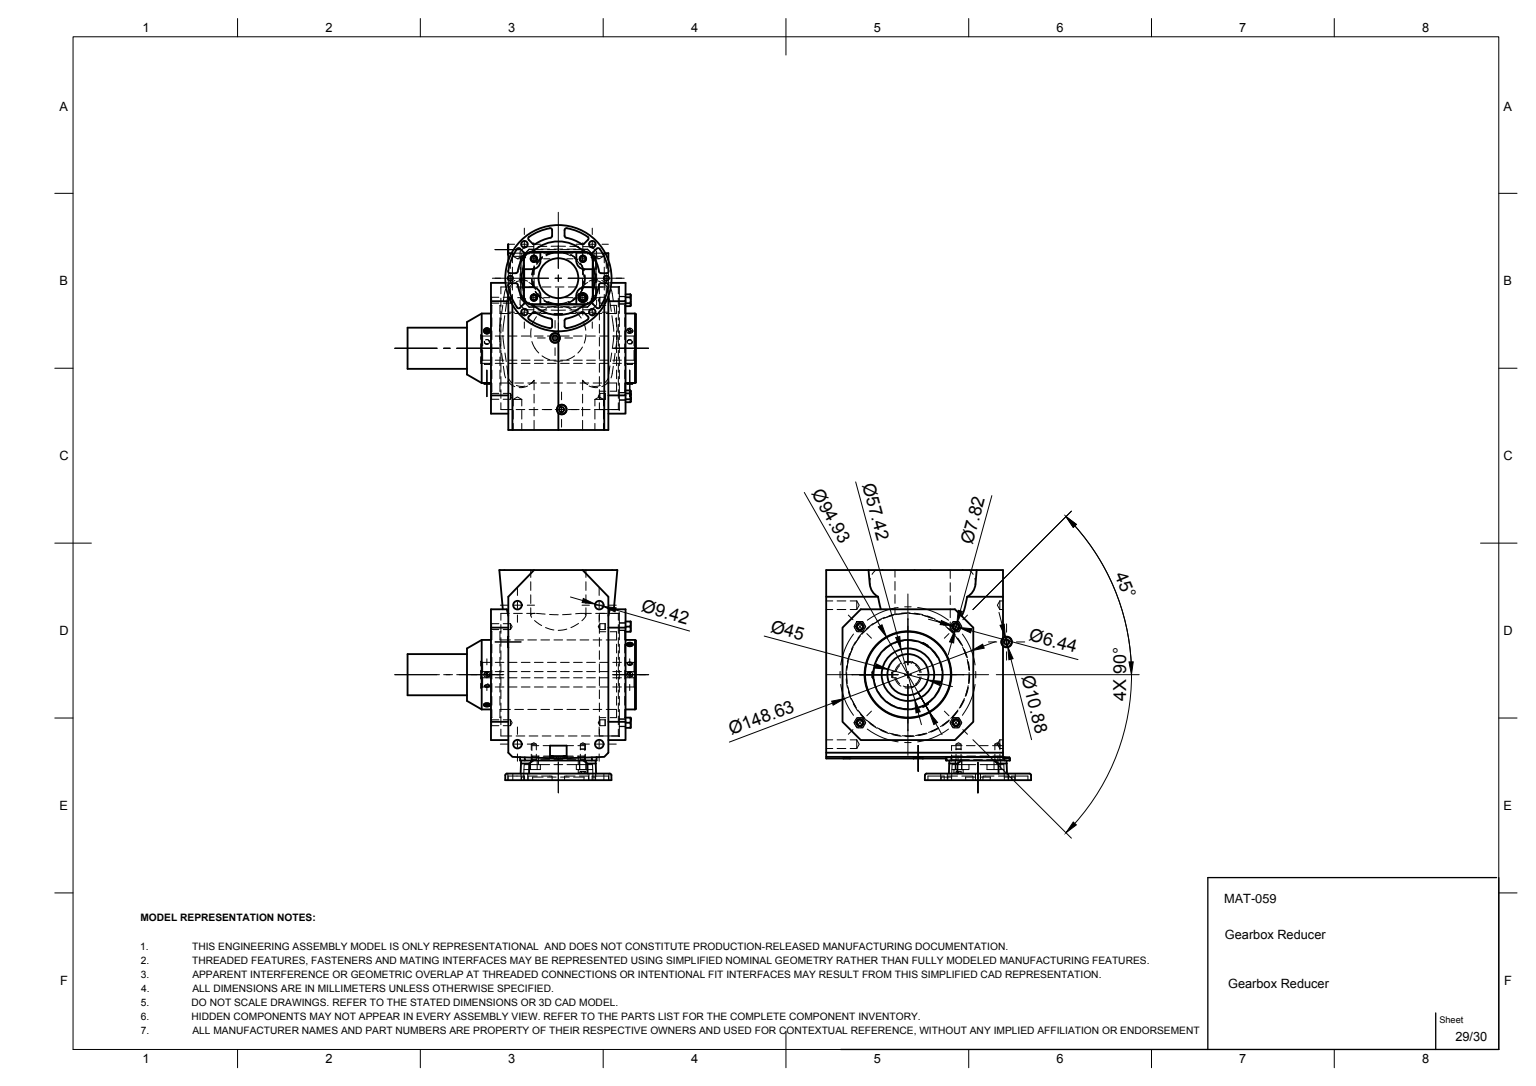
ISO-10303-21;
HEADER;
/* Generated by software containing ST-Developer
 * from STEP Tools, Inc. (www.steptools.com) 
 */

FILE_DESCRIPTION(
/* description */ ('', 'CAx-IF Rec.Pracs.---Representation and Presentation of Product Manufa
cturing Information (PMI)---4.0---2014-10-13'),
/* implementation_level */ '2;1');

FILE_NAME(
/* name */ 'Gearbox Reducer.step',
/* time_stamp */ '2026-10-28T23:00:48+01:00',
/* author */ (''),
/* organization */ (''),
/* preprocessor_version */ 'ST-DEVELOPER v20.2',
/* originating_system */ 'Autodesk Translation Framework v15.17.0.0',
/* authorisation */ '');

FILE_SCHEMA (('AP242_MANAGED_MODEL_BASED_3D_ENGINEERING_MIM_LF { 1 0 10303 442 2 1 4 }'));
ENDSEC;

DATA;
#10=MECHANICAL_DESIGN_GEOMETRIC_PRESENTATION_REPRESENTATION('',(#998),#61811);
#11=ORIENTED_CLOSED_SHELL('',*,#33828,.F.);
#12=ORIENTED_CLOSED_SHELL('',*,#33829,.F.);
#13=ORIENTED_CLOSED_SHELL('',*,#33830,.F.);
#14=ORIENTED_CLOSED_SHELL('',*,#33831,.F.);
#15=ORIENTED_CLOSED_SHELL('',*,#33832,.F.);
#16=ORIENTED_CLOSED_SHELL('',*,#33833,.F.);
#17=ORIENTED_CLOSED_SHELL('',*,#33834,.F.);
#18=ORIENTED_CLOSED_SHELL('',*,#33835,.F.);
#19=ORIENTED_CLOSED_SHELL('',*,#33836,.F.);
#20=ORIENTED_CLOSED_SHELL('',*,#33837,.F.);
#21=BREP_WITH_VOIDS('Body1',#33838,(#11,#12,#13,#14,#15,#16,#17,#18,#19,
#20));
#458=ELLIPSE('',#37359,23.7795204048042,16.4507119775366);
#459=ELLIPSE('',#37368,23.7795204048042,16.4507119775362);
#460=ELLIPSE('',#37370,5.0654611915013,5.05947474242203);
#461=ELLIPSE('',#37371,5.307986116055,5.30171304685244);
#462=ELLIPSE('',#37381,5.06546119150016,5.0594747424216);
#463=ELLIPSE('',#37382,5.30798611605508,5.3017130468524);
#464=ELLIPSE('',#37390,28.8874406483305,28.8698432);
#465=ELLIPSE('',#37391,28.8874406483305,28.8698432);
#466=ELLIPSE('',#37396,28.8695481487031,28.8519616);
#467=ELLIPSE('',#37397,28.8695481487031,28.8519616);
#468=ELLIPSE('',#37482,23.7795204048045,16.4507119775369);
#469=ELLIPSE('',#37484,23.7795204048049,16.4507119775379);
#470=ELLIPSE('',#37887,838.618438479801,28.7580992116283);
#471=ELLIPSE('',#37889,839.102181389802,28.77690685743);
#472=ELLIPSE('',#37898,838.752454381848,28.7633083459289);
#473=ELLIPSE('',#37900,838.930999847209,28.7702505633731);
#511=(
BOUNDED_CURVE()
B_SPLINE_CURVE(2,(#58779,#58780,#58781),.UNSPECIFIED.,.F.,.F.)
B_SPLINE_CURVE_WITH_KNOTS((3,3),(-1.96119676425552,-0.523147579176476),
 .UNSPECIFIED.)
CURVE()
GEOMETRIC_REPRESENTATION_ITEM()
RATIONAL_B_SPLINE_CURVE((1.06676786887492,1.04969648457804,1.02176211535249))
REPRESENTATION_ITEM('')
);
#512=(
BOUNDED_CURVE()
B_SPLINE_CURVE(2,(#58801,#58802,#58803),.UNSPECIFIED.,.F.,.F.)
B_SPLINE_CURVE_WITH_KNOTS((3,3),(-7.9190884120588,-5.23007186679282),
 .UNSPECIFIED.)
CURVE()
GEOMETRIC_REPRESENTATION_ITEM()
RATIONAL_B_SPLINE_CURVE((1.02176211535249,1.07399675503552,1.08824844879795))
REPRESENTATION_ITEM('')
);
#513=(
BOUNDED_CURVE()
B_SPLINE_CURVE(2,(#58988,#58989,#58990),.UNSPECIFIED.,.F.,.F.)
B_SPLINE_CURVE_WITH_KNOTS((3,3),(5.23007186679282,7.9190884120588),
 .UNSPECIFIED.)
CURVE()
GEOMETRIC_REPRESENTATION_ITEM()
RATIONAL_B_SPLINE_CURVE((1.08824844879795,1.07399675503552,1.02176211535249))
REPRESENTATION_ITEM('')
);
#514=(
BOUNDED_CURVE()
B_SPLINE_CURVE(2,(#59004,#59005,#59006),.UNSPECIFIED.,.F.,.F.)
B_SPLINE_CURVE_WITH_KNOTS((3,3),(0.523147579176475,1.96119676425551),
 .UNSPECIFIED.)
CURVE()
GEOMETRIC_REPRESENTATION_ITEM()
RATIONAL_B_SPLINE_CURVE((1.02176211535249,1.04969648457805,1.06676786887492))
REPRESENTATION_ITEM('')
);
#515=(
BOUNDED_CURVE()
B_SPLINE_CURVE(2,(#59072,#59073,#59074),.UNSPECIFIED.,.F.,.F.)
B_SPLINE_CURVE_WITH_KNOTS((3,3),(0.,0.357592968100342),.UNSPECIFIED.)
CURVE()
GEOMETRIC_REPRESENTATION_ITEM()
RATIONAL_B_SPLINE_CURVE((1.,1.00186100329507,1.))
REPRESENTATION_ITEM('')
);
#516=(
BOUNDED_CURVE()
B_SPLINE_CURVE(2,(#59077,#59078,#59079),.UNSPECIFIED.,.F.,.F.)
B_SPLINE_CURVE_WITH_KNOTS((3,3),(0.,0.357592968100342),.UNSPECIFIED.)
CURVE()
GEOMETRIC_REPRESENTATION_ITEM()
RATIONAL_B_SPLINE_CURVE((1.,1.00186100329509,1.))
REPRESENTATION_ITEM('')
);
#517=(
BOUNDED_CURVE()
B_SPLINE_CURVE(2,(#59162,#59163,#59164),.UNSPECIFIED.,.F.,.F.)
B_SPLINE_CURVE_WITH_KNOTS((3,3),(1.4922333840247,2.15631214646323),
 .UNSPECIFIED.)
CURVE()
GEOMETRIC_REPRESENTATION_ITEM()
RATIONAL_B_SPLINE_CURVE((1.8473383335981,1.95114786800464,1.97954092996664))
REPRESENTATION_ITEM('')
);
#518=(
BOUNDED_CURVE()
B_SPLINE_CURVE(2,(#59168,#59169,#59170),.UNSPECIFIED.,.F.,.F.)
B_SPLINE_CURVE_WITH_KNOTS((3,3),(2.65634161849746,3.32042038093599),
 .UNSPECIFIED.)
CURVE()
GEOMETRIC_REPRESENTATION_ITEM()
RATIONAL_B_SPLINE_CURVE((1.97954092996664,1.95114786800464,1.8473383335981))
REPRESENTATION_ITEM('')
);
#519=(
BOUNDED_CURVE()
B_SPLINE_CURVE(2,(#59179,#59180,#59181),.UNSPECIFIED.,.F.,.F.)
B_SPLINE_CURVE_WITH_KNOTS((3,3),(1.4922333840247,2.15631214646323),
 .UNSPECIFIED.)
CURVE()
GEOMETRIC_REPRESENTATION_ITEM()
RATIONAL_B_SPLINE_CURVE((1.8473383335981,1.95114786800464,1.97954092996664))
REPRESENTATION_ITEM('')
);
#520=(
BOUNDED_CURVE()
B_SPLINE_CURVE(2,(#59184,#59185,#59186),.UNSPECIFIED.,.F.,.F.)
B_SPLINE_CURVE_WITH_KNOTS((3,3),(2.65634161849746,3.32042038093599),
 .UNSPECIFIED.)
CURVE()
GEOMETRIC_REPRESENTATION_ITEM()
RATIONAL_B_SPLINE_CURVE((1.97954092996664,1.95114786800464,1.8473383335981))
REPRESENTATION_ITEM('')
);
#521=(
BOUNDED_CURVE()
B_SPLINE_CURVE(2,(#59193,#59194,#59195),.UNSPECIFIED.,.F.,.F.)
B_SPLINE_CURVE_WITH_KNOTS((3,3),(1.4922333840247,2.15631214646323),
 .UNSPECIFIED.)
CURVE()
GEOMETRIC_REPRESENTATION_ITEM()
RATIONAL_B_SPLINE_CURVE((1.8473383335981,1.95114786800464,1.97954092996664))
REPRESENTATION_ITEM('')
);
#522=(
BOUNDED_CURVE()
B_SPLINE_CURVE(2,(#59198,#59199,#59200),.UNSPECIFIED.,.F.,.F.)
B_SPLINE_CURVE_WITH_KNOTS((3,3),(2.65634161849746,3.32042038093599),
 .UNSPECIFIED.)
CURVE()
GEOMETRIC_REPRESENTATION_ITEM()
RATIONAL_B_SPLINE_CURVE((1.97954092996664,1.95114786800464,1.8473383335981))
REPRESENTATION_ITEM('')
);
#523=(
BOUNDED_CURVE()
B_SPLINE_CURVE(2,(#59207,#59208,#59209),.UNSPECIFIED.,.F.,.F.)
B_SPLINE_CURVE_WITH_KNOTS((3,3),(1.4922333840247,2.15631214646323),
 .UNSPECIFIED.)
CURVE()
GEOMETRIC_REPRESENTATION_ITEM()
RATIONAL_B_SPLINE_CURVE((1.8473383335981,1.95114786800464,1.97954092996664))
REPRESENTATION_ITEM('')
);
#524=(
BOUNDED_CURVE()
B_SPLINE_CURVE(2,(#59212,#59213,#59214),.UNSPECIFIED.,.F.,.F.)
B_SPLINE_CURVE_WITH_KNOTS((3,3),(2.65634161849746,3.32042038093599),
 .UNSPECIFIED.)
CURVE()
GEOMETRIC_REPRESENTATION_ITEM()
RATIONAL_B_SPLINE_CURVE((1.97954092996664,1.95114786800464,1.8473383335981))
REPRESENTATION_ITEM('')
);
#525=(
BOUNDED_CURVE()
B_SPLINE_CURVE(2,(#59220,#59221,#59222),.UNSPECIFIED.,.F.,.F.)
B_SPLINE_CURVE_WITH_KNOTS((3,3),(-2.15631214646323,-1.4922333840247),
 .UNSPECIFIED.)
CURVE()
GEOMETRIC_REPRESENTATION_ITEM()
RATIONAL_B_SPLINE_CURVE((1.97954092996664,1.95114786800464,1.8473383335981))
REPRESENTATION_ITEM('')
);
#526=(
BOUNDED_CURVE()
B_SPLINE_CURVE(2,(#59229,#59230,#59231),.UNSPECIFIED.,.F.,.F.)
B_SPLINE_CURVE_WITH_KNOTS((3,3),(-3.32042038093599,-2.65634161849746),
 .UNSPECIFIED.)
CURVE()
GEOMETRIC_REPRESENTATION_ITEM()
RATIONAL_B_SPLINE_CURVE((1.8473383335981,1.95114786800464,1.97954092996664))
REPRESENTATION_ITEM('')
);
#527=(
BOUNDED_CURVE()
B_SPLINE_CURVE(2,(#59233,#59234,#59235),.UNSPECIFIED.,.F.,.F.)
B_SPLINE_CURVE_WITH_KNOTS((3,3),(-2.15631214646323,-1.4922333840247),
 .UNSPECIFIED.)
CURVE()
GEOMETRIC_REPRESENTATION_ITEM()
RATIONAL_B_SPLINE_CURVE((1.97954092996664,1.95114786800464,1.8473383335981))
REPRESENTATION_ITEM('')
);
#528=(
BOUNDED_CURVE()
B_SPLINE_CURVE(2,(#59239,#59240,#59241),.UNSPECIFIED.,.F.,.F.)
B_SPLINE_CURVE_WITH_KNOTS((3,3),(-3.32042038093599,-2.65634161849746),
 .UNSPECIFIED.)
CURVE()
GEOMETRIC_REPRESENTATION_ITEM()
RATIONAL_B_SPLINE_CURVE((1.8473383335981,1.95114786800464,1.97954092996664))
REPRESENTATION_ITEM('')
);
#529=(
BOUNDED_CURVE()
B_SPLINE_CURVE(2,(#59259,#59260,#59261),.UNSPECIFIED.,.F.,.F.)
B_SPLINE_CURVE_WITH_KNOTS((3,3),(1.4922333840247,2.15631214646323),
 .UNSPECIFIED.)
CURVE()
GEOMETRIC_REPRESENTATION_ITEM()
RATIONAL_B_SPLINE_CURVE((1.8473383335981,1.95114786800464,1.97954092996664))
REPRESENTATION_ITEM('')
);
#530=(
BOUNDED_CURVE()
B_SPLINE_CURVE(2,(#59265,#59266,#59267),.UNSPECIFIED.,.F.,.F.)
B_SPLINE_CURVE_WITH_KNOTS((3,3),(2.65634161849746,3.32042038093599),
 .UNSPECIFIED.)
CURVE()
GEOMETRIC_REPRESENTATION_ITEM()
RATIONAL_B_SPLINE_CURVE((1.97954092996664,1.95114786800464,1.8473383335981))
REPRESENTATION_ITEM('')
);
#531=(
BOUNDED_CURVE()
B_SPLINE_CURVE(2,(#59276,#59277,#59278),.UNSPECIFIED.,.F.,.F.)
B_SPLINE_CURVE_WITH_KNOTS((3,3),(1.4922333840247,2.15631214646323),
 .UNSPECIFIED.)
CURVE()
GEOMETRIC_REPRESENTATION_ITEM()
RATIONAL_B_SPLINE_CURVE((1.8473383335981,1.95114786800464,1.97954092996664))
REPRESENTATION_ITEM('')
);
#532=(
BOUNDED_CURVE()
B_SPLINE_CURVE(2,(#59281,#59282,#59283),.UNSPECIFIED.,.F.,.F.)
B_SPLINE_CURVE_WITH_KNOTS((3,3),(2.65634161849746,3.32042038093599),
 .UNSPECIFIED.)
CURVE()
GEOMETRIC_REPRESENTATION_ITEM()
RATIONAL_B_SPLINE_CURVE((1.97954092996664,1.95114786800464,1.8473383335981))
REPRESENTATION_ITEM('')
);
#533=(
BOUNDED_CURVE()
B_SPLINE_CURVE(2,(#59290,#59291,#59292),.UNSPECIFIED.,.F.,.F.)
B_SPLINE_CURVE_WITH_KNOTS((3,3),(1.4922333840247,2.15631214646323),
 .UNSPECIFIED.)
CURVE()
GEOMETRIC_REPRESENTATION_ITEM()
RATIONAL_B_SPLINE_CURVE((1.8473383335981,1.95114786800464,1.97954092996664))
REPRESENTATION_ITEM('')
);
#534=(
BOUNDED_CURVE()
B_SPLINE_CURVE(2,(#59295,#59296,#59297),.UNSPECIFIED.,.F.,.F.)
B_SPLINE_CURVE_WITH_KNOTS((3,3),(2.65634161849746,3.32042038093599),
 .UNSPECIFIED.)
CURVE()
GEOMETRIC_REPRESENTATION_ITEM()
RATIONAL_B_SPLINE_CURVE((1.97954092996664,1.95114786800464,1.8473383335981))
REPRESENTATION_ITEM('')
);
#535=(
BOUNDED_CURVE()
B_SPLINE_CURVE(2,(#59304,#59305,#59306),.UNSPECIFIED.,.F.,.F.)
B_SPLINE_CURVE_WITH_KNOTS((3,3),(1.4922333840247,2.15631214646323),
 .UNSPECIFIED.)
CURVE()
GEOMETRIC_REPRESENTATION_ITEM()
RATIONAL_B_SPLINE_CURVE((1.8473383335981,1.95114786800464,1.97954092996664))
REPRESENTATION_ITEM('')
);
#536=(
BOUNDED_CURVE()
B_SPLINE_CURVE(2,(#59309,#59310,#59311),.UNSPECIFIED.,.F.,.F.)
B_SPLINE_CURVE_WITH_KNOTS((3,3),(2.65634161849746,3.32042038093599),
 .UNSPECIFIED.)
CURVE()
GEOMETRIC_REPRESENTATION_ITEM()
RATIONAL_B_SPLINE_CURVE((1.97954092996664,1.95114786800464,1.8473383335981))
REPRESENTATION_ITEM('')
);
#537=(
BOUNDED_CURVE()
B_SPLINE_CURVE(2,(#59317,#59318,#59319),.UNSPECIFIED.,.F.,.F.)
B_SPLINE_CURVE_WITH_KNOTS((3,3),(-2.15631214646323,-1.4922333840247),
 .UNSPECIFIED.)
CURVE()
GEOMETRIC_REPRESENTATION_ITEM()
RATIONAL_B_SPLINE_CURVE((1.97954092996664,1.95114786800464,1.8473383335981))
REPRESENTATION_ITEM('')
);
#538=(
BOUNDED_CURVE()
B_SPLINE_CURVE(2,(#59326,#59327,#59328),.UNSPECIFIED.,.F.,.F.)
B_SPLINE_CURVE_WITH_KNOTS((3,3),(-3.32042038093599,-2.65634161849746),
 .UNSPECIFIED.)
CURVE()
GEOMETRIC_REPRESENTATION_ITEM()
RATIONAL_B_SPLINE_CURVE((1.8473383335981,1.95114786800464,1.97954092996664))
REPRESENTATION_ITEM('')
);
#539=(
BOUNDED_CURVE()
B_SPLINE_CURVE(2,(#59330,#59331,#59332),.UNSPECIFIED.,.F.,.F.)
B_SPLINE_CURVE_WITH_KNOTS((3,3),(-2.15631214646323,-1.4922333840247),
 .UNSPECIFIED.)
CURVE()
GEOMETRIC_REPRESENTATION_ITEM()
RATIONAL_B_SPLINE_CURVE((1.97954092996664,1.95114786800464,1.8473383335981))
REPRESENTATION_ITEM('')
);
#540=(
BOUNDED_CURVE()
B_SPLINE_CURVE(2,(#59336,#59337,#59338),.UNSPECIFIED.,.F.,.F.)
B_SPLINE_CURVE_WITH_KNOTS((3,3),(-3.32042038093599,-2.65634161849746),
 .UNSPECIFIED.)
CURVE()
GEOMETRIC_REPRESENTATION_ITEM()
RATIONAL_B_SPLINE_CURVE((1.8473383335981,1.95114786800464,1.97954092996664))
REPRESENTATION_ITEM('')
);
#541=(
BOUNDED_CURVE()
B_SPLINE_CURVE(2,(#60436,#60437,#60438),.UNSPECIFIED.,.F.,.F.)
B_SPLINE_CURVE_WITH_KNOTS((3,3),(1.4922333840247,2.15631214646323),
 .UNSPECIFIED.)
CURVE()
GEOMETRIC_REPRESENTATION_ITEM()
RATIONAL_B_SPLINE_CURVE((1.8473383335981,1.95114786800464,1.97954092996664))
REPRESENTATION_ITEM('')
);
#542=(
BOUNDED_CURVE()
B_SPLINE_CURVE(2,(#60439,#60440,#60441),.UNSPECIFIED.,.F.,.F.)
B_SPLINE_CURVE_WITH_KNOTS((3,3),(2.65634161849746,3.32042038093599),
 .UNSPECIFIED.)
CURVE()
GEOMETRIC_REPRESENTATION_ITEM()
RATIONAL_B_SPLINE_CURVE((1.97954092996664,1.95114786800464,1.8473383335981))
REPRESENTATION_ITEM('')
);
#543=(
BOUNDED_CURVE()
B_SPLINE_CURVE(2,(#60444,#60445,#60446),.UNSPECIFIED.,.F.,.F.)
B_SPLINE_CURVE_WITH_KNOTS((3,3),(-3.32042038093599,-2.65634161849746),
 .UNSPECIFIED.)
CURVE()
GEOMETRIC_REPRESENTATION_ITEM()
RATIONAL_B_SPLINE_CURVE((1.8473383335981,1.95114786800464,1.97954092996664))
REPRESENTATION_ITEM('')
);
#544=(
BOUNDED_CURVE()
B_SPLINE_CURVE(2,(#60448,#60449,#60450),.UNSPECIFIED.,.F.,.F.)
B_SPLINE_CURVE_WITH_KNOTS((3,3),(-2.15631214646323,-1.4922333840247),
 .UNSPECIFIED.)
CURVE()
GEOMETRIC_REPRESENTATION_ITEM()
RATIONAL_B_SPLINE_CURVE((1.97954092996664,1.95114786800464,1.8473383335981))
REPRESENTATION_ITEM('')
);
#545=(
BOUNDED_CURVE()
B_SPLINE_CURVE(2,(#60455,#60456,#60457),.UNSPECIFIED.,.F.,.F.)
B_SPLINE_CURVE_WITH_KNOTS((3,3),(-3.32042038093599,-2.65634161849746),
 .UNSPECIFIED.)
CURVE()
GEOMETRIC_REPRESENTATION_ITEM()
RATIONAL_B_SPLINE_CURVE((1.8473383335981,1.95114786800464,1.97954092996664))
REPRESENTATION_ITEM('')
);
#546=(
BOUNDED_CURVE()
B_SPLINE_CURVE(2,(#60458,#60459,#60460),.UNSPECIFIED.,.F.,.F.)
B_SPLINE_CURVE_WITH_KNOTS((3,3),(-2.15631214646323,-1.4922333840247),
 .UNSPECIFIED.)
CURVE()
GEOMETRIC_REPRESENTATION_ITEM()
RATIONAL_B_SPLINE_CURVE((1.97954092996664,1.95114786800464,1.8473383335981))
REPRESENTATION_ITEM('')
);
#547=(
BOUNDED_CURVE()
B_SPLINE_CURVE(2,(#60464,#60465,#60466),.UNSPECIFIED.,.F.,.F.)
B_SPLINE_CURVE_WITH_KNOTS((3,3),(2.65634161849746,3.32042038093599),
 .UNSPECIFIED.)
CURVE()
GEOMETRIC_REPRESENTATION_ITEM()
RATIONAL_B_SPLINE_CURVE((1.97954092996664,1.95114786800464,1.8473383335981))
REPRESENTATION_ITEM('')
);
#548=(
BOUNDED_CURVE()
B_SPLINE_CURVE(2,(#60467,#60468,#60469),.UNSPECIFIED.,.F.,.F.)
B_SPLINE_CURVE_WITH_KNOTS((3,3),(1.4922333840247,2.15631214646323),
 .UNSPECIFIED.)
CURVE()
GEOMETRIC_REPRESENTATION_ITEM()
RATIONAL_B_SPLINE_CURVE((1.8473383335981,1.95114786800464,1.97954092996664))
REPRESENTATION_ITEM('')
);
#549=(
BOUNDED_CURVE()
B_SPLINE_CURVE(2,(#60471,#60472,#60473),.UNSPECIFIED.,.F.,.F.)
B_SPLINE_CURVE_WITH_KNOTS((3,3),(2.65634161849746,3.32042038093599),
 .UNSPECIFIED.)
CURVE()
GEOMETRIC_REPRESENTATION_ITEM()
RATIONAL_B_SPLINE_CURVE((1.97954092996664,1.95114786800464,1.8473383335981))
REPRESENTATION_ITEM('')
);
#550=(
BOUNDED_CURVE()
B_SPLINE_CURVE(2,(#60477,#60478,#60479),.UNSPECIFIED.,.F.,.F.)
B_SPLINE_CURVE_WITH_KNOTS((3,3),(2.65634161849746,3.32042038093599),
 .UNSPECIFIED.)
CURVE()
GEOMETRIC_REPRESENTATION_ITEM()
RATIONAL_B_SPLINE_CURVE((1.97954092996664,1.95114786800464,1.8473383335981))
REPRESENTATION_ITEM('')
);
#551=(
BOUNDED_CURVE()
B_SPLINE_CURVE(2,(#60480,#60481,#60482),.UNSPECIFIED.,.F.,.F.)
B_SPLINE_CURVE_WITH_KNOTS((3,3),(1.4922333840247,2.15631214646323),
 .UNSPECIFIED.)
CURVE()
GEOMETRIC_REPRESENTATION_ITEM()
RATIONAL_B_SPLINE_CURVE((1.8473383335981,1.95114786800464,1.97954092996664))
REPRESENTATION_ITEM('')
);
#552=(
BOUNDED_CURVE()
B_SPLINE_CURVE(2,(#60484,#60485,#60486),.UNSPECIFIED.,.F.,.F.)
B_SPLINE_CURVE_WITH_KNOTS((3,3),(1.4922333840247,2.15631214646323),
 .UNSPECIFIED.)
CURVE()
GEOMETRIC_REPRESENTATION_ITEM()
RATIONAL_B_SPLINE_CURVE((1.8473383335981,1.95114786800464,1.97954092996664))
REPRESENTATION_ITEM('')
);
#553=(
BOUNDED_CURVE()
B_SPLINE_CURVE(2,(#60521,#60522,#60523),.UNSPECIFIED.,.F.,.F.)
B_SPLINE_CURVE_WITH_KNOTS((3,3),(1.4922333840247,2.15631214646323),
 .UNSPECIFIED.)
CURVE()
GEOMETRIC_REPRESENTATION_ITEM()
RATIONAL_B_SPLINE_CURVE((1.8473383335981,1.95114786800464,1.97954092996664))
REPRESENTATION_ITEM('')
);
#554=(
BOUNDED_CURVE()
B_SPLINE_CURVE(2,(#60524,#60525,#60526),.UNSPECIFIED.,.F.,.F.)
B_SPLINE_CURVE_WITH_KNOTS((3,3),(2.65634161849746,3.32042038093599),
 .UNSPECIFIED.)
CURVE()
GEOMETRIC_REPRESENTATION_ITEM()
RATIONAL_B_SPLINE_CURVE((1.97954092996664,1.95114786800464,1.8473383335981))
REPRESENTATION_ITEM('')
);
#555=(
BOUNDED_CURVE()
B_SPLINE_CURVE(2,(#60529,#60530,#60531),.UNSPECIFIED.,.F.,.F.)
B_SPLINE_CURVE_WITH_KNOTS((3,3),(-3.32042038093599,-2.65634161849746),
 .UNSPECIFIED.)
CURVE()
GEOMETRIC_REPRESENTATION_ITEM()
RATIONAL_B_SPLINE_CURVE((1.8473383335981,1.95114786800464,1.97954092996664))
REPRESENTATION_ITEM('')
);
#556=(
BOUNDED_CURVE()
B_SPLINE_CURVE(2,(#60533,#60534,#60535),.UNSPECIFIED.,.F.,.F.)
B_SPLINE_CURVE_WITH_KNOTS((3,3),(-2.15631214646323,-1.4922333840247),
 .UNSPECIFIED.)
CURVE()
GEOMETRIC_REPRESENTATION_ITEM()
RATIONAL_B_SPLINE_CURVE((1.97954092996664,1.95114786800464,1.8473383335981))
REPRESENTATION_ITEM('')
);
#557=(
BOUNDED_CURVE()
B_SPLINE_CURVE(2,(#60540,#60541,#60542),.UNSPECIFIED.,.F.,.F.)
B_SPLINE_CURVE_WITH_KNOTS((3,3),(-3.32042038093599,-2.65634161849746),
 .UNSPECIFIED.)
CURVE()
GEOMETRIC_REPRESENTATION_ITEM()
RATIONAL_B_SPLINE_CURVE((1.8473383335981,1.95114786800464,1.97954092996664))
REPRESENTATION_ITEM('')
);
#558=(
BOUNDED_CURVE()
B_SPLINE_CURVE(2,(#60543,#60544,#60545),.UNSPECIFIED.,.F.,.F.)
B_SPLINE_CURVE_WITH_KNOTS((3,3),(-2.15631214646323,-1.4922333840247),
 .UNSPECIFIED.)
CURVE()
GEOMETRIC_REPRESENTATION_ITEM()
RATIONAL_B_SPLINE_CURVE((1.97954092996664,1.95114786800464,1.8473383335981))
REPRESENTATION_ITEM('')
);
#559=(
BOUNDED_CURVE()
B_SPLINE_CURVE(2,(#60549,#60550,#60551),.UNSPECIFIED.,.F.,.F.)
B_SPLINE_CURVE_WITH_KNOTS((3,3),(2.65634161849746,3.32042038093599),
 .UNSPECIFIED.)
CURVE()
GEOMETRIC_REPRESENTATION_ITEM()
RATIONAL_B_SPLINE_CURVE((1.97954092996664,1.95114786800464,1.8473383335981))
REPRESENTATION_ITEM('')
);
#560=(
BOUNDED_CURVE()
B_SPLINE_CURVE(2,(#60552,#60553,#60554),.UNSPECIFIED.,.F.,.F.)
B_SPLINE_CURVE_WITH_KNOTS((3,3),(1.4922333840247,2.15631214646323),
 .UNSPECIFIED.)
CURVE()
GEOMETRIC_REPRESENTATION_ITEM()
RATIONAL_B_SPLINE_CURVE((1.8473383335981,1.95114786800464,1.97954092996664))
REPRESENTATION_ITEM('')
);
#561=(
BOUNDED_CURVE()
B_SPLINE_CURVE(2,(#60556,#60557,#60558),.UNSPECIFIED.,.F.,.F.)
B_SPLINE_CURVE_WITH_KNOTS((3,3),(2.65634161849746,3.32042038093599),
 .UNSPECIFIED.)
CURVE()
GEOMETRIC_REPRESENTATION_ITEM()
RATIONAL_B_SPLINE_CURVE((1.97954092996664,1.95114786800464,1.8473383335981))
REPRESENTATION_ITEM('')
);
#562=(
BOUNDED_CURVE()
B_SPLINE_CURVE(2,(#60562,#60563,#60564),.UNSPECIFIED.,.F.,.F.)
B_SPLINE_CURVE_WITH_KNOTS((3,3),(2.65634161849746,3.32042038093599),
 .UNSPECIFIED.)
CURVE()
GEOMETRIC_REPRESENTATION_ITEM()
RATIONAL_B_SPLINE_CURVE((1.97954092996664,1.95114786800464,1.8473383335981))
REPRESENTATION_ITEM('')
);
#563=(
BOUNDED_CURVE()
B_SPLINE_CURVE(2,(#60565,#60566,#60567),.UNSPECIFIED.,.F.,.F.)
B_SPLINE_CURVE_WITH_KNOTS((3,3),(1.4922333840247,2.15631214646323),
 .UNSPECIFIED.)
CURVE()
GEOMETRIC_REPRESENTATION_ITEM()
RATIONAL_B_SPLINE_CURVE((1.8473383335981,1.95114786800464,1.97954092996664))
REPRESENTATION_ITEM('')
);
#564=(
BOUNDED_CURVE()
B_SPLINE_CURVE(2,(#60569,#60570,#60571),.UNSPECIFIED.,.F.,.F.)
B_SPLINE_CURVE_WITH_KNOTS((3,3),(1.4922333840247,2.15631214646323),
 .UNSPECIFIED.)
CURVE()
GEOMETRIC_REPRESENTATION_ITEM()
RATIONAL_B_SPLINE_CURVE((1.8473383335981,1.95114786800464,1.97954092996664))
REPRESENTATION_ITEM('')
);
#616=CONICAL_SURFACE('',#37248,3.21359174399996,0.785398163397452);
#617=CONICAL_SURFACE('',#37253,0.322047616000012,1.0471975511966);
#618=CONICAL_SURFACE('',#37265,3.21359174400012,0.785398163397384);
#619=CONICAL_SURFACE('',#37270,0.322047616,1.04719755119659);
#620=CONICAL_SURFACE('',#37282,2.74142809600001,0.785398163397436);
#621=CONICAL_SURFACE('',#37290,0.274750783999988,1.04719755119659);
#622=CONICAL_SURFACE('',#37307,3.21359174400008,0.785398163397464);
#623=CONICAL_SURFACE('',#37315,0.322047616,1.04719755119659);
#624=CONICAL_SURFACE('',#37324,3.21359174399998,0.785398163397522);
#625=CONICAL_SURFACE('',#37332,0.322047616000012,1.04719755119659);
#626=CONICAL_SURFACE('',#37334,62.4381557149574,0.0364929375524579);
#627=CONICAL_SURFACE('',#37338,62.4381557149626,0.0364929375527776);
#628=CONICAL_SURFACE('',#37404,28.7625535999985,0.785398163397467);
#629=CONICAL_SURFACE('',#37440,6.37205498762855,1.04719755119635);
#630=CONICAL_SURFACE('',#37442,6.37205498762726,1.04719755119649);
#631=CONICAL_SURFACE('',#37444,6.37205498762869,1.04719755119634);
#632=CONICAL_SURFACE('',#37446,6.37205498762701,1.04719755119652);
#633=CONICAL_SURFACE('',#37448,6.37205498762724,1.04719755119655);
#634=CONICAL_SURFACE('',#37452,6.37205498762882,1.04719755119634);
#635=CONICAL_SURFACE('',#37459,6.37205498762342,1.04719755119681);
#636=CONICAL_SURFACE('',#37461,6.37205498762507,1.04719755119686);
#637=CONICAL_SURFACE('',#37463,6.37205498763146,1.04719755119606);
#638=CONICAL_SURFACE('',#37465,6.37205498762404,1.04719755119683);
#639=CONICAL_SURFACE('',#37467,6.37205498762824,1.04719755119636);
#640=CONICAL_SURFACE('',#37471,6.37205498763465,1.04719755119586);
#641=CONICAL_SURFACE('',#37485,17.3000533734216,0.0872664625997182);
#642=CONICAL_SURFACE('',#37486,5.46753820577589,0.769793460898297);
#643=CONICAL_SURFACE('',#37488,5.24100524633615,0.769793460899118);
#644=CONICAL_SURFACE('',#37497,5.24100524634338,0.769793460898339);
#645=CONICAL_SURFACE('',#37507,5.46753820577565,0.769793460898311);
#646=CONICAL_SURFACE('',#37515,5.83240278777977,0.769793460898674);
#647=CONICAL_SURFACE('',#37516,0.274750783999998,1.04719755119659);
#648=CONICAL_SURFACE('',#37522,2.80803705600002,0.785398163397436);
#649=CONICAL_SURFACE('',#37524,0.274750783999993,1.04719755119659);
#650=CONICAL_SURFACE('',#37530,2.808037056,0.785398163397464);
#651=CONICAL_SURFACE('',#37532,0.274750783999995,1.04719755119659);
#652=CONICAL_SURFACE('',#37538,2.80803705600003,0.785398163397438);
#653=CONICAL_SURFACE('',#37540,3.28958854399998,0.78539816339744);
#654=CONICAL_SURFACE('',#37547,0.322047616000123,1.04719755119657);
#655=CONICAL_SURFACE('',#37548,3.2895885439999,0.785398163397438);
#656=CONICAL_SURFACE('',#37555,0.322047615999997,1.04719755119659);
#657=CONICAL_SURFACE('',#37556,3.289588544,0.78539816339742);
#658=CONICAL_SURFACE('',#37563,0.322047616000094,1.04719755119659);
#659=CONICAL_SURFACE('',#37564,3.2895885439999,0.78539816339744);
#660=CONICAL_SURFACE('',#37571,0.32204761600005,1.04719755119655);
#661=CONICAL_SURFACE('',#37572,0.470822528000023,1.04719755119659);
#662=CONICAL_SURFACE('',#37573,0.470822528000024,1.04719755119659);
#663=CONICAL_SURFACE('',#37574,0.470822528000001,1.04719755119667);
#664=CONICAL_SURFACE('',#37575,0.470822528000002,1.04719755119667);
#665=CONICAL_SURFACE('',#37576,0.47082252800002,1.04719755119667);
#666=CONICAL_SURFACE('',#37577,0.470822528000018,1.04719755119667);
#667=CONICAL_SURFACE('',#37578,0.470822528000013,1.04719755119659);
#668=CONICAL_SURFACE('',#37579,0.470822528000016,1.04719755119659);
#669=CONICAL_SURFACE('',#37594,46.9997605328678,0.523598775598269);
#670=CONICAL_SURFACE('',#37609,17.3000533734219,0.0872664625997327);
#671=CONICAL_SURFACE('',#37610,67.117943679437,0.523598775598465);
#672=CONICAL_SURFACE('',#37615,28.921462932868,0.52359877559825);
#673=CONICAL_SURFACE('',#37618,17.3539050991947,0.0872664625997172);
#674=CONICAL_SURFACE('',#37619,17.3539050991947,0.0872664625997133);
#675=CONICAL_SURFACE('',#37623,46.9997605328686,0.523598775598271);
#676=CONICAL_SURFACE('',#37637,37.927515520559,0.523598775598339);
#677=CONICAL_SURFACE('',#37643,13.5507337588825,0.523598775598299);
#678=CONICAL_SURFACE('',#37670,3.2861910399999,0.785398163397455);
#679=CONICAL_SURFACE('',#37674,2.74142809599801,0.78539816339774);
#680=CONICAL_SURFACE('',#37681,3.28619103999997,0.78539816339744);
#681=CONICAL_SURFACE('',#37700,3.28619104000002,0.785398163397459);
#682=CONICAL_SURFACE('',#37704,2.74142809600037,0.785398163397935);
#683=CONICAL_SURFACE('',#37711,3.28619104000001,0.785398163397442);
#684=CONICAL_SURFACE('',#37715,2.74142809599998,0.78539816339744);
#685=CONICAL_SURFACE('',#37722,2.74142809599988,0.785398163397487);
#686=CONICAL_SURFACE('',#37728,37.0614901167744,0.523598775598295);
#687=CONICAL_SURFACE('',#37730,13.5507337588825,0.523598775598308);
#688=CONICAL_SURFACE('',#37752,6.37205498763392,1.04719755119592);
#689=CONICAL_SURFACE('',#37755,6.37205498762829,1.04719755119636);
#690=CONICAL_SURFACE('',#37756,6.37205498762407,1.04719755119683);
#691=CONICAL_SURFACE('',#37757,6.3720549876336,1.04719755119585);
#692=CONICAL_SURFACE('',#37758,6.3720549876249,1.04719755119687);
#693=CONICAL_SURFACE('',#37759,6.37205498762508,1.04719755119666);
#694=CONICAL_SURFACE('',#37771,6.37205498762851,1.04719755119636);
#695=CONICAL_SURFACE('',#37774,6.372054987629,1.04719755119631);
#696=CONICAL_SURFACE('',#37775,6.37205498762379,1.04719755119685);
#697=CONICAL_SURFACE('',#37776,6.37205498762845,1.04719755119638);
#698=CONICAL_SURFACE('',#37777,6.37205498762874,1.04719755119636);
#699=CONICAL_SURFACE('',#37778,6.37205498762885,1.04719755119632);
#700=CONICAL_SURFACE('',#37913,58.1057817920919,0.0174532925199245);
#701=CONICAL_SURFACE('',#37922,8.57550304943042,0.0349065850398547);
#702=CONICAL_SURFACE('',#37925,8.57550304942994,0.0349065850398894);
#703=CONICAL_SURFACE('',#37928,8.57550304942982,0.0349065850398904);
#704=CONICAL_SURFACE('',#37934,8.57550304942991,0.034906585039891);
#705=CONICAL_SURFACE('',#38071,4.98002560000028,0.785398163397452);
#706=CONICAL_SURFACE('',#38078,5.01355360000019,0.785398163397488);
#831=B_SPLINE_CURVE_WITH_KNOTS('',3,(#59743,#59744,#59745,#59746,#59747,
#59748,#59749,#59750),.UNSPECIFIED.,.F.,.F.,(4,2,2,4),(-6.50854151614474,
-6.00862181551197,-5.43826767053468,-4.86791352555738),.UNSPECIFIED.);
#832=B_SPLINE_CURVE_WITH_KNOTS('',3,(#59752,#59753,#59754,#59755,#59756,
#59757,#59758,#59759,#59760,#59761,#59762,#59763,#59764,#59765,#59766,#59767,
#59768,#59769,#59770,#59771,#59772,#59773,#59774,#59775,#59776,#59777),
 .UNSPECIFIED.,.F.,.F.,(4,2,2,2,2,2,2,2,2,2,2,2,4),(6.50854151613977,6.57897596048927,
7.14933010546656,7.72311029238147,8.29689047929639,8.8706706662113,9.44445085312622,
10.0182310400411,10.592011226956,11.165791413871,11.7395716007859,12.3099257457632,
12.3803601901077),.UNSPECIFIED.);
#833=B_SPLINE_CURVE_WITH_KNOTS('',3,(#59778,#59779,#59780,#59781,#59782,
#59783,#59784,#59785,#59786,#59787,#59788,#59789,#59790,#59791,#59792,#59793,
#59794,#59795,#59796,#59797,#59798,#59799,#59800,#59801,#59802,#59803,#59804,
#59805,#59806,#59807,#59808,#59809,#59810,#59811,#59812,#59813,#59814,#59815,
#59816,#59817,#59818),.UNSPECIFIED.,.F.,.F.,(4,2,2,2,2,2,2,2,3,2,2,2,2,
2,2,2,2,2,2,4),(-4.86791352555738,-4.23909906011465,-3.61028459467191,-2.98147012922918,
-2.35265566378644,-1.76449174783983,-1.17632783189322,-0.588163915946611,
0.,0.588163915946613,1.17632783189323,1.76449174783983,2.35265566378645,
2.98147012922918,3.61028459467192,4.23909906011465,4.86791352555738,5.43826767053468,
6.00862181551197,6.50854151613977),.UNSPECIFIED.);
#834=B_SPLINE_CURVE_WITH_KNOTS('',3,(#59904,#59905,#59906,#59907),
 .UNSPECIFIED.,.F.,.F.,(4,4),(0.0184096978210032,0.021955582065653),
 .UNSPECIFIED.);
#835=B_SPLINE_CURVE_WITH_KNOTS('',3,(#59908,#59909,#59910,#59911),
 .UNSPECIFIED.,.F.,.F.,(4,4),(0.0186156132125293,0.0221618161533776),
 .UNSPECIFIED.);
#836=B_SPLINE_CURVE_WITH_KNOTS('',3,(#59922,#59923,#59924,#59925,#59926,
#59927,#59928,#59929,#59930,#59931,#59932,#59933,#59934,#59935,#59936,#59937,
#59938,#59939,#59940,#59941,#59942,#59943,#59944,#59945,#59946,#59947,#59948,
#59949,#59950,#59951,#59952,#59953,#59954,#59955),.UNSPECIFIED.,.T.,.F.,
(4,2,2,2,2,2,2,2,2,2,2,2,2,2,2,2,4),(0.,0.103814244533191,0.207628489066383,
0.311436347509041,0.415244205951698,0.519052064394355,0.622859922837012,
0.726674167370203,0.830488411903395,0.934302656436586,1.03811690096978,
1.14192475941243,1.24573261785509,1.34954047629775,1.45334833474041,1.5571625792736,
1.66097682380679),.UNSPECIFIED.);
#837=B_SPLINE_CURVE_WITH_KNOTS('',3,(#59957,#59958,#59959,#59960,#59961,
#59962,#59963,#59964,#59965,#59966,#59967,#59968,#59969,#59970,#59971,#59972,
#59973,#59974,#59975,#59976,#59977,#59978,#59979,#59980,#59981,#59982,#59983,
#59984,#59985,#59986,#59987,#59988,#59989,#59990),.UNSPECIFIED.,.T.,.F.,
(4,2,2,2,2,2,2,2,2,2,2,2,2,2,2,2,4),(0.,0.103814244533193,0.207628489066386,
0.311436347509045,0.415244205951704,0.519052064394364,0.622859922837024,
0.726674167370216,0.830488411903409,0.934302656436602,1.0381169009698,1.14192475941245,
1.24573261785511,1.34954047629777,1.45334833474043,1.55716257927362,1.66097682380682),
 .UNSPECIFIED.);
#838=B_SPLINE_CURVE_WITH_KNOTS('',3,(#60087,#60088,#60089,#60090,#60091,
#60092,#60093,#60094,#60095,#60096,#60097,#60098,#60099,#60100,#60101,#60102,
#60103,#60104,#60105,#60106,#60107,#60108,#60109,#60110,#60111,#60112,#60113,
#60114,#60115,#60116,#60117,#60118,#60119,#60120),.UNSPECIFIED.,.T.,.F.,
(4,2,2,2,2,2,2,2,2,2,2,2,2,2,2,2,4),(0.,0.126366208363918,0.252732416727836,
0.37909836467664,0.505464312625444,0.631830260574249,0.758196208523054,
0.884562416886971,1.01092862525089,1.13729483361481,1.26366104197873,1.39002698992753,
1.51639293787633,1.64275888582514,1.76912483377394,1.89549104213786,2.02185725050178),
 .UNSPECIFIED.);
#839=B_SPLINE_CURVE_WITH_KNOTS('',3,(#60225,#60226,#60227,#60228,#60229,
#60230,#60231,#60232,#60233,#60234,#60235,#60236,#60237,#60238,#60239,#60240,
#60241,#60242,#60243,#60244,#60245,#60246,#60247,#60248,#60249,#60250,#60251,
#60252,#60253,#60254,#60255,#60256,#60257,#60258),.UNSPECIFIED.,.T.,.F.,
(4,2,2,2,2,2,2,2,2,2,2,2,2,2,2,2,4),(0.,0.126366208363919,0.252732416727838,
0.379098364676642,0.505464312625446,0.631830260574251,0.758196208523055,
0.884562416886973,1.01092862525089,1.13729483361481,1.26366104197873,1.39002698992753,
1.51639293787634,1.64275888582514,1.76912483377395,1.89549104213787,2.02185725050179),
 .UNSPECIFIED.);
#840=B_SPLINE_CURVE_WITH_KNOTS('',3,(#60280,#60281,#60282,#60283,#60284,
#60285,#60286,#60287,#60288,#60289,#60290,#60291,#60292,#60293,#60294,#60295,
#60296,#60297,#60298,#60299,#60300,#60301,#60302,#60303,#60304,#60305,#60306,
#60307,#60308,#60309,#60310,#60311,#60312,#60313),.UNSPECIFIED.,.T.,.F.,
(4,2,2,2,2,2,2,2,2,2,2,2,2,2,2,2,4),(0.,0.126366208363919,0.252732416727837,
0.379098364676641,0.505464312625445,0.63183026057425,0.758196208523054,
0.884562416886973,1.01092862525089,1.13729483361481,1.26366104197873,1.39002698992753,
1.51639293787634,1.64275888582514,1.76912483377395,1.89549104213786,2.02185725050178),
 .UNSPECIFIED.);
#841=B_SPLINE_CURVE_WITH_KNOTS('',3,(#60331,#60332,#60333,#60334,#60335,
#60336,#60337,#60338,#60339,#60340,#60341,#60342,#60343,#60344,#60345,#60346,
#60347,#60348,#60349,#60350,#60351,#60352,#60353,#60354,#60355,#60356,#60357,
#60358,#60359,#60360,#60361,#60362,#60363,#60364),.UNSPECIFIED.,.T.,.F.,
(4,2,2,2,2,2,2,2,2,2,2,2,2,2,2,2,4),(0.,0.126366208363918,0.252732416727836,
0.37909836467664,0.505464312625445,0.631830260574249,0.758196208523054,
0.884562416886972,1.01092862525089,1.13729483361481,1.26366104197873,1.39002698992753,
1.51639293787633,1.64275888582514,1.76912483377394,1.89549104213786,2.02185725050178),
 .UNSPECIFIED.);
#842=B_SPLINE_CURVE_WITH_KNOTS('',3,(#60377,#60378,#60379,#60380),
 .UNSPECIFIED.,.F.,.F.,(4,4),(0.0184096978210031,0.0219555820656529),
 .UNSPECIFIED.);
#843=B_SPLINE_CURVE_WITH_KNOTS('',3,(#60382,#60383,#60384,#60385),
 .UNSPECIFIED.,.F.,.F.,(4,4),(0.0186156132125292,0.0221618161533775),
 .UNSPECIFIED.);
#910=TOROIDAL_SURFACE('',#38057,56.233130266379,1.78815999999988);
#934=SHAPE_REPRESENTATION_RELATIONSHIP('SRR','None',#61996,#959);
#959=ADVANCED_BREP_SHAPE_REPRESENTATION('',(#21),#61809);
#998=STYLED_ITEM('',(#62170),#21);
#1751=CYLINDRICAL_SURFACE('',#37256,3.22047616000001);
#1752=CYLINDRICAL_SURFACE('',#37257,3.9116);
#1753=CYLINDRICAL_SURFACE('',#37264,4.19099999999999);
#1754=CYLINDRICAL_SURFACE('',#37273,3.22047616000001);
#1755=CYLINDRICAL_SURFACE('',#37274,3.91160000000001);
#1756=CYLINDRICAL_SURFACE('',#37281,4.19099999999999);
#1757=CYLINDRICAL_SURFACE('',#37287,2.74750784000002);
#1758=CYLINDRICAL_SURFACE('',#37291,3.3527999999999);
#1759=CYLINDRICAL_SURFACE('',#37296,3.6322);
#1760=CYLINDRICAL_SURFACE('',#37299,3.9116);
#1761=CYLINDRICAL_SURFACE('',#37304,4.191);
#1762=CYLINDRICAL_SURFACE('',#37312,3.22047616000001);
#1763=CYLINDRICAL_SURFACE('',#37316,3.91160000000001);
#1764=CYLINDRICAL_SURFACE('',#37321,4.19099999999999);
#1765=CYLINDRICAL_SURFACE('',#37329,3.22047616000001);
#1766=CYLINDRICAL_SURFACE('',#37354,4.70822528);
#1767=CYLINDRICAL_SURFACE('',#37364,4.70822528000001);
#1768=CYLINDRICAL_SURFACE('',#37372,4.70822528000003);
#1769=CYLINDRICAL_SURFACE('',#37377,4.70822527999992);
#1770=CYLINDRICAL_SURFACE('',#37385,28.8698432);
#1771=CYLINDRICAL_SURFACE('',#37392,28.8519616);
#1772=CYLINDRICAL_SURFACE('',#37408,4.70822528000001);
#1773=CYLINDRICAL_SURFACE('',#37412,4.70822528);
#1774=CYLINDRICAL_SURFACE('',#37416,4.70822528000001);
#1775=CYLINDRICAL_SURFACE('',#37420,4.70822528000002);
#1776=CYLINDRICAL_SURFACE('',#37432,22.5);
#1777=CYLINDRICAL_SURFACE('',#37519,2.74750784);
#1778=CYLINDRICAL_SURFACE('',#37527,2.74750784000001);
#1779=CYLINDRICAL_SURFACE('',#37535,2.74750784);
#1780=CYLINDRICAL_SURFACE('',#37544,3.2204761600001);
#1781=CYLINDRICAL_SURFACE('',#37552,3.22047616000001);
#1782=CYLINDRICAL_SURFACE('',#37560,3.22047616000007);
#1783=CYLINDRICAL_SURFACE('',#37568,3.22047616000001);
#1784=CYLINDRICAL_SURFACE('',#37592,46.9481408);
#1785=CYLINDRICAL_SURFACE('',#37614,30.1930816);
#1786=CYLINDRICAL_SURFACE('',#37617,67.056);
#1787=CYLINDRICAL_SURFACE('',#37620,46.9481408);
#1788=CYLINDRICAL_SURFACE('',#37630,67.0291776);
#1789=CYLINDRICAL_SURFACE('',#37633,2.74750783999999);
#1790=CYLINDRICAL_SURFACE('',#37647,13.4268464);
#1791=CYLINDRICAL_SURFACE('',#37649,2.74750784);
#1792=CYLINDRICAL_SURFACE('',#37673,3.3528);
#1793=CYLINDRICAL_SURFACE('',#37703,3.35280000000001);
#1794=CYLINDRICAL_SURFACE('',#37714,3.3528);
#1795=CYLINDRICAL_SURFACE('',#37718,2.74750783999998);
#1796=CYLINDRICAL_SURFACE('',#37719,2.74750784000003);
#1797=CYLINDRICAL_SURFACE('',#37723,3.3528);
#1798=CYLINDRICAL_SURFACE('',#37724,37.9894592000001);
#1799=CYLINDRICAL_SURFACE('',#37732,37.9894592000001);
#1800=CYLINDRICAL_SURFACE('',#37738,46.9481408);
#1801=CYLINDRICAL_SURFACE('',#37739,37.9894592000001);
#1802=CYLINDRICAL_SURFACE('',#37744,46.9481408);
#1803=CYLINDRICAL_SURFACE('',#37789,2.74750784);
#1804=CYLINDRICAL_SURFACE('',#37792,2.74750784000001);
#1805=CYLINDRICAL_SURFACE('',#37795,21.82583392);
#1806=CYLINDRICAL_SURFACE('',#37797,3.63219999999997);
#1807=CYLINDRICAL_SURFACE('',#37800,3.63219999999997);
#1808=CYLINDRICAL_SURFACE('',#37803,3.63219999999999);
#1809=CYLINDRICAL_SURFACE('',#37806,3.63219999999999);
#1810=CYLINDRICAL_SURFACE('',#37817,2.14579200000041);
#1811=CYLINDRICAL_SURFACE('',#37820,55.4329599999993);
#1812=CYLINDRICAL_SURFACE('',#37823,2.14579200000012);
#1813=CYLINDRICAL_SURFACE('',#37827,2.14579200000009);
#1814=CYLINDRICAL_SURFACE('',#37830,45.0616320000007);
#1815=CYLINDRICAL_SURFACE('',#37833,2.145792);
#1816=CYLINDRICAL_SURFACE('',#37838,2.14579200000016);
#1817=CYLINDRICAL_SURFACE('',#37841,55.4329600000005);
#1818=CYLINDRICAL_SURFACE('',#37844,2.14579199999963);
#1819=CYLINDRICAL_SURFACE('',#37848,2.14579199999972);
#1820=CYLINDRICAL_SURFACE('',#37851,45.0616320000002);
#1821=CYLINDRICAL_SURFACE('',#37854,2.14579199999999);
#1822=CYLINDRICAL_SURFACE('',#37859,2.14579199999966);
#1823=CYLINDRICAL_SURFACE('',#37862,55.432960000003);
#1824=CYLINDRICAL_SURFACE('',#37865,2.14579200000016);
#1825=CYLINDRICAL_SURFACE('',#37869,2.14579199999998);
#1826=CYLINDRICAL_SURFACE('',#37872,45.0616319999968);
#1827=CYLINDRICAL_SURFACE('',#37875,2.14579199999998);
#1828=CYLINDRICAL_SURFACE('',#37879,3.63219999999999);
#1829=CYLINDRICAL_SURFACE('',#37881,3.63220000000001);
#1830=CYLINDRICAL_SURFACE('',#37883,3.63220000000001);
#1831=CYLINDRICAL_SURFACE('',#37885,40.2514816000001);
#1832=CYLINDRICAL_SURFACE('',#37891,40.251481599999);
#1833=CYLINDRICAL_SURFACE('',#37897,40.2514815999998);
#1834=CYLINDRICAL_SURFACE('',#37942,8.94079999999995);
#1835=CYLINDRICAL_SURFACE('',#37946,8.9408000000001);
#1836=CYLINDRICAL_SURFACE('',#37949,8.94079999999996);
#1837=CYLINDRICAL_SURFACE('',#37952,8.94080000000006);
#1838=CYLINDRICAL_SURFACE('',#37955,40.2514815999993);
#1839=CYLINDRICAL_SURFACE('',#37959,2.14579200000032);
#1840=CYLINDRICAL_SURFACE('',#37963,2.14579199999841);
#1841=CYLINDRICAL_SURFACE('',#37966,45.0616320000031);
#1842=CYLINDRICAL_SURFACE('',#37969,2.14579199999958);
#1843=CYLINDRICAL_SURFACE('',#37973,2.1457920000008);
#1844=CYLINDRICAL_SURFACE('',#37976,55.4329600000096);
#1845=CYLINDRICAL_SURFACE('',#37981,2.14579199999998);
#1846=CYLINDRICAL_SURFACE('',#37984,45.0616319999932);
#1847=CYLINDRICAL_SURFACE('',#37987,2.14579199999989);
#1848=CYLINDRICAL_SURFACE('',#37991,2.14579199999978);
#1849=CYLINDRICAL_SURFACE('',#37994,55.4329600000042);
#1850=CYLINDRICAL_SURFACE('',#37997,2.14579200000232);
#1851=CYLINDRICAL_SURFACE('',#38001,55.4329599999945);
#1852=CYLINDRICAL_SURFACE('',#38004,2.14579199999928);
#1853=CYLINDRICAL_SURFACE('',#38008,2.14579200000044);
#1854=CYLINDRICAL_SURFACE('',#38011,45.0616320000025);
#1855=CYLINDRICAL_SURFACE('',#38014,2.14579200000129);
#1856=CYLINDRICAL_SURFACE('',#38018,2.14579199999758);
#1857=CYLINDRICAL_SURFACE('',#38022,55.4329600000029);
#1858=CYLINDRICAL_SURFACE('',#38025,2.14579199999957);
#1859=CYLINDRICAL_SURFACE('',#38029,2.1457920000006);
#1860=CYLINDRICAL_SURFACE('',#38032,45.0616319999986);
#1861=CYLINDRICAL_SURFACE('',#38035,2.14579199999942);
#1862=CYLINDRICAL_SURFACE('',#38039,2.14579200000082);
#1863=CYLINDRICAL_SURFACE('',#38043,45.0616319999982);
#1864=CYLINDRICAL_SURFACE('',#38045,2.1457920000002);
#1865=CYLINDRICAL_SURFACE('',#38048,2.14579199999973);
#1866=CYLINDRICAL_SURFACE('',#38050,55.4329600000018);
#1867=CYLINDRICAL_SURFACE('',#38052,2.14579199999995);
#1868=CYLINDRICAL_SURFACE('',#38054,2.145792);
#1869=CYLINDRICAL_SURFACE('',#38075,5.02472959999993);
#2137=FACE_BOUND('',#7787,.T.);
#2138=FACE_BOUND('',#7789,.T.);
#2139=FACE_BOUND('',#7797,.T.);
#2140=FACE_BOUND('',#7799,.T.);
#2141=FACE_BOUND('',#7807,.T.);
#2142=FACE_BOUND('',#7810,.T.);
#2143=FACE_BOUND('',#7813,.T.);
#2144=FACE_BOUND('',#7816,.T.);
#2145=FACE_BOUND('',#7823,.T.);
#2146=FACE_BOUND('',#7826,.T.);
#2147=FACE_BOUND('',#7841,.T.);
#2148=FACE_BOUND('',#7845,.T.);
#2149=FACE_BOUND('',#7846,.T.);
#2150=FACE_BOUND('',#7847,.T.);
#2151=FACE_BOUND('',#7848,.T.);
#2152=FACE_BOUND('',#7868,.T.);
#2153=FACE_BOUND('',#7877,.T.);
#2154=FACE_BOUND('',#7928,.T.);
#2155=FACE_BOUND('',#7938,.T.);
#2156=FACE_BOUND('',#7943,.T.);
#2157=FACE_BOUND('',#7983,.T.);
#2158=FACE_BOUND('',#7985,.T.);
#2159=FACE_BOUND('',#7989,.T.);
#2160=FACE_BOUND('',#7990,.T.);
#2161=FACE_BOUND('',#7991,.T.);
#2162=FACE_BOUND('',#7992,.T.);
#2163=FACE_BOUND('',#8001,.T.);
#2164=FACE_BOUND('',#8002,.T.);
#2165=FACE_BOUND('',#8003,.T.);
#2166=FACE_BOUND('',#8004,.T.);
#2167=FACE_BOUND('',#8005,.T.);
#2168=FACE_BOUND('',#8018,.T.);
#2169=FACE_BOUND('',#8019,.T.);
#2170=FACE_BOUND('',#8020,.T.);
#2171=FACE_BOUND('',#8021,.T.);
#2172=FACE_BOUND('',#8022,.T.);
#2173=FACE_BOUND('',#8024,.T.);
#2174=FACE_BOUND('',#8027,.T.);
#2175=FACE_BOUND('',#8031,.T.);
#2176=FACE_BOUND('',#8034,.T.);
#2177=FACE_BOUND('',#8036,.T.);
#2178=FACE_BOUND('',#8037,.T.);
#2179=FACE_BOUND('',#8040,.T.);
#2180=FACE_BOUND('',#8041,.T.);
#2181=FACE_BOUND('',#8057,.T.);
#2182=FACE_BOUND('',#8063,.T.);
#2183=FACE_BOUND('',#8080,.T.);
#2184=FACE_BOUND('',#8086,.T.);
#2185=FACE_BOUND('',#8097,.T.);
#2186=FACE_BOUND('',#8098,.T.);
#2187=FACE_BOUND('',#8104,.T.);
#2188=FACE_BOUND('',#8105,.T.);
#2189=FACE_BOUND('',#8107,.T.);
#2190=FACE_BOUND('',#8109,.T.);
#2191=FACE_BOUND('',#8113,.T.);
#2192=FACE_BOUND('',#8115,.T.);
#2193=FACE_BOUND('',#8144,.T.);
#2194=FACE_BOUND('',#8146,.T.);
#2195=FACE_BOUND('',#8148,.T.);
#2196=FACE_BOUND('',#8194,.T.);
#2197=FACE_BOUND('',#8196,.T.);
#2198=FACE_BOUND('',#8198,.T.);
#2199=FACE_BOUND('',#8213,.T.);
#2200=FACE_BOUND('',#8227,.T.);
#2201=FACE_BOUND('',#8276,.T.);
#2202=FACE_BOUND('',#8277,.T.);
#2203=FACE_BOUND('',#8278,.T.);
#2204=FACE_BOUND('',#8279,.T.);
#2205=FACE_BOUND('',#8280,.T.);
#2206=FACE_BOUND('',#8281,.T.);
#2207=FACE_BOUND('',#8282,.T.);
#2208=FACE_BOUND('',#8289,.T.);
#2209=FACE_BOUND('',#8290,.T.);
#2210=FACE_BOUND('',#8291,.T.);
#2211=FACE_BOUND('',#8292,.T.);
#2212=FACE_BOUND('',#8293,.T.);
#2213=FACE_BOUND('',#8294,.T.);
#2214=FACE_BOUND('',#8295,.T.);
#2215=FACE_BOUND('',#8296,.T.);
#2216=FACE_BOUND('',#8297,.T.);
#2217=FACE_BOUND('',#8298,.T.);
#2218=FACE_BOUND('',#8299,.T.);
#2219=FACE_BOUND('',#8300,.T.);
#2220=FACE_BOUND('',#8301,.T.);
#2221=FACE_BOUND('',#8302,.T.);
#2222=FACE_BOUND('',#8303,.T.);
#2223=FACE_BOUND('',#8308,.T.);
#2224=FACE_BOUND('',#8320,.T.);
#3847=CIRCLE('',#37249,3.22047616);
#3848=CIRCLE('',#37250,3.22047616);
#3849=CIRCLE('',#37251,3.15163199999999);
#3850=CIRCLE('',#37254,3.22047616);
#3851=CIRCLE('',#37255,3.22047616);
#3852=CIRCLE('',#37258,3.9116);
#3853=CIRCLE('',#37259,3.9116);
#3854=CIRCLE('',#37261,4.19099999999999);
#3855=CIRCLE('',#37263,4.19100000000001);
#3856=CIRCLE('',#37266,3.22047616);
#3857=CIRCLE('',#37267,3.22047616);
#3858=CIRCLE('',#37268,3.151632);
#3859=CIRCLE('',#37271,3.22047616000001);
#3860=CIRCLE('',#37272,3.22047616000001);
#3861=CIRCLE('',#37275,3.9116);
#3862=CIRCLE('',#37276,3.9116);
#3863=CIRCLE('',#37278,4.19099999999999);
#3864=CIRCLE('',#37280,4.191);
#3865=CIRCLE('',#37283,2.74750784);
#3866=CIRCLE('',#37284,2.68671039999999);
#3867=CIRCLE('',#37285,2.74750784);
#3868=CIRCLE('',#37288,2.74750784);
#3869=CIRCLE('',#37289,2.74750784);
#3870=CIRCLE('',#37292,3.3528);
#3871=CIRCLE('',#37293,3.35280000000001);
#3872=CIRCLE('',#37295,3.6322);
#3873=CIRCLE('',#37297,3.6322);
#3874=CIRCLE('',#37300,3.9116);
#3875=CIRCLE('',#37301,3.9116);
#3876=CIRCLE('',#37303,4.191);
#3877=CIRCLE('',#37305,4.19099999999999);
#3878=CIRCLE('',#37308,3.22047616);
#3879=CIRCLE('',#37309,3.22047616);
#3880=CIRCLE('',#37310,3.15163200000001);
#3881=CIRCLE('',#37313,3.22047616);
#3882=CIRCLE('',#37314,3.22047616);
#3883=CIRCLE('',#37317,3.9116);
#3884=CIRCLE('',#37318,3.9116);
#3885=CIRCLE('',#37320,4.191);
#3886=CIRCLE('',#37322,4.191);
#3887=CIRCLE('',#37325,3.22047616000001);
#3888=CIRCLE('',#37326,3.22047616000001);
#3889=CIRCLE('',#37327,3.151632);
#3890=CIRCLE('',#37330,3.22047616);
#3891=CIRCLE('',#37331,3.22047616);
#3892=CIRCLE('',#37335,62.3964875794553);
#3893=CIRCLE('',#37336,60.8301548187703);
#3894=CIRCLE('',#37339,62.3964875794704);
#3895=CIRCLE('',#37340,60.8301548187776);
#3896=CIRCLE('',#37344,13.9758160535843);
#3897=CIRCLE('',#37346,13.9758160535819);
#3898=CIRCLE('',#37349,17.7292483264849);
#3899=CIRCLE('',#37350,17.729248326485);
#3900=CIRCLE('',#37351,17.7292483264851);
#3901=CIRCLE('',#37352,17.7292483264851);
#3902=CIRCLE('',#37353,30.1930816);
#3903=CIRCLE('',#37355,4.70822528);
#3904=CIRCLE('',#37356,4.70822528);
#3905=CIRCLE('',#37357,4.70822528);
#3906=CIRCLE('',#37361,4.70822528);
#3907=CIRCLE('',#37362,4.70822528);
#3908=CIRCLE('',#37363,4.70822528000005);
#3909=CIRCLE('',#37365,4.70822528);
#3910=CIRCLE('',#37366,4.70822528);
#3911=CIRCLE('',#37373,4.70822528000005);
#3912=CIRCLE('',#37374,4.70822528000005);
#3913=CIRCLE('',#37378,4.70822527999999);
#3914=CIRCLE('',#37379,4.70822527999999);
#3915=CIRCLE('',#37384,5.87573292967013);
#3916=CIRCLE('',#37386,28.8698432);
#3917=CIRCLE('',#37387,28.8698432);
#3918=CIRCLE('',#37388,28.8698432);
#3919=CIRCLE('',#37389,28.8698432);
#3920=CIRCLE('',#37393,28.8519616);
#3921=CIRCLE('',#37394,28.8519616);
#3922=CIRCLE('',#37395,28.8519616);
#3923=CIRCLE('',#37405,27.9578816);
#3924=CIRCLE('',#37407,21.82583392);
#3925=CIRCLE('',#37409,4.70822527999999);
#3926=CIRCLE('',#37410,4.70822527999999);
#3927=CIRCLE('',#37411,4.70822528);
#3928=CIRCLE('',#37413,4.70822528);
#3929=CIRCLE('',#37414,4.70822528);
#3930=CIRCLE('',#37415,4.70822528);
#3931=CIRCLE('',#37417,4.70822528);
#3932=CIRCLE('',#37418,4.70822528);
#3933=CIRCLE('',#37419,4.70822528);
#3934=CIRCLE('',#37421,4.70822528);
#3935=CIRCLE('',#37422,4.70822528);
#3936=CIRCLE('',#37423,4.70822528);
#3937=CIRCLE('',#37428,5.87573292967001);
#3938=CIRCLE('',#37429,5.87573292967001);
#3939=CIRCLE('',#37431,14.6657199888249);
#3940=CIRCLE('',#37433,22.5);
#3941=CIRCLE('',#37434,22.5);
#3942=CIRCLE('',#37441,5.64835039999983);
#3943=CIRCLE('',#37443,5.6483504000001);
#3944=CIRCLE('',#37445,5.64835039999984);
#3945=CIRCLE('',#37447,5.64835040000001);
#3946=CIRCLE('',#37449,5.64835039999994);
#3947=CIRCLE('',#37453,5.64835039999982);
#3948=CIRCLE('',#37460,5.64835040000232);
#3949=CIRCLE('',#37462,5.64835039999654);
#3950=CIRCLE('',#37464,5.64835040000021);
#3951=CIRCLE('',#37466,5.64835039999982);
#3952=CIRCLE('',#37468,5.64835040000023);
#3953=CIRCLE('',#37472,5.64835040000259);
#3954=CIRCLE('',#37487,5.17762544927992);
#3955=CIRCLE('',#37489,5.17762544927979);
#3956=CIRCLE('',#37498,5.17762544928);
#3957=CIRCLE('',#37508,5.17762544927989);
#3958=CIRCLE('',#37514,5.44243151077326);
#3959=CIRCLE('',#37517,2.74750784);
#3960=CIRCLE('',#37518,2.74750784);
#3961=CIRCLE('',#37520,2.74750784);
#3962=CIRCLE('',#37521,2.74750784);
#3963=CIRCLE('',#37523,3.35280000000001);
#3964=CIRCLE('',#37525,2.74750784);
#3965=CIRCLE('',#37526,2.74750784);
#3966=CIRCLE('',#37528,2.74750784000001);
#3967=CIRCLE('',#37529,2.74750784000001);
#3968=CIRCLE('',#37531,3.3528);
#3969=CIRCLE('',#37533,2.74750784);
#3970=CIRCLE('',#37534,2.74750784);
#3971=CIRCLE('',#37536,2.74750784000001);
#3972=CIRCLE('',#37537,2.74750784000001);
#3973=CIRCLE('',#37539,3.3528);
#3974=CIRCLE('',#37541,3.22047616000005);
#3975=CIRCLE('',#37542,3.22047616000005);
#3976=CIRCLE('',#37543,3.9116);
#3977=CIRCLE('',#37545,3.22047616000005);
#3978=CIRCLE('',#37546,3.22047616000005);
#3979=CIRCLE('',#37549,3.22047616);
#3980=CIRCLE('',#37550,3.22047616);
#3981=CIRCLE('',#37551,3.9116);
#3982=CIRCLE('',#37553,3.22047616);
#3983=CIRCLE('',#37554,3.22047616);
#3984=CIRCLE('',#37557,3.22047616000005);
#3985=CIRCLE('',#37558,3.22047616000005);
#3986=CIRCLE('',#37559,3.9116);
#3987=CIRCLE('',#37561,3.22047616000005);
#3988=CIRCLE('',#37562,3.22047616000005);
#3989=CIRCLE('',#37565,3.22047616000001);
#3990=CIRCLE('',#37566,3.22047616000001);
#3991=CIRCLE('',#37567,3.9116);
#3992=CIRCLE('',#37569,3.22047616000001);
#3993=CIRCLE('',#37570,3.22047616000001);
#3994=CIRCLE('',#37590,67.056);
#3995=CIRCLE('',#37591,46.9481408);
#3996=CIRCLE('',#37593,46.9481408);
#3997=CIRCLE('',#37595,46.9481408);
#3998=CIRCLE('',#37596,47.4643381286771);
#3999=CIRCLE('',#37597,46.9481408);
#4000=CIRCLE('',#37611,67.056);
#4001=CIRCLE('',#37612,67.056);
#4002=CIRCLE('',#37613,67.6754367944125);
#4003=CIRCLE('',#37616,29.386040528677);
#4004=CIRCLE('',#37621,46.9481408);
#4005=CIRCLE('',#37622,46.9481408);
#4006=CIRCLE('',#37624,46.9481408);
#4007=CIRCLE('',#37625,46.9481408);
#4008=CIRCLE('',#37626,47.4643381286771);
#4009=CIRCLE('',#37629,67.0291776);
#4010=CIRCLE('',#37631,67.0291776000001);
#4011=CIRCLE('',#37634,2.74750784);
#4012=CIRCLE('',#37635,2.74750784);
#4013=CIRCLE('',#37636,2.74750784);
#4014=CIRCLE('',#37638,37.9894592000001);
#4015=CIRCLE('',#37639,37.9894592000001);
#4016=CIRCLE('',#37640,37.3700224055875);
#4017=CIRCLE('',#37642,14.6657199888249);
#4018=CIRCLE('',#37644,13.4268464);
#4019=CIRCLE('',#37646,28.7097683677432);
#4020=CIRCLE('',#37648,13.4268464);
#4021=CIRCLE('',#37650,2.74750784);
#4022=CIRCLE('',#37651,2.74750784);
#4023=CIRCLE('',#37652,2.74750784);
#4024=CIRCLE('',#37669,2.68671040000002);
#4025=CIRCLE('',#37671,3.35279999999999);
#4026=CIRCLE('',#37672,3.35279999999999);
#4027=CIRCLE('',#37675,2.74750783999999);
#4028=CIRCLE('',#37676,2.74750783999999);
#4029=CIRCLE('',#37677,2.6867104);
#4030=CIRCLE('',#37680,2.68671040000002);
#4031=CIRCLE('',#37682,3.3528);
#4032=CIRCLE('',#37683,3.3528);
#4033=CIRCLE('',#37699,2.6867104);
#4034=CIRCLE('',#37701,3.35279999999998);
#4035=CIRCLE('',#37702,3.35279999999998);
#4036=CIRCLE('',#37705,2.74750783999999);
#4037=CIRCLE('',#37706,2.74750783999999);
#4038=CIRCLE('',#37707,2.6867104);
#4039=CIRCLE('',#37710,2.6867104);
#4040=CIRCLE('',#37712,3.3528);
#4041=CIRCLE('',#37713,3.3528);
#4042=CIRCLE('',#37716,2.6867104);
#4043=CIRCLE('',#37721,2.6867104);
#4044=CIRCLE('',#37725,37.9894592000001);
#4045=CIRCLE('',#37726,37.9894592000001);
#4046=CIRCLE('',#37727,37.9894592);
#4047=CIRCLE('',#37733,37.9894592);
#4048=CIRCLE('',#37735,37.9894592);
#4049=CIRCLE('',#37737,46.9481408);
#4050=CIRCLE('',#37740,37.9894592);
#4051=CIRCLE('',#37743,46.9481408);
#4052=CIRCLE('',#37746,5.64835039999681);
#4053=CIRCLE('',#37747,5.64835040000208);
#4054=CIRCLE('',#37748,5.64835039999998);
#4055=CIRCLE('',#37749,5.64835040000009);
#4056=CIRCLE('',#37750,5.64835040000009);
#4057=CIRCLE('',#37751,5.64835040000243);
#4058=CIRCLE('',#37765,5.64835039999982);
#4059=CIRCLE('',#37766,5.64835040000004);
#4060=CIRCLE('',#37767,5.64835040000006);
#4061=CIRCLE('',#37768,5.64835039999973);
#4062=CIRCLE('',#37769,5.64835039999998);
#4063=CIRCLE('',#37770,5.64835039999987);
#4064=CIRCLE('',#37784,3.63220000000001);
#4065=CIRCLE('',#37786,3.6322);
#4066=CIRCLE('',#37788,3.63220000000001);
#4067=CIRCLE('',#37790,2.74750784);
#4068=CIRCLE('',#37791,2.74750784);
#4069=CIRCLE('',#37793,2.74750784);
#4070=CIRCLE('',#37794,2.74750784);
#4071=CIRCLE('',#37796,21.82583392);
#4072=CIRCLE('',#37798,3.6322);
#4073=CIRCLE('',#37799,3.6322);
#4074=CIRCLE('',#37801,3.6322);
#4075=CIRCLE('',#37802,3.6322);
#4076=CIRCLE('',#37804,3.6322);
#4077=CIRCLE('',#37805,3.6322);
#4078=CIRCLE('',#37807,3.6322);
#4079=CIRCLE('',#37808,3.6322);
#4080=CIRCLE('',#37810,45.0616320000016);
#4081=CIRCLE('',#37811,2.14579199999995);
#4082=CIRCLE('',#37812,2.14579200000003);
#4083=CIRCLE('',#37813,55.4329599999972);
#4084=CIRCLE('',#37814,2.14579200000022);
#4085=CIRCLE('',#37815,2.14579200000003);
#4086=CIRCLE('',#37818,2.14579200000017);
#4087=CIRCLE('',#37819,2.14579200000006);
#4088=CIRCLE('',#37821,55.4329599999999);
#4089=CIRCLE('',#37822,55.4329599999999);
#4090=CIRCLE('',#37824,2.14579200000009);
#4091=CIRCLE('',#37825,2.14579199999991);
#4092=CIRCLE('',#37828,2.14579200000003);
#4093=CIRCLE('',#37829,2.14579200000003);
#4094=CIRCLE('',#37831,45.0616320000003);
#4095=CIRCLE('',#37832,45.0616320000003);
#4096=CIRCLE('',#37834,2.14579199999998);
#4097=CIRCLE('',#37835,2.14579199999998);
#4098=CIRCLE('',#37839,2.14579200000001);
#4099=CIRCLE('',#37840,2.14579200000002);
#4100=CIRCLE('',#37842,55.4329600000002);
#4101=CIRCLE('',#37843,55.4329600000002);
#4102=CIRCLE('',#37845,2.14579200000004);
#4103=CIRCLE('',#37846,2.14579200000004);
#4104=CIRCLE('',#37849,2.1457919999999);
#4105=CIRCLE('',#37850,2.14579200000004);
#4106=CIRCLE('',#37852,45.0616320000005);
#4107=CIRCLE('',#37853,45.0616320000005);
#4108=CIRCLE('',#37855,2.14579199999994);
#4109=CIRCLE('',#37856,2.14579199999996);
#4110=CIRCLE('',#37860,2.14579200000037);
#4111=CIRCLE('',#37861,2.14579200000037);
#4112=CIRCLE('',#37863,55.432960000001);
#4113=CIRCLE('',#37864,55.432960000001);
#4114=CIRCLE('',#37866,2.14579200000004);
#4115=CIRCLE('',#37867,2.14579200000016);
#4116=CIRCLE('',#37870,2.14579199999993);
#4117=CIRCLE('',#37871,2.14579200000008);
#4118=CIRCLE('',#37873,45.0616319999978);
#4119=CIRCLE('',#37874,45.0616319999978);
#4120=CIRCLE('',#37876,2.14579200000014);
#4121=CIRCLE('',#37877,2.14579200000014);
#4122=CIRCLE('',#37880,3.6322);
#4123=CIRCLE('',#37882,3.6322);
#4124=CIRCLE('',#37884,3.6322);
#4125=CIRCLE('',#37886,40.2514816);
#4126=CIRCLE('',#37888,40.2514816000002);
#4127=CIRCLE('',#37892,40.2514816000021);
#4128=CIRCLE('',#37893,1249.18823030311);
#4129=CIRCLE('',#37894,40.2514815999989);
#4130=CIRCLE('',#37895,1249.18823049325);
#4131=CIRCLE('',#37899,40.2514815999998);
#4132=CIRCLE('',#37901,40.2514815999992);
#4133=CIRCLE('',#37904,8.94079999999999);
#4134=CIRCLE('',#37905,8.5349144993668);
#4135=CIRCLE('',#37907,8.53491449936691);
#4136=CIRCLE('',#37908,8.94079999999999);
#4137=CIRCLE('',#37910,8.5349144993666);
#4138=CIRCLE('',#37911,8.9408);
#4139=CIRCLE('',#37912,4.91296959999996);
#4140=CIRCLE('',#37914,58.1152000000001);
#4141=CIRCLE('',#37915,58.0210179209497);
#4142=CIRCLE('',#37916,58.0210179209497);
#4143=CIRCLE('',#37923,8.94080000000002);
#4144=CIRCLE('',#37926,8.94079999999995);
#4145=CIRCLE('',#37929,8.53491449936659);
#4146=CIRCLE('',#37930,8.94079999999992);
#4147=CIRCLE('',#37932,1249.18889184763);
#4148=CIRCLE('',#37933,1249.18889156446);
#4149=CIRCLE('',#37935,8.94080000000007);
#4150=CIRCLE('',#37937,8.94079999999999);
#4151=CIRCLE('',#37938,8.94079999999999);
#4152=CIRCLE('',#37939,8.94080000000001);
#4153=CIRCLE('',#37940,8.94079999999999);
#4154=CIRCLE('',#37943,8.94079999999999);
#4155=CIRCLE('',#37956,40.2514816000013);
#4156=CIRCLE('',#37957,40.2514815999992);
#4157=CIRCLE('',#37960,2.14579200000002);
#4158=CIRCLE('',#37961,2.14579200000014);
#4159=CIRCLE('',#37964,2.14579199999958);
#4160=CIRCLE('',#37965,2.14579199999958);
#4161=CIRCLE('',#37967,45.0616320000041);
#4162=CIRCLE('',#37968,45.061632000004);
#4163=CIRCLE('',#37970,2.14579200000037);
#4164=CIRCLE('',#37971,2.14579200000037);
#4165=CIRCLE('',#37974,2.14579200000006);
#4166=CIRCLE('',#37975,2.14579200000006);
#4167=CIRCLE('',#37977,55.4329600000085);
#4168=CIRCLE('',#37978,55.4329600000085);
#4169=CIRCLE('',#37982,2.14579200000079);
#4170=CIRCLE('',#37983,2.14579200000084);
#4171=CIRCLE('',#37985,45.0616319999978);
#4172=CIRCLE('',#37986,45.0616319999971);
#4173=CIRCLE('',#37988,2.14579199999999);
#4174=CIRCLE('',#37989,2.14579199999999);
#4175=CIRCLE('',#37992,2.14579200000036);
#4176=CIRCLE('',#37993,2.14579200000036);
#4177=CIRCLE('',#37995,55.4329600000016);
#4178=CIRCLE('',#37996,55.4329600000016);
#4179=CIRCLE('',#37998,2.14579199999924);
#4180=CIRCLE('',#37999,2.14579199999924);
#4181=CIRCLE('',#38002,55.4329599999945);
#4182=CIRCLE('',#38003,55.4329599999945);
#4183=CIRCLE('',#38005,2.1457919999994);
#4184=CIRCLE('',#38006,2.1457919999994);
#4185=CIRCLE('',#38009,2.14579200000024);
#4186=CIRCLE('',#38010,2.14579200000024);
#4187=CIRCLE('',#38012,45.0616320000037);
#4188=CIRCLE('',#38013,45.0616320000037);
#4189=CIRCLE('',#38015,2.1457919999996);
#4190=CIRCLE('',#38016,2.1457919999996);
#4191=CIRCLE('',#38019,2.14579200000019);
#4192=CIRCLE('',#38020,2.14579200000016);
#4193=CIRCLE('',#38023,55.4329599999988);
#4194=CIRCLE('',#38024,55.432959999998);
#4195=CIRCLE('',#38026,2.1457920000003);
#4196=CIRCLE('',#38027,2.1457920000003);
#4197=CIRCLE('',#38030,2.14579200000034);
#4198=CIRCLE('',#38031,2.14579200000023);
#4199=CIRCLE('',#38033,45.0616319999981);
#4200=CIRCLE('',#38034,45.0616319999962);
#4201=CIRCLE('',#38036,2.14579199999954);
#4202=CIRCLE('',#38037,2.14579199999954);
#4203=CIRCLE('',#38040,2.14579199999923);
#4204=CIRCLE('',#38041,2.14579199999923);
#4205=CIRCLE('',#38044,45.0616320000016);
#4206=CIRCLE('',#38046,2.14579200000003);
#4207=CIRCLE('',#38049,2.14579200000008);
#4208=CIRCLE('',#38051,55.4329599999972);
#4209=CIRCLE('',#38053,2.14579200000014);
#4210=CIRCLE('',#38055,2.14579199999995);
#4211=CIRCLE('',#38058,1.78815999999988);
#4212=CIRCLE('',#38059,56.2331302663788);
#4213=CIRCLE('',#38072,5.0247296);
#4214=CIRCLE('',#38073,5.0247296);
#4215=CIRCLE('',#38074,4.5776896);
#4216=CIRCLE('',#38076,5.0247296);
#4217=CIRCLE('',#38077,5.0247296);
#5644=FACE_OUTER_BOUND('',#7781,.T.);
#5645=FACE_OUTER_BOUND('',#7782,.T.);
#5646=FACE_OUTER_BOUND('',#7783,.T.);
#5647=FACE_OUTER_BOUND('',#7784,.T.);
#5648=FACE_OUTER_BOUND('',#7785,.T.);
#5649=FACE_OUTER_BOUND('',#7786,.T.);
#5650=FACE_OUTER_BOUND('',#7788,.T.);
#5651=FACE_OUTER_BOUND('',#7790,.T.);
#5652=FACE_OUTER_BOUND('',#7791,.T.);
#5653=FACE_OUTER_BOUND('',#7792,.T.);
#5654=FACE_OUTER_BOUND('',#7793,.T.);
#5655=FACE_OUTER_BOUND('',#7794,.T.);
#5656=FACE_OUTER_BOUND('',#7795,.T.);
#5657=FACE_OUTER_BOUND('',#7796,.T.);
#5658=FACE_OUTER_BOUND('',#7798,.T.);
#5659=FACE_OUTER_BOUND('',#7800,.T.);
#5660=FACE_OUTER_BOUND('',#7801,.T.);
#5661=FACE_OUTER_BOUND('',#7802,.T.);
#5662=FACE_OUTER_BOUND('',#7803,.T.);
#5663=FACE_OUTER_BOUND('',#7804,.T.);
#5664=FACE_OUTER_BOUND('',#7805,.T.);
#5665=FACE_OUTER_BOUND('',#7806,.T.);
#5666=FACE_OUTER_BOUND('',#7808,.T.);
#5667=FACE_OUTER_BOUND('',#7809,.T.);
#5668=FACE_OUTER_BOUND('',#7811,.T.);
#5669=FACE_OUTER_BOUND('',#7812,.T.);
#5670=FACE_OUTER_BOUND('',#7814,.T.);
#5671=FACE_OUTER_BOUND('',#7815,.T.);
#5672=FACE_OUTER_BOUND('',#7817,.T.);
#5673=FACE_OUTER_BOUND('',#7818,.T.);
#5674=FACE_OUTER_BOUND('',#7819,.T.);
#5675=FACE_OUTER_BOUND('',#7820,.T.);
#5676=FACE_OUTER_BOUND('',#7821,.T.);
#5677=FACE_OUTER_BOUND('',#7822,.T.);
#5678=FACE_OUTER_BOUND('',#7824,.T.);
#5679=FACE_OUTER_BOUND('',#7825,.T.);
#5680=FACE_OUTER_BOUND('',#7827,.T.);
#5681=FACE_OUTER_BOUND('',#7828,.T.);
#5682=FACE_OUTER_BOUND('',#7829,.T.);
#5683=FACE_OUTER_BOUND('',#7830,.T.);
#5684=FACE_OUTER_BOUND('',#7831,.T.);
#5685=FACE_OUTER_BOUND('',#7832,.T.);
#5686=FACE_OUTER_BOUND('',#7833,.T.);
#5687=FACE_OUTER_BOUND('',#7834,.T.);
#5688=FACE_OUTER_BOUND('',#7835,.T.);
#5689=FACE_OUTER_BOUND('',#7836,.T.);
#5690=FACE_OUTER_BOUND('',#7837,.T.);
#5691=FACE_OUTER_BOUND('',#7838,.T.);
#5692=FACE_OUTER_BOUND('',#7839,.T.);
#5693=FACE_OUTER_BOUND('',#7840,.T.);
#5694=FACE_OUTER_BOUND('',#7842,.T.);
#5695=FACE_OUTER_BOUND('',#7843,.T.);
#5696=FACE_OUTER_BOUND('',#7844,.T.);
#5697=FACE_OUTER_BOUND('',#7849,.T.);
#5698=FACE_OUTER_BOUND('',#7850,.T.);
#5699=FACE_OUTER_BOUND('',#7851,.T.);
#5700=FACE_OUTER_BOUND('',#7852,.T.);
#5701=FACE_OUTER_BOUND('',#7853,.T.);
#5702=FACE_OUTER_BOUND('',#7854,.T.);
#5703=FACE_OUTER_BOUND('',#7855,.T.);
#5704=FACE_OUTER_BOUND('',#7856,.T.);
#5705=FACE_OUTER_BOUND('',#7857,.T.);
#5706=FACE_OUTER_BOUND('',#7858,.T.);
#5707=FACE_OUTER_BOUND('',#7859,.T.);
#5708=FACE_OUTER_BOUND('',#7860,.T.);
#5709=FACE_OUTER_BOUND('',#7861,.T.);
#5710=FACE_OUTER_BOUND('',#7862,.T.);
#5711=FACE_OUTER_BOUND('',#7863,.T.);
#5712=FACE_OUTER_BOUND('',#7864,.T.);
#5713=FACE_OUTER_BOUND('',#7865,.T.);
#5714=FACE_OUTER_BOUND('',#7866,.T.);
#5715=FACE_OUTER_BOUND('',#7867,.T.);
#5716=FACE_OUTER_BOUND('',#7869,.T.);
#5717=FACE_OUTER_BOUND('',#7870,.T.);
#5718=FACE_OUTER_BOUND('',#7871,.T.);
#5719=FACE_OUTER_BOUND('',#7872,.T.);
#5720=FACE_OUTER_BOUND('',#7873,.T.);
#5721=FACE_OUTER_BOUND('',#7874,.T.);
#5722=FACE_OUTER_BOUND('',#7875,.T.);
#5723=FACE_OUTER_BOUND('',#7876,.T.);
#5724=FACE_OUTER_BOUND('',#7878,.T.);
#5725=FACE_OUTER_BOUND('',#7879,.T.);
#5726=FACE_OUTER_BOUND('',#7880,.T.);
#5727=FACE_OUTER_BOUND('',#7881,.T.);
#5728=FACE_OUTER_BOUND('',#7882,.T.);
#5729=FACE_OUTER_BOUND('',#7883,.T.);
#5730=FACE_OUTER_BOUND('',#7884,.T.);
#5731=FACE_OUTER_BOUND('',#7885,.T.);
#5732=FACE_OUTER_BOUND('',#7886,.T.);
#5733=FACE_OUTER_BOUND('',#7887,.T.);
#5734=FACE_OUTER_BOUND('',#7888,.T.);
#5735=FACE_OUTER_BOUND('',#7889,.T.);
#5736=FACE_OUTER_BOUND('',#7890,.T.);
#5737=FACE_OUTER_BOUND('',#7891,.T.);
#5738=FACE_OUTER_BOUND('',#7892,.T.);
#5739=FACE_OUTER_BOUND('',#7893,.T.);
#5740=FACE_OUTER_BOUND('',#7894,.T.);
#5741=FACE_OUTER_BOUND('',#7895,.T.);
#5742=FACE_OUTER_BOUND('',#7896,.T.);
#5743=FACE_OUTER_BOUND('',#7897,.T.);
#5744=FACE_OUTER_BOUND('',#7898,.T.);
#5745=FACE_OUTER_BOUND('',#7899,.T.);
#5746=FACE_OUTER_BOUND('',#7900,.T.);
#5747=FACE_OUTER_BOUND('',#7901,.T.);
#5748=FACE_OUTER_BOUND('',#7902,.T.);
#5749=FACE_OUTER_BOUND('',#7903,.T.);
#5750=FACE_OUTER_BOUND('',#7904,.T.);
#5751=FACE_OUTER_BOUND('',#7905,.T.);
#5752=FACE_OUTER_BOUND('',#7906,.T.);
#5753=FACE_OUTER_BOUND('',#7907,.T.);
#5754=FACE_OUTER_BOUND('',#7908,.T.);
#5755=FACE_OUTER_BOUND('',#7909,.T.);
#5756=FACE_OUTER_BOUND('',#7910,.T.);
#5757=FACE_OUTER_BOUND('',#7911,.T.);
#5758=FACE_OUTER_BOUND('',#7912,.T.);
#5759=FACE_OUTER_BOUND('',#7913,.T.);
#5760=FACE_OUTER_BOUND('',#7914,.T.);
#5761=FACE_OUTER_BOUND('',#7915,.T.);
#5762=FACE_OUTER_BOUND('',#7916,.T.);
#5763=FACE_OUTER_BOUND('',#7917,.T.);
#5764=FACE_OUTER_BOUND('',#7918,.T.);
#5765=FACE_OUTER_BOUND('',#7919,.T.);
#5766=FACE_OUTER_BOUND('',#7920,.T.);
#5767=FACE_OUTER_BOUND('',#7921,.T.);
#5768=FACE_OUTER_BOUND('',#7922,.T.);
#5769=FACE_OUTER_BOUND('',#7923,.T.);
#5770=FACE_OUTER_BOUND('',#7924,.T.);
#5771=FACE_OUTER_BOUND('',#7925,.T.);
#5772=FACE_OUTER_BOUND('',#7926,.T.);
#5773=FACE_OUTER_BOUND('',#7927,.T.);
#5774=FACE_OUTER_BOUND('',#7929,.T.);
#5775=FACE_OUTER_BOUND('',#7930,.T.);
#5776=FACE_OUTER_BOUND('',#7931,.T.);
#5777=FACE_OUTER_BOUND('',#7932,.T.);
#5778=FACE_OUTER_BOUND('',#7933,.T.);
#5779=FACE_OUTER_BOUND('',#7934,.T.);
#5780=FACE_OUTER_BOUND('',#7935,.T.);
#5781=FACE_OUTER_BOUND('',#7936,.T.);
#5782=FACE_OUTER_BOUND('',#7937,.T.);
#5783=FACE_OUTER_BOUND('',#7939,.T.);
#5784=FACE_OUTER_BOUND('',#7940,.T.);
#5785=FACE_OUTER_BOUND('',#7941,.T.);
#5786=FACE_OUTER_BOUND('',#7942,.T.);
#5787=FACE_OUTER_BOUND('',#7944,.T.);
#5788=FACE_OUTER_BOUND('',#7945,.T.);
#5789=FACE_OUTER_BOUND('',#7946,.T.);
#5790=FACE_OUTER_BOUND('',#7947,.T.);
#5791=FACE_OUTER_BOUND('',#7948,.T.);
#5792=FACE_OUTER_BOUND('',#7949,.T.);
#5793=FACE_OUTER_BOUND('',#7950,.T.);
#5794=FACE_OUTER_BOUND('',#7951,.T.);
#5795=FACE_OUTER_BOUND('',#7952,.T.);
#5796=FACE_OUTER_BOUND('',#7953,.T.);
#5797=FACE_OUTER_BOUND('',#7954,.T.);
#5798=FACE_OUTER_BOUND('',#7955,.T.);
#5799=FACE_OUTER_BOUND('',#7956,.T.);
#5800=FACE_OUTER_BOUND('',#7957,.T.);
#5801=FACE_OUTER_BOUND('',#7958,.T.);
#5802=FACE_OUTER_BOUND('',#7959,.T.);
#5803=FACE_OUTER_BOUND('',#7960,.T.);
#5804=FACE_OUTER_BOUND('',#7961,.T.);
#5805=FACE_OUTER_BOUND('',#7962,.T.);
#5806=FACE_OUTER_BOUND('',#7963,.T.);
#5807=FACE_OUTER_BOUND('',#7964,.T.);
#5808=FACE_OUTER_BOUND('',#7965,.T.);
#5809=FACE_OUTER_BOUND('',#7966,.T.);
#5810=FACE_OUTER_BOUND('',#7967,.T.);
#5811=FACE_OUTER_BOUND('',#7968,.T.);
#5812=FACE_OUTER_BOUND('',#7969,.T.);
#5813=FACE_OUTER_BOUND('',#7970,.T.);
#5814=FACE_OUTER_BOUND('',#7971,.T.);
#5815=FACE_OUTER_BOUND('',#7972,.T.);
#5816=FACE_OUTER_BOUND('',#7973,.T.);
#5817=FACE_OUTER_BOUND('',#7974,.T.);
#5818=FACE_OUTER_BOUND('',#7975,.T.);
#5819=FACE_OUTER_BOUND('',#7976,.T.);
#5820=FACE_OUTER_BOUND('',#7977,.T.);
#5821=FACE_OUTER_BOUND('',#7978,.T.);
#5822=FACE_OUTER_BOUND('',#7979,.T.);
#5823=FACE_OUTER_BOUND('',#7980,.T.);
#5824=FACE_OUTER_BOUND('',#7981,.T.);
#5825=FACE_OUTER_BOUND('',#7982,.T.);
#5826=FACE_OUTER_BOUND('',#7984,.T.);
#5827=FACE_OUTER_BOUND('',#7986,.T.);
#5828=FACE_OUTER_BOUND('',#7987,.T.);
#5829=FACE_OUTER_BOUND('',#7988,.T.);
#5830=FACE_OUTER_BOUND('',#7993,.T.);
#5831=FACE_OUTER_BOUND('',#7994,.T.);
#5832=FACE_OUTER_BOUND('',#7995,.T.);
#5833=FACE_OUTER_BOUND('',#7996,.T.);
#5834=FACE_OUTER_BOUND('',#7997,.T.);
#5835=FACE_OUTER_BOUND('',#7998,.T.);
#5836=FACE_OUTER_BOUND('',#7999,.T.);
#5837=FACE_OUTER_BOUND('',#8000,.T.);
#5838=FACE_OUTER_BOUND('',#8006,.T.);
#5839=FACE_OUTER_BOUND('',#8007,.T.);
#5840=FACE_OUTER_BOUND('',#8008,.T.);
#5841=FACE_OUTER_BOUND('',#8009,.T.);
#5842=FACE_OUTER_BOUND('',#8010,.T.);
#5843=FACE_OUTER_BOUND('',#8011,.T.);
#5844=FACE_OUTER_BOUND('',#8012,.T.);
#5845=FACE_OUTER_BOUND('',#8013,.T.);
#5846=FACE_OUTER_BOUND('',#8014,.T.);
#5847=FACE_OUTER_BOUND('',#8015,.T.);
#5848=FACE_OUTER_BOUND('',#8016,.T.);
#5849=FACE_OUTER_BOUND('',#8017,.T.);
#5850=FACE_OUTER_BOUND('',#8023,.T.);
#5851=FACE_OUTER_BOUND('',#8025,.T.);
#5852=FACE_OUTER_BOUND('',#8026,.T.);
#5853=FACE_OUTER_BOUND('',#8028,.T.);
#5854=FACE_OUTER_BOUND('',#8029,.T.);
#5855=FACE_OUTER_BOUND('',#8030,.T.);
#5856=FACE_OUTER_BOUND('',#8032,.T.);
#5857=FACE_OUTER_BOUND('',#8033,.T.);
#5858=FACE_OUTER_BOUND('',#8035,.T.);
#5859=FACE_OUTER_BOUND('',#8038,.T.);
#5860=FACE_OUTER_BOUND('',#8039,.T.);
#5861=FACE_OUTER_BOUND('',#8042,.T.);
#5862=FACE_OUTER_BOUND('',#8043,.T.);
#5863=FACE_OUTER_BOUND('',#8044,.T.);
#5864=FACE_OUTER_BOUND('',#8045,.T.);
#5865=FACE_OUTER_BOUND('',#8046,.T.);
#5866=FACE_OUTER_BOUND('',#8047,.T.);
#5867=FACE_OUTER_BOUND('',#8048,.T.);
#5868=FACE_OUTER_BOUND('',#8049,.T.);
#5869=FACE_OUTER_BOUND('',#8050,.T.);
#5870=FACE_OUTER_BOUND('',#8051,.T.);
#5871=FACE_OUTER_BOUND('',#8052,.T.);
#5872=FACE_OUTER_BOUND('',#8053,.T.);
#5873=FACE_OUTER_BOUND('',#8054,.T.);
#5874=FACE_OUTER_BOUND('',#8055,.T.);
#5875=FACE_OUTER_BOUND('',#8056,.T.);
#5876=FACE_OUTER_BOUND('',#8058,.T.);
#5877=FACE_OUTER_BOUND('',#8059,.T.);
#5878=FACE_OUTER_BOUND('',#8060,.T.);
#5879=FACE_OUTER_BOUND('',#8061,.T.);
#5880=FACE_OUTER_BOUND('',#8062,.T.);
#5881=FACE_OUTER_BOUND('',#8064,.T.);
#5882=FACE_OUTER_BOUND('',#8065,.T.);
#5883=FACE_OUTER_BOUND('',#8066,.T.);
#5884=FACE_OUTER_BOUND('',#8067,.T.);
#5885=FACE_OUTER_BOUND('',#8068,.T.);
#5886=FACE_OUTER_BOUND('',#8069,.T.);
#5887=FACE_OUTER_BOUND('',#8070,.T.);
#5888=FACE_OUTER_BOUND('',#8071,.T.);
#5889=FACE_OUTER_BOUND('',#8072,.T.);
#5890=FACE_OUTER_BOUND('',#8073,.T.);
#5891=FACE_OUTER_BOUND('',#8074,.T.);
#5892=FACE_OUTER_BOUND('',#8075,.T.);
#5893=FACE_OUTER_BOUND('',#8076,.T.);
#5894=FACE_OUTER_BOUND('',#8077,.T.);
#5895=FACE_OUTER_BOUND('',#8078,.T.);
#5896=FACE_OUTER_BOUND('',#8079,.T.);
#5897=FACE_OUTER_BOUND('',#8081,.T.);
#5898=FACE_OUTER_BOUND('',#8082,.T.);
#5899=FACE_OUTER_BOUND('',#8083,.T.);
#5900=FACE_OUTER_BOUND('',#8084,.T.);
#5901=FACE_OUTER_BOUND('',#8085,.T.);
#5902=FACE_OUTER_BOUND('',#8087,.T.);
#5903=FACE_OUTER_BOUND('',#8088,.T.);
#5904=FACE_OUTER_BOUND('',#8089,.T.);
#5905=FACE_OUTER_BOUND('',#8090,.T.);
#5906=FACE_OUTER_BOUND('',#8091,.T.);
#5907=FACE_OUTER_BOUND('',#8092,.T.);
#5908=FACE_OUTER_BOUND('',#8093,.T.);
#5909=FACE_OUTER_BOUND('',#8094,.T.);
#5910=FACE_OUTER_BOUND('',#8095,.T.);
#5911=FACE_OUTER_BOUND('',#8096,.T.);
#5912=FACE_OUTER_BOUND('',#8099,.T.);
#5913=FACE_OUTER_BOUND('',#8100,.T.);
#5914=FACE_OUTER_BOUND('',#8101,.T.);
#5915=FACE_OUTER_BOUND('',#8102,.T.);
#5916=FACE_OUTER_BOUND('',#8103,.T.);
#5917=FACE_OUTER_BOUND('',#8106,.T.);
#5918=FACE_OUTER_BOUND('',#8108,.T.);
#5919=FACE_OUTER_BOUND('',#8110,.T.);
#5920=FACE_OUTER_BOUND('',#8111,.T.);
#5921=FACE_OUTER_BOUND('',#8112,.T.);
#5922=FACE_OUTER_BOUND('',#8114,.T.);
#5923=FACE_OUTER_BOUND('',#8116,.T.);
#5924=FACE_OUTER_BOUND('',#8117,.T.);
#5925=FACE_OUTER_BOUND('',#8118,.T.);
#5926=FACE_OUTER_BOUND('',#8119,.T.);
#5927=FACE_OUTER_BOUND('',#8120,.T.);
#5928=FACE_OUTER_BOUND('',#8121,.T.);
#5929=FACE_OUTER_BOUND('',#8122,.T.);
#5930=FACE_OUTER_BOUND('',#8123,.T.);
#5931=FACE_OUTER_BOUND('',#8124,.T.);
#5932=FACE_OUTER_BOUND('',#8125,.T.);
#5933=FACE_OUTER_BOUND('',#8126,.T.);
#5934=FACE_OUTER_BOUND('',#8127,.T.);
#5935=FACE_OUTER_BOUND('',#8128,.T.);
#5936=FACE_OUTER_BOUND('',#8129,.T.);
#5937=FACE_OUTER_BOUND('',#8130,.T.);
#5938=FACE_OUTER_BOUND('',#8131,.T.);
#5939=FACE_OUTER_BOUND('',#8132,.T.);
#5940=FACE_OUTER_BOUND('',#8133,.T.);
#5941=FACE_OUTER_BOUND('',#8134,.T.);
#5942=FACE_OUTER_BOUND('',#8135,.T.);
#5943=FACE_OUTER_BOUND('',#8136,.T.);
#5944=FACE_OUTER_BOUND('',#8137,.T.);
#5945=FACE_OUTER_BOUND('',#8138,.T.);
#5946=FACE_OUTER_BOUND('',#8139,.T.);
#5947=FACE_OUTER_BOUND('',#8140,.T.);
#5948=FACE_OUTER_BOUND('',#8141,.T.);
#5949=FACE_OUTER_BOUND('',#8142,.T.);
#5950=FACE_OUTER_BOUND('',#8143,.T.);
#5951=FACE_OUTER_BOUND('',#8145,.T.);
#5952=FACE_OUTER_BOUND('',#8147,.T.);
#5953=FACE_OUTER_BOUND('',#8149,.T.);
#5954=FACE_OUTER_BOUND('',#8150,.T.);
#5955=FACE_OUTER_BOUND('',#8151,.T.);
#5956=FACE_OUTER_BOUND('',#8152,.T.);
#5957=FACE_OUTER_BOUND('',#8153,.T.);
#5958=FACE_OUTER_BOUND('',#8154,.T.);
#5959=FACE_OUTER_BOUND('',#8155,.T.);
#5960=FACE_OUTER_BOUND('',#8156,.T.);
#5961=FACE_OUTER_BOUND('',#8157,.T.);
#5962=FACE_OUTER_BOUND('',#8158,.T.);
#5963=FACE_OUTER_BOUND('',#8159,.T.);
#5964=FACE_OUTER_BOUND('',#8160,.T.);
#5965=FACE_OUTER_BOUND('',#8161,.T.);
#5966=FACE_OUTER_BOUND('',#8162,.T.);
#5967=FACE_OUTER_BOUND('',#8163,.T.);
#5968=FACE_OUTER_BOUND('',#8164,.T.);
#5969=FACE_OUTER_BOUND('',#8165,.T.);
#5970=FACE_OUTER_BOUND('',#8166,.T.);
#5971=FACE_OUTER_BOUND('',#8167,.T.);
#5972=FACE_OUTER_BOUND('',#8168,.T.);
#5973=FACE_OUTER_BOUND('',#8169,.T.);
#5974=FACE_OUTER_BOUND('',#8170,.T.);
#5975=FACE_OUTER_BOUND('',#8171,.T.);
#5976=FACE_OUTER_BOUND('',#8172,.T.);
#5977=FACE_OUTER_BOUND('',#8173,.T.);
#5978=FACE_OUTER_BOUND('',#8174,.T.);
#5979=FACE_OUTER_BOUND('',#8175,.T.);
#5980=FACE_OUTER_BOUND('',#8176,.T.);
#5981=FACE_OUTER_BOUND('',#8177,.T.);
#5982=FACE_OUTER_BOUND('',#8178,.T.);
#5983=FACE_OUTER_BOUND('',#8179,.T.);
#5984=FACE_OUTER_BOUND('',#8180,.T.);
#5985=FACE_OUTER_BOUND('',#8181,.T.);
#5986=FACE_OUTER_BOUND('',#8182,.T.);
#5987=FACE_OUTER_BOUND('',#8183,.T.);
#5988=FACE_OUTER_BOUND('',#8184,.T.);
#5989=FACE_OUTER_BOUND('',#8185,.T.);
#5990=FACE_OUTER_BOUND('',#8186,.T.);
#5991=FACE_OUTER_BOUND('',#8187,.T.);
#5992=FACE_OUTER_BOUND('',#8188,.T.);
#5993=FACE_OUTER_BOUND('',#8189,.T.);
#5994=FACE_OUTER_BOUND('',#8190,.T.);
#5995=FACE_OUTER_BOUND('',#8191,.T.);
#5996=FACE_OUTER_BOUND('',#8192,.T.);
#5997=FACE_OUTER_BOUND('',#8193,.T.);
#5998=FACE_OUTER_BOUND('',#8195,.T.);
#5999=FACE_OUTER_BOUND('',#8197,.T.);
#6000=FACE_OUTER_BOUND('',#8199,.T.);
#6001=FACE_OUTER_BOUND('',#8200,.T.);
#6002=FACE_OUTER_BOUND('',#8201,.T.);
#6003=FACE_OUTER_BOUND('',#8202,.T.);
#6004=FACE_OUTER_BOUND('',#8203,.T.);
#6005=FACE_OUTER_BOUND('',#8204,.T.);
#6006=FACE_OUTER_BOUND('',#8205,.T.);
#6007=FACE_OUTER_BOUND('',#8206,.T.);
#6008=FACE_OUTER_BOUND('',#8207,.T.);
#6009=FACE_OUTER_BOUND('',#8208,.T.);
#6010=FACE_OUTER_BOUND('',#8209,.T.);
#6011=FACE_OUTER_BOUND('',#8210,.T.);
#6012=FACE_OUTER_BOUND('',#8211,.T.);
#6013=FACE_OUTER_BOUND('',#8212,.T.);
#6014=FACE_OUTER_BOUND('',#8214,.T.);
#6015=FACE_OUTER_BOUND('',#8215,.T.);
#6016=FACE_OUTER_BOUND('',#8216,.T.);
#6017=FACE_OUTER_BOUND('',#8217,.T.);
#6018=FACE_OUTER_BOUND('',#8218,.T.);
#6019=FACE_OUTER_BOUND('',#8219,.T.);
#6020=FACE_OUTER_BOUND('',#8220,.T.);
#6021=FACE_OUTER_BOUND('',#8221,.T.);
#6022=FACE_OUTER_BOUND('',#8222,.T.);
#6023=FACE_OUTER_BOUND('',#8223,.T.);
#6024=FACE_OUTER_BOUND('',#8224,.T.);
#6025=FACE_OUTER_BOUND('',#8225,.T.);
#6026=FACE_OUTER_BOUND('',#8226,.T.);
#6027=FACE_OUTER_BOUND('',#8228,.T.);
#6028=FACE_OUTER_BOUND('',#8229,.T.);
#6029=FACE_OUTER_BOUND('',#8230,.T.);
#6030=FACE_OUTER_BOUND('',#8231,.T.);
#6031=FACE_OUTER_BOUND('',#8232,.T.);
#6032=FACE_OUTER_BOUND('',#8233,.T.);
#6033=FACE_OUTER_BOUND('',#8234,.T.);
#6034=FACE_OUTER_BOUND('',#8235,.T.);
#6035=FACE_OUTER_BOUND('',#8236,.T.);
#6036=FACE_OUTER_BOUND('',#8237,.T.);
#6037=FACE_OUTER_BOUND('',#8238,.T.);
#6038=FACE_OUTER_BOUND('',#8239,.T.);
#6039=FACE_OUTER_BOUND('',#8240,.T.);
#6040=FACE_OUTER_BOUND('',#8241,.T.);
#6041=FACE_OUTER_BOUND('',#8242,.T.);
#6042=FACE_OUTER_BOUND('',#8243,.T.);
#6043=FACE_OUTER_BOUND('',#8244,.T.);
#6044=FACE_OUTER_BOUND('',#8245,.T.);
#6045=FACE_OUTER_BOUND('',#8246,.T.);
#6046=FACE_OUTER_BOUND('',#8247,.T.);
#6047=FACE_OUTER_BOUND('',#8248,.T.);
#6048=FACE_OUTER_BOUND('',#8249,.T.);
#6049=FACE_OUTER_BOUND('',#8250,.T.);
#6050=FACE_OUTER_BOUND('',#8251,.T.);
#6051=FACE_OUTER_BOUND('',#8252,.T.);
#6052=FACE_OUTER_BOUND('',#8253,.T.);
#6053=FACE_OUTER_BOUND('',#8254,.T.);
#6054=FACE_OUTER_BOUND('',#8255,.T.);
#6055=FACE_OUTER_BOUND('',#8256,.T.);
#6056=FACE_OUTER_BOUND('',#8257,.T.);
#6057=FACE_OUTER_BOUND('',#8258,.T.);
#6058=FACE_OUTER_BOUND('',#8259,.T.);
#6059=FACE_OUTER_BOUND('',#8260,.T.);
#6060=FACE_OUTER_BOUND('',#8261,.T.);
#6061=FACE_OUTER_BOUND('',#8262,.T.);
#6062=FACE_OUTER_BOUND('',#8263,.T.);
#6063=FACE_OUTER_BOUND('',#8264,.T.);
#6064=FACE_OUTER_BOUND('',#8265,.T.);
#6065=FACE_OUTER_BOUND('',#8266,.T.);
#6066=FACE_OUTER_BOUND('',#8267,.T.);
#6067=FACE_OUTER_BOUND('',#8268,.T.);
#6068=FACE_OUTER_BOUND('',#8269,.T.);
#6069=FACE_OUTER_BOUND('',#8270,.T.);
#6070=FACE_OUTER_BOUND('',#8271,.T.);
#6071=FACE_OUTER_BOUND('',#8272,.T.);
#6072=FACE_OUTER_BOUND('',#8273,.T.);
#6073=FACE_OUTER_BOUND('',#8274,.T.);
#6074=FACE_OUTER_BOUND('',#8275,.T.);
#6075=FACE_OUTER_BOUND('',#8283,.T.);
#6076=FACE_OUTER_BOUND('',#8284,.T.);
#6077=FACE_OUTER_BOUND('',#8285,.T.);
#6078=FACE_OUTER_BOUND('',#8286,.T.);
#6079=FACE_OUTER_BOUND('',#8287,.T.);
#6080=FACE_OUTER_BOUND('',#8288,.T.);
#6081=FACE_OUTER_BOUND('',#8304,.T.);
#6082=FACE_OUTER_BOUND('',#8305,.T.);
#6083=FACE_OUTER_BOUND('',#8306,.T.);
#6084=FACE_OUTER_BOUND('',#8307,.T.);
#6085=FACE_OUTER_BOUND('',#8309,.T.);
#6086=FACE_OUTER_BOUND('',#8310,.T.);
#6087=FACE_OUTER_BOUND('',#8311,.T.);
#6088=FACE_OUTER_BOUND('',#8312,.T.);
#6089=FACE_OUTER_BOUND('',#8313,.T.);
#6090=FACE_OUTER_BOUND('',#8314,.T.);
#6091=FACE_OUTER_BOUND('',#8315,.T.);
#6092=FACE_OUTER_BOUND('',#8316,.T.);
#6093=FACE_OUTER_BOUND('',#8317,.T.);
#6094=FACE_OUTER_BOUND('',#8318,.T.);
#6095=FACE_OUTER_BOUND('',#8319,.T.);
#7781=EDGE_LOOP('',(#28770,#28771,#28772,#28773,#28774));
#7782=EDGE_LOOP('',(#28775));
#7783=EDGE_LOOP('',(#28776,#28777,#28778,#28779));
#7784=EDGE_LOOP('',(#28780,#28781,#28782,#28783,#28784,#28785));
#7785=EDGE_LOOP('',(#28786,#28787,#28788,#28789));
#7786=EDGE_LOOP('',(#28790));
#7787=EDGE_LOOP('',(#28791));
#7788=EDGE_LOOP('',(#28792));
#7789=EDGE_LOOP('',(#28793));
#7790=EDGE_LOOP('',(#28794,#28795,#28796,#28797));
#7791=EDGE_LOOP('',(#28798,#28799,#28800,#28801,#28802));
#7792=EDGE_LOOP('',(#28803));
#7793=EDGE_LOOP('',(#28804,#28805,#28806,#28807));
#7794=EDGE_LOOP('',(#28808,#28809,#28810,#28811,#28812,#28813));
#7795=EDGE_LOOP('',(#28814,#28815,#28816,#28817));
#7796=EDGE_LOOP('',(#28818));
#7797=EDGE_LOOP('',(#28819));
#7798=EDGE_LOOP('',(#28820));
#7799=EDGE_LOOP('',(#28821));
#7800=EDGE_LOOP('',(#28822,#28823,#28824,#28825));
#7801=EDGE_LOOP('',(#28826,#28827,#28828,#28829,#28830));
#7802=EDGE_LOOP('',(#28831));
#7803=EDGE_LOOP('',(#28832,#28833,#28834,#28835,#28836,#28837));
#7804=EDGE_LOOP('',(#28838,#28839,#28840,#28841));
#7805=EDGE_LOOP('',(#28842,#28843,#28844,#28845));
#7806=EDGE_LOOP('',(#28846));
#7807=EDGE_LOOP('',(#28847));
#7808=EDGE_LOOP('',(#28848,#28849,#28850,#28851));
#7809=EDGE_LOOP('',(#28852));
#7810=EDGE_LOOP('',(#28853));
#7811=EDGE_LOOP('',(#28854,#28855,#28856,#28857));
#7812=EDGE_LOOP('',(#28858));
#7813=EDGE_LOOP('',(#28859));
#7814=EDGE_LOOP('',(#28860,#28861,#28862,#28863));
#7815=EDGE_LOOP('',(#28864));
#7816=EDGE_LOOP('',(#28865));
#7817=EDGE_LOOP('',(#28866,#28867,#28868,#28869,#28870));
#7818=EDGE_LOOP('',(#28871));
#7819=EDGE_LOOP('',(#28872,#28873,#28874,#28875,#28876,#28877));
#7820=EDGE_LOOP('',(#28878,#28879,#28880,#28881));
#7821=EDGE_LOOP('',(#28882,#28883,#28884,#28885));
#7822=EDGE_LOOP('',(#28886));
#7823=EDGE_LOOP('',(#28887));
#7824=EDGE_LOOP('',(#28888,#28889,#28890,#28891));
#7825=EDGE_LOOP('',(#28892));
#7826=EDGE_LOOP('',(#28893));
#7827=EDGE_LOOP('',(#28894,#28895,#28896,#28897,#28898));
#7828=EDGE_LOOP('',(#28899));
#7829=EDGE_LOOP('',(#28900,#28901,#28902,#28903,#28904,#28905));
#7830=EDGE_LOOP('',(#28906,#28907,#28908,#28909));
#7831=EDGE_LOOP('',(#28910,#28911,#28912,#28913,#28914,#28915,#28916,#28917,
#28918,#28919,#28920,#28921,#28922,#28923,#28924,#28925));
#7832=EDGE_LOOP('',(#28926,#28927,#28928,#28929));
#7833=EDGE_LOOP('',(#28930,#28931,#28932,#28933));
#7834=EDGE_LOOP('',(#28934,#28935,#28936,#28937));
#7835=EDGE_LOOP('',(#28938,#28939,#28940,#28941,#28942,#28943));
#7836=EDGE_LOOP('',(#28944,#28945,#28946,#28947,#28948,#28949));
#7837=EDGE_LOOP('',(#28950,#28951,#28952,#28953,#28954,#28955,#28956,#28957));
#7838=EDGE_LOOP('',(#28958,#28959,#28960,#28961,#28962,#28963,#28964,#28965));
#7839=EDGE_LOOP('',(#28966,#28967,#28968,#28969));
#7840=EDGE_LOOP('',(#28970,#28971,#28972,#28973,#28974,#28975,#28976,#28977,
#28978,#28979,#28980,#28981,#28982,#28983,#28984,#28985));
#7841=EDGE_LOOP('',(#28986));
#7842=EDGE_LOOP('',(#28987,#28988,#28989,#28990,#28991));
#7843=EDGE_LOOP('',(#28992,#28993,#28994,#28995));
#7844=EDGE_LOOP('',(#28996,#28997,#28998,#28999,#29000,#29001,#29002,#29003,
#29004));
#7845=EDGE_LOOP('',(#29005));
#7846=EDGE_LOOP('',(#29006));
#7847=EDGE_LOOP('',(#29007));
#7848=EDGE_LOOP('',(#29008));
#7849=EDGE_LOOP('',(#29009,#29010,#29011,#29012,#29013));
#7850=EDGE_LOOP('',(#29014,#29015,#29016,#29017));
#7851=EDGE_LOOP('',(#29018,#29019,#29020,#29021,#29022,#29023,#29024,#29025,
#29026,#29027,#29028));
#7852=EDGE_LOOP('',(#29029,#29030,#29031,#29032,#29033));
#7853=EDGE_LOOP('',(#29034,#29035,#29036,#29037));
#7854=EDGE_LOOP('',(#29038,#29039,#29040,#29041));
#7855=EDGE_LOOP('',(#29042,#29043,#29044,#29045,#29046));
#7856=EDGE_LOOP('',(#29047,#29048,#29049,#29050,#29051,#29052,#29053,#29054,
#29055,#29056,#29057));
#7857=EDGE_LOOP('',(#29058,#29059,#29060,#29061,#29062,#29063,#29064,#29065,
#29066,#29067,#29068,#29069,#29070,#29071,#29072,#29073,#29074,#29075));
#7858=EDGE_LOOP('',(#29076,#29077,#29078,#29079,#29080,#29081,#29082,#29083,
#29084,#29085));
#7859=EDGE_LOOP('',(#29086,#29087,#29088,#29089,#29090,#29091,#29092,#29093,
#29094));
#7860=EDGE_LOOP('',(#29095,#29096,#29097));
#7861=EDGE_LOOP('',(#29098,#29099,#29100));
#7862=EDGE_LOOP('',(#29101,#29102,#29103,#29104));
#7863=EDGE_LOOP('',(#29105,#29106,#29107,#29108));
#7864=EDGE_LOOP('',(#29109,#29110,#29111,#29112));
#7865=EDGE_LOOP('',(#29113,#29114,#29115));
#7866=EDGE_LOOP('',(#29116,#29117,#29118,#29119,#29120));
#7867=EDGE_LOOP('',(#29121,#29122));
#7868=EDGE_LOOP('',(#29123));
#7869=EDGE_LOOP('',(#29124,#29125,#29126,#29127,#29128));
#7870=EDGE_LOOP('',(#29129,#29130,#29131,#29132,#29133));
#7871=EDGE_LOOP('',(#29134,#29135,#29136,#29137,#29138));
#7872=EDGE_LOOP('',(#29139,#29140,#29141,#29142,#29143));
#7873=EDGE_LOOP('',(#29144,#29145,#29146,#29147,#29148,#29149,#29150));
#7874=EDGE_LOOP('',(#29151,#29152,#29153,#29154,#29155,#29156));
#7875=EDGE_LOOP('',(#29157,#29158,#29159,#29160,#29161,#29162));
#7876=EDGE_LOOP('',(#29163,#29164,#29165));
#7877=EDGE_LOOP('',(#29166,#29167,#29168,#29169,#29170,#29171));
#7878=EDGE_LOOP('',(#29172,#29173,#29174,#29175));
#7879=EDGE_LOOP('',(#29176,#29177,#29178,#29179));
#7880=EDGE_LOOP('',(#29180));
#7881=EDGE_LOOP('',(#29181,#29182,#29183,#29184,#29185,#29186));
#7882=EDGE_LOOP('',(#29187,#29188,#29189,#29190,#29191,#29192));
#7883=EDGE_LOOP('',(#29193,#29194,#29195,#29196,#29197,#29198));
#7884=EDGE_LOOP('',(#29199,#29200,#29201,#29202,#29203,#29204));
#7885=EDGE_LOOP('',(#29205,#29206,#29207));
#7886=EDGE_LOOP('',(#29208,#29209,#29210));
#7887=EDGE_LOOP('',(#29211,#29212,#29213));
#7888=EDGE_LOOP('',(#29214,#29215,#29216));
#7889=EDGE_LOOP('',(#29217,#29218,#29219));
#7890=EDGE_LOOP('',(#29220,#29221,#29222,#29223,#29224,#29225));
#7891=EDGE_LOOP('',(#29226,#29227,#29228,#29229,#29230,#29231));
#7892=EDGE_LOOP('',(#29232,#29233,#29234));
#7893=EDGE_LOOP('',(#29235,#29236,#29237,#29238,#29239,#29240,#29241,#29242,
#29243,#29244,#29245,#29246));
#7894=EDGE_LOOP('',(#29247,#29248,#29249,#29250,#29251,#29252));
#7895=EDGE_LOOP('',(#29253,#29254,#29255,#29256,#29257,#29258));
#7896=EDGE_LOOP('',(#29259,#29260,#29261,#29262,#29263,#29264));
#7897=EDGE_LOOP('',(#29265,#29266,#29267,#29268,#29269,#29270));
#7898=EDGE_LOOP('',(#29271,#29272,#29273));
#7899=EDGE_LOOP('',(#29274,#29275,#29276));
#7900=EDGE_LOOP('',(#29277,#29278,#29279));
#7901=EDGE_LOOP('',(#29280,#29281,#29282));
#7902=EDGE_LOOP('',(#29283,#29284,#29285));
#7903=EDGE_LOOP('',(#29286,#29287,#29288,#29289,#29290,#29291));
#7904=EDGE_LOOP('',(#29292,#29293,#29294,#29295,#29296,#29297));
#7905=EDGE_LOOP('',(#29298,#29299,#29300));
#7906=EDGE_LOOP('',(#29301,#29302,#29303,#29304,#29305,#29306,#29307,#29308,
#29309,#29310,#29311,#29312));
#7907=EDGE_LOOP('',(#29313,#29314,#29315,#29316,#29317));
#7908=EDGE_LOOP('',(#29318,#29319,#29320,#29321));
#7909=EDGE_LOOP('',(#29322,#29323,#29324,#29325));
#7910=EDGE_LOOP('',(#29326,#29327,#29328,#29329));
#7911=EDGE_LOOP('',(#29330,#29331,#29332,#29333));
#7912=EDGE_LOOP('',(#29334,#29335,#29336,#29337));
#7913=EDGE_LOOP('',(#29338,#29339,#29340,#29341));
#7914=EDGE_LOOP('',(#29342,#29343,#29344,#29345));
#7915=EDGE_LOOP('',(#29346,#29347,#29348,#29349));
#7916=EDGE_LOOP('',(#29350,#29351,#29352,#29353));
#7917=EDGE_LOOP('',(#29354,#29355));
#7918=EDGE_LOOP('',(#29356,#29357));
#7919=EDGE_LOOP('',(#29358,#29359,#29360,#29361,#29362,#29363));
#7920=EDGE_LOOP('',(#29364,#29365,#29366,#29367));
#7921=EDGE_LOOP('',(#29368,#29369,#29370,#29371));
#7922=EDGE_LOOP('',(#29372,#29373,#29374,#29375));
#7923=EDGE_LOOP('',(#29376,#29377,#29378,#29379));
#7924=EDGE_LOOP('',(#29380,#29381,#29382,#29383));
#7925=EDGE_LOOP('',(#29384,#29385,#29386,#29387));
#7926=EDGE_LOOP('',(#29388,#29389));
#7927=EDGE_LOOP('',(#29390,#29391));
#7928=EDGE_LOOP('',(#29392,#29393,#29394,#29395,#29396,#29397));
#7929=EDGE_LOOP('',(#29398,#29399,#29400,#29401,#29402,#29403));
#7930=EDGE_LOOP('',(#29404,#29405,#29406,#29407));
#7931=EDGE_LOOP('',(#29408,#29409,#29410,#29411));
#7932=EDGE_LOOP('',(#29412,#29413,#29414,#29415));
#7933=EDGE_LOOP('',(#29416,#29417,#29418,#29419));
#7934=EDGE_LOOP('',(#29420,#29421,#29422,#29423));
#7935=EDGE_LOOP('',(#29424,#29425,#29426,#29427));
#7936=EDGE_LOOP('',(#29428,#29429));
#7937=EDGE_LOOP('',(#29430,#29431));
#7938=EDGE_LOOP('',(#29432,#29433,#29434,#29435,#29436,#29437));
#7939=EDGE_LOOP('',(#29438,#29439,#29440,#29441));
#7940=EDGE_LOOP('',(#29442,#29443,#29444,#29445));
#7941=EDGE_LOOP('',(#29446,#29447,#29448,#29449));
#7942=EDGE_LOOP('',(#29450));
#7943=EDGE_LOOP('',(#29451,#29452,#29453,#29454,#29455,#29456));
#7944=EDGE_LOOP('',(#29457,#29458,#29459,#29460,#29461,#29462));
#7945=EDGE_LOOP('',(#29463,#29464,#29465,#29466));
#7946=EDGE_LOOP('',(#29467,#29468,#29469,#29470,#29471,#29472));
#7947=EDGE_LOOP('',(#29473,#29474,#29475,#29476,#29477));
#7948=EDGE_LOOP('',(#29478,#29479,#29480,#29481));
#7949=EDGE_LOOP('',(#29482,#29483,#29484,#29485,#29486,#29487));
#7950=EDGE_LOOP('',(#29488,#29489,#29490,#29491,#29492));
#7951=EDGE_LOOP('',(#29493,#29494,#29495,#29496));
#7952=EDGE_LOOP('',(#29497,#29498,#29499,#29500,#29501,#29502));
#7953=EDGE_LOOP('',(#29503,#29504,#29505,#29506,#29507));
#7954=EDGE_LOOP('',(#29508,#29509,#29510,#29511,#29512));
#7955=EDGE_LOOP('',(#29513,#29514,#29515,#29516,#29517,#29518));
#7956=EDGE_LOOP('',(#29519,#29520,#29521,#29522));
#7957=EDGE_LOOP('',(#29523,#29524,#29525,#29526,#29527));
#7958=EDGE_LOOP('',(#29528,#29529,#29530,#29531,#29532,#29533));
#7959=EDGE_LOOP('',(#29534,#29535,#29536,#29537));
#7960=EDGE_LOOP('',(#29538,#29539,#29540,#29541,#29542));
#7961=EDGE_LOOP('',(#29543,#29544,#29545,#29546,#29547,#29548));
#7962=EDGE_LOOP('',(#29549,#29550,#29551,#29552));
#7963=EDGE_LOOP('',(#29553,#29554,#29555,#29556,#29557));
#7964=EDGE_LOOP('',(#29558,#29559,#29560,#29561,#29562,#29563));
#7965=EDGE_LOOP('',(#29564,#29565,#29566,#29567));
#7966=EDGE_LOOP('',(#29568,#29569,#29570,#29571));
#7967=EDGE_LOOP('',(#29572,#29573,#29574,#29575));
#7968=EDGE_LOOP('',(#29576,#29577,#29578,#29579));
#7969=EDGE_LOOP('',(#29580,#29581,#29582,#29583));
#7970=EDGE_LOOP('',(#29584,#29585,#29586,#29587));
#7971=EDGE_LOOP('',(#29588,#29589,#29590,#29591));
#7972=EDGE_LOOP('',(#29592,#29593,#29594,#29595));
#7973=EDGE_LOOP('',(#29596,#29597,#29598,#29599));
#7974=EDGE_LOOP('',(#29600,#29601,#29602,#29603));
#7975=EDGE_LOOP('',(#29604,#29605,#29606,#29607));
#7976=EDGE_LOOP('',(#29608,#29609,#29610,#29611));
#7977=EDGE_LOOP('',(#29612,#29613,#29614,#29615));
#7978=EDGE_LOOP('',(#29616,#29617,#29618,#29619));
#7979=EDGE_LOOP('',(#29620,#29621,#29622,#29623,#29624));
#7980=EDGE_LOOP('',(#29625,#29626,#29627,#29628));
#7981=EDGE_LOOP('',(#29629,#29630,#29631,#29632));
#7982=EDGE_LOOP('',(#29633,#29634,#29635,#29636,#29637,#29638,#29639,#29640,
#29641,#29642));
#7983=EDGE_LOOP('',(#29643,#29644,#29645,#29646,#29647,#29648,#29649,#29650));
#7984=EDGE_LOOP('',(#29651));
#7985=EDGE_LOOP('',(#29652));
#7986=EDGE_LOOP('',(#29653,#29654,#29655,#29656));
#7987=EDGE_LOOP('',(#29657,#29658,#29659,#29660,#29661));
#7988=EDGE_LOOP('',(#29662,#29663,#29664,#29665,#29666,#29667,#29668,#29669,
#29670,#29671,#29672,#29673,#29674,#29675,#29676,#29677));
#7989=EDGE_LOOP('',(#29678));
#7990=EDGE_LOOP('',(#29679));
#7991=EDGE_LOOP('',(#29680));
#7992=EDGE_LOOP('',(#29681));
#7993=EDGE_LOOP('',(#29682,#29683,#29684,#29685,#29686));
#7994=EDGE_LOOP('',(#29687,#29688,#29689,#29690));
#7995=EDGE_LOOP('',(#29691,#29692,#29693,#29694));
#7996=EDGE_LOOP('',(#29695,#29696,#29697,#29698));
#7997=EDGE_LOOP('',(#29699,#29700,#29701,#29702));
#7998=EDGE_LOOP('',(#29703,#29704,#29705,#29706));
#7999=EDGE_LOOP('',(#29707,#29708,#29709,#29710));
#8000=EDGE_LOOP('',(#29711,#29712,#29713,#29714,#29715,#29716,#29717,#29718));
#8001=EDGE_LOOP('',(#29719));
#8002=EDGE_LOOP('',(#29720));
#8003=EDGE_LOOP('',(#29721));
#8004=EDGE_LOOP('',(#29722));
#8005=EDGE_LOOP('',(#29723));
#8006=EDGE_LOOP('',(#29724,#29725,#29726,#29727,#29728));
#8007=EDGE_LOOP('',(#29729,#29730,#29731,#29732));
#8008=EDGE_LOOP('',(#29733,#29734,#29735,#29736));
#8009=EDGE_LOOP('',(#29737,#29738,#29739,#29740,#29741));
#8010=EDGE_LOOP('',(#29742,#29743,#29744,#29745,#29746,#29747));
#8011=EDGE_LOOP('',(#29748,#29749,#29750,#29751,#29752));
#8012=EDGE_LOOP('',(#29753,#29754,#29755,#29756,#29757,#29758,#29759,#29760,
#29761,#29762));
#8013=EDGE_LOOP('',(#29763,#29764,#29765,#29766,#29767));
#8014=EDGE_LOOP('',(#29768,#29769,#29770,#29771,#29772));
#8015=EDGE_LOOP('',(#29773,#29774,#29775,#29776));
#8016=EDGE_LOOP('',(#29777,#29778,#29779,#29780,#29781));
#8017=EDGE_LOOP('',(#29782,#29783,#29784,#29785,#29786,#29787,#29788,#29789));
#8018=EDGE_LOOP('',(#29790,#29791,#29792,#29793,#29794,#29795));
#8019=EDGE_LOOP('',(#29796,#29797,#29798,#29799,#29800,#29801));
#8020=EDGE_LOOP('',(#29802,#29803,#29804,#29805,#29806,#29807));
#8021=EDGE_LOOP('',(#29808,#29809,#29810,#29811,#29812,#29813));
#8022=EDGE_LOOP('',(#29814));
#8023=EDGE_LOOP('',(#29815));
#8024=EDGE_LOOP('',(#29816));
#8025=EDGE_LOOP('',(#29817,#29818,#29819,#29820));
#8026=EDGE_LOOP('',(#29821));
#8027=EDGE_LOOP('',(#29822));
#8028=EDGE_LOOP('',(#29823,#29824,#29825,#29826,#29827));
#8029=EDGE_LOOP('',(#29828,#29829,#29830,#29831,#29832));
#8030=EDGE_LOOP('',(#29833));
#8031=EDGE_LOOP('',(#29834,#29835,#29836,#29837));
#8032=EDGE_LOOP('',(#29838,#29839,#29840,#29841));
#8033=EDGE_LOOP('',(#29842));
#8034=EDGE_LOOP('',(#29843));
#8035=EDGE_LOOP('',(#29844,#29845,#29846,#29847));
#8036=EDGE_LOOP('',(#29848));
#8037=EDGE_LOOP('',(#29849));
#8038=EDGE_LOOP('',(#29850,#29851,#29852,#29853,#29854));
#8039=EDGE_LOOP('',(#29855,#29856,#29857,#29858));
#8040=EDGE_LOOP('',(#29859));
#8041=EDGE_LOOP('',(#29860));
#8042=EDGE_LOOP('',(#29861,#29862,#29863,#29864,#29865,#29866));
#8043=EDGE_LOOP('',(#29867,#29868,#29869,#29870));
#8044=EDGE_LOOP('',(#29871,#29872,#29873,#29874));
#8045=EDGE_LOOP('',(#29875,#29876,#29877,#29878));
#8046=EDGE_LOOP('',(#29879,#29880,#29881,#29882));
#8047=EDGE_LOOP('',(#29883,#29884,#29885,#29886));
#8048=EDGE_LOOP('',(#29887,#29888,#29889,#29890));
#8049=EDGE_LOOP('',(#29891,#29892,#29893,#29894,#29895,#29896));
#8050=EDGE_LOOP('',(#29897,#29898,#29899,#29900));
#8051=EDGE_LOOP('',(#29901,#29902,#29903,#29904));
#8052=EDGE_LOOP('',(#29905,#29906,#29907,#29908));
#8053=EDGE_LOOP('',(#29909,#29910,#29911,#29912));
#8054=EDGE_LOOP('',(#29913,#29914,#29915,#29916));
#8055=EDGE_LOOP('',(#29917,#29918,#29919,#29920));
#8056=EDGE_LOOP('',(#29921));
#8057=EDGE_LOOP('',(#29922,#29923,#29924,#29925,#29926,#29927));
#8058=EDGE_LOOP('',(#29928,#29929,#29930,#29931,#29932));
#8059=EDGE_LOOP('',(#29933,#29934,#29935,#29936,#29937));
#8060=EDGE_LOOP('',(#29938,#29939,#29940,#29941,#29942));
#8061=EDGE_LOOP('',(#29943));
#8062=EDGE_LOOP('',(#29944));
#8063=EDGE_LOOP('',(#29945,#29946,#29947,#29948,#29949,#29950));
#8064=EDGE_LOOP('',(#29951,#29952,#29953,#29954,#29955));
#8065=EDGE_LOOP('',(#29956,#29957,#29958,#29959,#29960,#29961));
#8066=EDGE_LOOP('',(#29962,#29963,#29964,#29965));
#8067=EDGE_LOOP('',(#29966,#29967,#29968,#29969));
#8068=EDGE_LOOP('',(#29970,#29971,#29972,#29973));
#8069=EDGE_LOOP('',(#29974,#29975,#29976,#29977));
#8070=EDGE_LOOP('',(#29978,#29979,#29980,#29981));
#8071=EDGE_LOOP('',(#29982,#29983,#29984,#29985));
#8072=EDGE_LOOP('',(#29986,#29987,#29988,#29989,#29990,#29991));
#8073=EDGE_LOOP('',(#29992,#29993,#29994,#29995));
#8074=EDGE_LOOP('',(#29996,#29997,#29998,#29999));
#8075=EDGE_LOOP('',(#30000,#30001,#30002,#30003));
#8076=EDGE_LOOP('',(#30004,#30005,#30006,#30007));
#8077=EDGE_LOOP('',(#30008,#30009,#30010,#30011));
#8078=EDGE_LOOP('',(#30012,#30013,#30014,#30015));
#8079=EDGE_LOOP('',(#30016));
#8080=EDGE_LOOP('',(#30017,#30018,#30019,#30020,#30021,#30022));
#8081=EDGE_LOOP('',(#30023,#30024,#30025,#30026,#30027));
#8082=EDGE_LOOP('',(#30028,#30029,#30030,#30031,#30032));
#8083=EDGE_LOOP('',(#30033,#30034,#30035,#30036,#30037));
#8084=EDGE_LOOP('',(#30038));
#8085=EDGE_LOOP('',(#30039));
#8086=EDGE_LOOP('',(#30040,#30041,#30042,#30043,#30044,#30045));
#8087=EDGE_LOOP('',(#30046,#30047,#30048,#30049,#30050));
#8088=EDGE_LOOP('',(#30051,#30052,#30053,#30054,#30055));
#8089=EDGE_LOOP('',(#30056,#30057,#30058,#30059,#30060));
#8090=EDGE_LOOP('',(#30061));
#8091=EDGE_LOOP('',(#30062,#30063,#30064,#30065,#30066));
#8092=EDGE_LOOP('',(#30067,#30068,#30069,#30070,#30071));
#8093=EDGE_LOOP('',(#30072));
#8094=EDGE_LOOP('',(#30073,#30074,#30075,#30076,#30077));
#8095=EDGE_LOOP('',(#30078,#30079,#30080,#30081,#30082));
#8096=EDGE_LOOP('',(#30083,#30084,#30085,#30086,#30087));
#8097=EDGE_LOOP('',(#30088));
#8098=EDGE_LOOP('',(#30089));
#8099=EDGE_LOOP('',(#30090,#30091,#30092,#30093,#30094));
#8100=EDGE_LOOP('',(#30095,#30096,#30097,#30098,#30099,#30100));
#8101=EDGE_LOOP('',(#30101,#30102,#30103,#30104));
#8102=EDGE_LOOP('',(#30105,#30106,#30107,#30108,#30109,#30110));
#8103=EDGE_LOOP('',(#30111,#30112,#30113,#30114,#30115));
#8104=EDGE_LOOP('',(#30116));
#8105=EDGE_LOOP('',(#30117));
#8106=EDGE_LOOP('',(#30118));
#8107=EDGE_LOOP('',(#30119));
#8108=EDGE_LOOP('',(#30120));
#8109=EDGE_LOOP('',(#30121));
#8110=EDGE_LOOP('',(#30122,#30123,#30124,#30125,#30126));
#8111=EDGE_LOOP('',(#30127,#30128,#30129,#30130));
#8112=EDGE_LOOP('',(#30131));
#8113=EDGE_LOOP('',(#30132));
#8114=EDGE_LOOP('',(#30133));
#8115=EDGE_LOOP('',(#30134));
#8116=EDGE_LOOP('',(#30135,#30136,#30137,#30138,#30139));
#8117=EDGE_LOOP('',(#30140,#30141,#30142,#30143,#30144,#30145,#30146,#30147,
#30148,#30149,#30150,#30151));
#8118=EDGE_LOOP('',(#30152,#30153,#30154));
#8119=EDGE_LOOP('',(#30155,#30156,#30157,#30158,#30159,#30160));
#8120=EDGE_LOOP('',(#30161,#30162,#30163,#30164,#30165,#30166));
#8121=EDGE_LOOP('',(#30167,#30168,#30169));
#8122=EDGE_LOOP('',(#30170,#30171,#30172));
#8123=EDGE_LOOP('',(#30173,#30174,#30175));
#8124=EDGE_LOOP('',(#30176,#30177,#30178));
#8125=EDGE_LOOP('',(#30179,#30180,#30181));
#8126=EDGE_LOOP('',(#30182,#30183,#30184,#30185,#30186,#30187));
#8127=EDGE_LOOP('',(#30188,#30189,#30190,#30191,#30192,#30193));
#8128=EDGE_LOOP('',(#30194,#30195,#30196,#30197,#30198,#30199));
#8129=EDGE_LOOP('',(#30200,#30201,#30202,#30203,#30204,#30205));
#8130=EDGE_LOOP('',(#30206,#30207,#30208,#30209,#30210,#30211,#30212,#30213,
#30214,#30215,#30216,#30217));
#8131=EDGE_LOOP('',(#30218,#30219,#30220));
#8132=EDGE_LOOP('',(#30221,#30222,#30223,#30224,#30225,#30226));
#8133=EDGE_LOOP('',(#30227,#30228,#30229,#30230,#30231,#30232));
#8134=EDGE_LOOP('',(#30233,#30234,#30235));
#8135=EDGE_LOOP('',(#30236,#30237,#30238));
#8136=EDGE_LOOP('',(#30239,#30240,#30241));
#8137=EDGE_LOOP('',(#30242,#30243,#30244));
#8138=EDGE_LOOP('',(#30245,#30246,#30247));
#8139=EDGE_LOOP('',(#30248,#30249,#30250,#30251,#30252,#30253));
#8140=EDGE_LOOP('',(#30254,#30255,#30256,#30257,#30258,#30259));
#8141=EDGE_LOOP('',(#30260,#30261,#30262,#30263,#30264,#30265));
#8142=EDGE_LOOP('',(#30266,#30267,#30268,#30269,#30270,#30271));
#8143=EDGE_LOOP('',(#30272));
#8144=EDGE_LOOP('',(#30273));
#8145=EDGE_LOOP('',(#30274));
#8146=EDGE_LOOP('',(#30275));
#8147=EDGE_LOOP('',(#30276));
#8148=EDGE_LOOP('',(#30277));
#8149=EDGE_LOOP('',(#30278,#30279,#30280,#30281));
#8150=EDGE_LOOP('',(#30282,#30283,#30284,#30285));
#8151=EDGE_LOOP('',(#30286,#30287,#30288,#30289));
#8152=EDGE_LOOP('',(#30290,#30291,#30292,#30293));
#8153=EDGE_LOOP('',(#30294,#30295,#30296,#30297));
#8154=EDGE_LOOP('',(#30298,#30299,#30300,#30301));
#8155=EDGE_LOOP('',(#30302,#30303,#30304,#30305));
#8156=EDGE_LOOP('',(#30306,#30307,#30308,#30309,#30310,#30311,#30312,#30313));
#8157=EDGE_LOOP('',(#30314,#30315,#30316,#30317));
#8158=EDGE_LOOP('',(#30318,#30319,#30320,#30321));
#8159=EDGE_LOOP('',(#30322,#30323,#30324,#30325));
#8160=EDGE_LOOP('',(#30326,#30327,#30328,#30329));
#8161=EDGE_LOOP('',(#30330,#30331,#30332,#30333));
#8162=EDGE_LOOP('',(#30334,#30335,#30336,#30337));
#8163=EDGE_LOOP('',(#30338,#30339,#30340,#30341));
#8164=EDGE_LOOP('',(#30342,#30343,#30344,#30345));
#8165=EDGE_LOOP('',(#30346,#30347,#30348,#30349,#30350,#30351,#30352,#30353));
#8166=EDGE_LOOP('',(#30354,#30355,#30356,#30357));
#8167=EDGE_LOOP('',(#30358,#30359,#30360,#30361));
#8168=EDGE_LOOP('',(#30362,#30363,#30364,#30365));
#8169=EDGE_LOOP('',(#30366,#30367,#30368,#30369));
#8170=EDGE_LOOP('',(#30370,#30371,#30372,#30373));
#8171=EDGE_LOOP('',(#30374,#30375,#30376,#30377));
#8172=EDGE_LOOP('',(#30378,#30379,#30380,#30381));
#8173=EDGE_LOOP('',(#30382,#30383,#30384,#30385));
#8174=EDGE_LOOP('',(#30386,#30387,#30388,#30389,#30390,#30391,#30392,#30393));
#8175=EDGE_LOOP('',(#30394,#30395,#30396,#30397));
#8176=EDGE_LOOP('',(#30398,#30399,#30400,#30401));
#8177=EDGE_LOOP('',(#30402,#30403,#30404,#30405));
#8178=EDGE_LOOP('',(#30406,#30407,#30408,#30409));
#8179=EDGE_LOOP('',(#30410,#30411,#30412,#30413));
#8180=EDGE_LOOP('',(#30414,#30415,#30416,#30417));
#8181=EDGE_LOOP('',(#30418,#30419,#30420,#30421));
#8182=EDGE_LOOP('',(#30422,#30423,#30424,#30425));
#8183=EDGE_LOOP('',(#30426,#30427,#30428,#30429,#30430,#30431,#30432,#30433));
#8184=EDGE_LOOP('',(#30434,#30435,#30436,#30437));
#8185=EDGE_LOOP('',(#30438,#30439,#30440,#30441));
#8186=EDGE_LOOP('',(#30442,#30443,#30444,#30445));
#8187=EDGE_LOOP('',(#30446,#30447,#30448,#30449));
#8188=EDGE_LOOP('',(#30450,#30451));
#8189=EDGE_LOOP('',(#30452,#30453,#30454,#30455));
#8190=EDGE_LOOP('',(#30456,#30457));
#8191=EDGE_LOOP('',(#30458,#30459,#30460,#30461));
#8192=EDGE_LOOP('',(#30462,#30463));
#8193=EDGE_LOOP('',(#30464,#30465,#30466,#30467,#30468,#30469));
#8194=EDGE_LOOP('',(#30470));
#8195=EDGE_LOOP('',(#30471,#30472,#30473,#30474,#30475,#30476));
#8196=EDGE_LOOP('',(#30477));
#8197=EDGE_LOOP('',(#30478,#30479,#30480,#30481,#30482,#30483));
#8198=EDGE_LOOP('',(#30484));
#8199=EDGE_LOOP('',(#30485,#30486,#30487,#30488,#30489));
#8200=EDGE_LOOP('',(#30490,#30491,#30492,#30493));
#8201=EDGE_LOOP('',(#30494,#30495,#30496,#30497));
#8202=EDGE_LOOP('',(#30498,#30499,#30500,#30501));
#8203=EDGE_LOOP('',(#30502,#30503,#30504,#30505));
#8204=EDGE_LOOP('',(#30506,#30507,#30508,#30509,#30510,#30511,#30512,#30513,
#30514,#30515,#30516,#30517));
#8205=EDGE_LOOP('',(#30518,#30519,#30520,#30521));
#8206=EDGE_LOOP('',(#30522,#30523,#30524,#30525,#30526,#30527,#30528,#30529,
#30530,#30531,#30532,#30533));
#8207=EDGE_LOOP('',(#30534,#30535,#30536,#30537));
#8208=EDGE_LOOP('',(#30538,#30539,#30540,#30541,#30542,#30543,#30544,#30545,
#30546,#30547,#30548,#30549));
#8209=EDGE_LOOP('',(#30550,#30551,#30552,#30553));
#8210=EDGE_LOOP('',(#30554,#30555,#30556,#30557,#30558,#30559,#30560,#30561,
#30562,#30563,#30564,#30565));
#8211=EDGE_LOOP('',(#30566,#30567,#30568,#30569));
#8212=EDGE_LOOP('',(#30570,#30571,#30572,#30573,#30574,#30575,#30576,#30577,
#30578,#30579,#30580,#30581,#30582,#30583,#30584,#30585));
#8213=EDGE_LOOP('',(#30586));
#8214=EDGE_LOOP('',(#30587,#30588,#30589,#30590));
#8215=EDGE_LOOP('',(#30591,#30592,#30593,#30594));
#8216=EDGE_LOOP('',(#30595,#30596,#30597,#30598));
#8217=EDGE_LOOP('',(#30599,#30600,#30601,#30602));
#8218=EDGE_LOOP('',(#30603,#30604,#30605,#30606));
#8219=EDGE_LOOP('',(#30607,#30608,#30609,#30610));
#8220=EDGE_LOOP('',(#30611,#30612,#30613,#30614));
#8221=EDGE_LOOP('',(#30615,#30616,#30617,#30618));
#8222=EDGE_LOOP('',(#30619,#30620,#30621,#30622));
#8223=EDGE_LOOP('',(#30623,#30624,#30625,#30626));
#8224=EDGE_LOOP('',(#30627,#30628,#30629,#30630));
#8225=EDGE_LOOP('',(#30631,#30632,#30633,#30634));
#8226=EDGE_LOOP('',(#30635,#30636,#30637,#30638,#30639,#30640));
#8227=EDGE_LOOP('',(#30641));
#8228=EDGE_LOOP('',(#30642,#30643,#30644,#30645));
#8229=EDGE_LOOP('',(#30646,#30647));
#8230=EDGE_LOOP('',(#30648,#30649,#30650,#30651));
#8231=EDGE_LOOP('',(#30652,#30653,#30654,#30655));
#8232=EDGE_LOOP('',(#30656,#30657,#30658,#30659));
#8233=EDGE_LOOP('',(#30660,#30661,#30662,#30663));
#8234=EDGE_LOOP('',(#30664,#30665,#30666,#30667));
#8235=EDGE_LOOP('',(#30668,#30669,#30670,#30671));
#8236=EDGE_LOOP('',(#30672,#30673,#30674,#30675));
#8237=EDGE_LOOP('',(#30676,#30677,#30678,#30679));
#8238=EDGE_LOOP('',(#30680,#30681,#30682,#30683,#30684,#30685,#30686,#30687));
#8239=EDGE_LOOP('',(#30688,#30689,#30690,#30691));
#8240=EDGE_LOOP('',(#30692,#30693,#30694,#30695));
#8241=EDGE_LOOP('',(#30696,#30697,#30698,#30699));
#8242=EDGE_LOOP('',(#30700,#30701,#30702,#30703));
#8243=EDGE_LOOP('',(#30704,#30705,#30706,#30707));
#8244=EDGE_LOOP('',(#30708,#30709,#30710,#30711));
#8245=EDGE_LOOP('',(#30712,#30713,#30714,#30715));
#8246=EDGE_LOOP('',(#30716,#30717,#30718,#30719));
#8247=EDGE_LOOP('',(#30720,#30721,#30722,#30723,#30724,#30725,#30726,#30727));
#8248=EDGE_LOOP('',(#30728,#30729,#30730,#30731));
#8249=EDGE_LOOP('',(#30732,#30733,#30734,#30735));
#8250=EDGE_LOOP('',(#30736,#30737,#30738,#30739));
#8251=EDGE_LOOP('',(#30740,#30741,#30742,#30743));
#8252=EDGE_LOOP('',(#30744,#30745,#30746,#30747));
#8253=EDGE_LOOP('',(#30748,#30749,#30750,#30751));
#8254=EDGE_LOOP('',(#30752,#30753,#30754,#30755));
#8255=EDGE_LOOP('',(#30756,#30757,#30758,#30759));
#8256=EDGE_LOOP('',(#30760,#30761,#30762,#30763,#30764,#30765,#30766,#30767));
#8257=EDGE_LOOP('',(#30768,#30769,#30770,#30771));
#8258=EDGE_LOOP('',(#30772,#30773,#30774,#30775));
#8259=EDGE_LOOP('',(#30776,#30777,#30778,#30779));
#8260=EDGE_LOOP('',(#30780,#30781,#30782,#30783));
#8261=EDGE_LOOP('',(#30784,#30785,#30786,#30787));
#8262=EDGE_LOOP('',(#30788,#30789,#30790,#30791));
#8263=EDGE_LOOP('',(#30792,#30793,#30794,#30795));
#8264=EDGE_LOOP('',(#30796,#30797,#30798,#30799));
#8265=EDGE_LOOP('',(#30800,#30801,#30802,#30803,#30804,#30805,#30806,#30807));
#8266=EDGE_LOOP('',(#30808,#30809,#30810,#30811));
#8267=EDGE_LOOP('',(#30812,#30813,#30814,#30815));
#8268=EDGE_LOOP('',(#30816,#30817,#30818,#30819));
#8269=EDGE_LOOP('',(#30820,#30821,#30822,#30823));
#8270=EDGE_LOOP('',(#30824,#30825,#30826,#30827));
#8271=EDGE_LOOP('',(#30828,#30829,#30830,#30831));
#8272=EDGE_LOOP('',(#30832,#30833,#30834,#30835));
#8273=EDGE_LOOP('',(#30836,#30837,#30838,#30839));
#8274=EDGE_LOOP('',(#30840,#30841,#30842,#30843,#30844));
#8275=EDGE_LOOP('',(#30845));
#8276=EDGE_LOOP('',(#30846));
#8277=EDGE_LOOP('',(#30847));
#8278=EDGE_LOOP('',(#30848));
#8279=EDGE_LOOP('',(#30849));
#8280=EDGE_LOOP('',(#30850));
#8281=EDGE_LOOP('',(#30851));
#8282=EDGE_LOOP('',(#30852,#30853,#30854,#30855,#30856,#30857,#30858,#30859));
#8283=EDGE_LOOP('',(#30860,#30861,#30862,#30863));
#8284=EDGE_LOOP('',(#30864,#30865,#30866,#30867));
#8285=EDGE_LOOP('',(#30868,#30869,#30870,#30871,#30872,#30873));
#8286=EDGE_LOOP('',(#30874,#30875,#30876,#30877,#30878,#30879));
#8287=EDGE_LOOP('',(#30880,#30881,#30882,#30883));
#8288=EDGE_LOOP('',(#30884));
#8289=EDGE_LOOP('',(#30885,#30886,#30887,#30888,#30889,#30890,#30891,#30892));
#8290=EDGE_LOOP('',(#30893,#30894,#30895,#30896,#30897,#30898,#30899,#30900,
#30901,#30902,#30903,#30904,#30905,#30906,#30907,#30908));
#8291=EDGE_LOOP('',(#30909));
#8292=EDGE_LOOP('',(#30910));
#8293=EDGE_LOOP('',(#30911));
#8294=EDGE_LOOP('',(#30912));
#8295=EDGE_LOOP('',(#30913));
#8296=EDGE_LOOP('',(#30914));
#8297=EDGE_LOOP('',(#30915,#30916,#30917,#30918,#30919,#30920,#30921,#30922));
#8298=EDGE_LOOP('',(#30923,#30924,#30925,#30926,#30927,#30928,#30929,#30930));
#8299=EDGE_LOOP('',(#30931,#30932,#30933,#30934,#30935,#30936,#30937,#30938));
#8300=EDGE_LOOP('',(#30939,#30940,#30941,#30942,#30943,#30944,#30945,#30946));
#8301=EDGE_LOOP('',(#30947,#30948,#30949,#30950,#30951,#30952,#30953,#30954));
#8302=EDGE_LOOP('',(#30955,#30956,#30957,#30958,#30959,#30960,#30961,#30962));
#8303=EDGE_LOOP('',(#30963,#30964,#30965,#30966,#30967,#30968,#30969,#30970));
#8304=EDGE_LOOP('',(#30971,#30972,#30973,#30974,#30975,#30976));
#8305=EDGE_LOOP('',(#30977,#30978,#30979,#30980,#30981,#30982));
#8306=EDGE_LOOP('',(#30983,#30984,#30985,#30986));
#8307=EDGE_LOOP('',(#30987));
#8308=EDGE_LOOP('',(#30988));
#8309=EDGE_LOOP('',(#30989,#30990,#30991,#30992,#30993));
#8310=EDGE_LOOP('',(#30994,#30995,#30996,#30997,#30998,#30999));
#8311=EDGE_LOOP('',(#31000,#31001,#31002,#31003,#31004));
#8312=EDGE_LOOP('',(#31005,#31006,#31007,#31008));
#8313=EDGE_LOOP('',(#31009,#31010,#31011,#31012));
#8314=EDGE_LOOP('',(#31013,#31014,#31015,#31016));
#8315=EDGE_LOOP('',(#31017,#31018,#31019,#31020));
#8316=EDGE_LOOP('',(#31021,#31022,#31023,#31024));
#8317=EDGE_LOOP('',(#31025,#31026,#31027,#31028,#31029,#31030));
#8318=EDGE_LOOP('',(#31031,#31032,#31033,#31034));
#8319=EDGE_LOOP('',(#31035));
#8320=EDGE_LOOP('',(#31036,#31037,#31038,#31039,#31040,#31041));
#10200=LINE('',#58614,#12747);
#10201=LINE('',#58620,#12748);
#10202=LINE('',#58625,#12749);
#10203=LINE('',#58630,#12750);
#10204=LINE('',#58639,#12751);
#10205=LINE('',#58646,#12752);
#10206=LINE('',#58652,#12753);
#10207=LINE('',#58657,#12754);
#10208=LINE('',#58662,#12755);
#10209=LINE('',#58671,#12756);
#10210=LINE('',#58677,#12757);
#10211=LINE('',#58686,#12758);
#10212=LINE('',#58689,#12759);
#10213=LINE('',#58694,#12760);
#10214=LINE('',#58702,#12761);
#10215=LINE('',#58708,#12762);
#10216=LINE('',#58715,#12763);
#10217=LINE('',#58724,#12764);
#10218=LINE('',#58732,#12765);
#10219=LINE('',#58735,#12766);
#10220=LINE('',#58740,#12767);
#10221=LINE('',#58747,#12768);
#10222=LINE('',#58756,#12769);
#10223=LINE('',#58764,#12770);
#10224=LINE('',#58767,#12771);
#10225=LINE('',#58771,#12772);
#10226=LINE('',#58773,#12773);
#10227=LINE('',#58775,#12774);
#10228=LINE('',#58777,#12775);
#10229=LINE('',#58783,#12776);
#10230=LINE('',#58785,#12777);
#10231=LINE('',#58787,#12778);
#10232=LINE('',#58789,#12779);
#10233=LINE('',#58791,#12780);
#10234=LINE('',#58793,#12781);
#10235=LINE('',#58795,#12782);
#10236=LINE('',#58797,#12783);
#10237=LINE('',#58799,#12784);
#10238=LINE('',#58804,#12785);
#10239=LINE('',#58810,#12786);
#10240=LINE('',#58813,#12787);
#10241=LINE('',#58816,#12788);
#10242=LINE('',#58818,#12789);
#10243=LINE('',#58819,#12790);
#10244=LINE('',#58825,#12791);
#10245=LINE('',#58828,#12792);
#10246=LINE('',#58831,#12793);
#10247=LINE('',#58833,#12794);
#10248=LINE('',#58835,#12795);
#10249=LINE('',#58837,#12796);
#10250=LINE('',#58838,#12797);
#10251=LINE('',#58841,#12798);
#10252=LINE('',#58842,#12799);
#10253=LINE('',#58844,#12800);
#10254=LINE('',#58845,#12801);
#10255=LINE('',#58848,#12802);
#10256=LINE('',#58850,#12803);
#10257=LINE('',#58851,#12804);
#10258=LINE('',#58855,#12805);
#10259=LINE('',#58859,#12806);
#10260=LINE('',#58861,#12807);
#10261=LINE('',#58863,#12808);
#10262=LINE('',#58864,#12809);
#10263=LINE('',#58867,#12810);
#10264=LINE('',#58868,#12811);
#10265=LINE('',#58873,#12812);
#10266=LINE('',#58875,#12813);
#10267=LINE('',#58877,#12814);
#10268=LINE('',#58882,#12815);
#10269=LINE('',#58884,#12816);
#10270=LINE('',#58886,#12817);
#10271=LINE('',#58894,#12818);
#10272=LINE('',#58900,#12819);
#10273=LINE('',#58903,#12820);
#10274=LINE('',#58905,#12821);
#10275=LINE('',#58907,#12822);
#10276=LINE('',#58909,#12823);
#10277=LINE('',#58911,#12824);
#10278=LINE('',#58912,#12825);
#10279=LINE('',#58921,#12826);
#10280=LINE('',#58927,#12827);
#10281=LINE('',#58931,#12828);
#10282=LINE('',#58933,#12829);
#10283=LINE('',#58937,#12830);
#10284=LINE('',#58941,#12831);
#10285=LINE('',#58943,#12832);
#10286=LINE('',#58945,#12833);
#10287=LINE('',#58947,#12834);
#10288=LINE('',#58948,#12835);
#10289=LINE('',#58951,#12836);
#10290=LINE('',#58957,#12837);
#10291=LINE('',#58958,#12838);
#10292=LINE('',#58961,#12839);
#10293=LINE('',#58962,#12840);
#10294=LINE('',#58965,#12841);
#10295=LINE('',#58971,#12842);
#10296=LINE('',#58973,#12843);
#10297=LINE('',#58975,#12844);
#10298=LINE('',#58976,#12845);
#10299=LINE('',#58981,#12846);
#10300=LINE('',#58985,#12847);
#10301=LINE('',#58987,#12848);
#10302=LINE('',#58992,#12849);
#10303=LINE('',#58994,#12850);
#10304=LINE('',#58996,#12851);
#10305=LINE('',#58998,#12852);
#10306=LINE('',#59000,#12853);
#10307=LINE('',#59002,#12854);
#10308=LINE('',#59003,#12855);
#10309=LINE('',#59012,#12856);
#10310=LINE('',#59019,#12857);
#10311=LINE('',#59024,#12858);
#10312=LINE('',#59030,#12859);
#10313=LINE('',#59035,#12860);
#10314=LINE('',#59040,#12861);
#10315=LINE('',#59043,#12862);
#10316=LINE('',#59044,#12863);
#10317=LINE('',#59046,#12864);
#10318=LINE('',#59050,#12865);
#10319=LINE('',#59052,#12866);
#10320=LINE('',#59054,#12867);
#10321=LINE('',#59055,#12868);
#10322=LINE('',#59058,#12869);
#10323=LINE('',#59060,#12870);
#10324=LINE('',#59061,#12871);
#10325=LINE('',#59064,#12872);
#10326=LINE('',#59066,#12873);
#10327=LINE('',#59067,#12874);
#10328=LINE('',#59069,#12875);
#10329=LINE('',#59081,#12876);
#10330=LINE('',#59090,#12877);
#10331=LINE('',#59098,#12878);
#10332=LINE('',#59106,#12879);
#10333=LINE('',#59114,#12880);
#10334=LINE('',#59119,#12881);
#10335=LINE('',#59121,#12882);
#10336=LINE('',#59123,#12883);
#10337=LINE('',#59124,#12884);
#10338=LINE('',#59125,#12885);
#10339=LINE('',#59127,#12886);
#10340=LINE('',#59129,#12887);
#10341=LINE('',#59131,#12888);
#10342=LINE('',#59132,#12889);
#10343=LINE('',#59134,#12890);
#10344=LINE('',#59139,#12891);
#10345=LINE('',#59141,#12892);
#10346=LINE('',#59142,#12893);
#10347=LINE('',#59146,#12894);
#10348=LINE('',#59148,#12895);
#10349=LINE('',#59151,#12896);
#10350=LINE('',#59156,#12897);
#10351=LINE('',#59166,#12898);
#10352=LINE('',#59172,#12899);
#10353=LINE('',#59174,#12900);
#10354=LINE('',#59175,#12901);
#10355=LINE('',#59183,#12902);
#10356=LINE('',#59188,#12903);
#10357=LINE('',#59189,#12904);
#10358=LINE('',#59197,#12905);
#10359=LINE('',#59202,#12906);
#10360=LINE('',#59203,#12907);
#10361=LINE('',#59211,#12908);
#10362=LINE('',#59216,#12909);
#10363=LINE('',#59217,#12910);
#10364=LINE('',#59246,#12911);
#10365=LINE('',#59248,#12912);
#10366=LINE('',#59249,#12913);
#10367=LINE('',#59251,#12914);
#10368=LINE('',#59252,#12915);
#10369=LINE('',#59263,#12916);
#10370=LINE('',#59269,#12917);
#10371=LINE('',#59271,#12918);
#10372=LINE('',#59272,#12919);
#10373=LINE('',#59280,#12920);
#10374=LINE('',#59285,#12921);
#10375=LINE('',#59286,#12922);
#10376=LINE('',#59294,#12923);
#10377=LINE('',#59299,#12924);
#10378=LINE('',#59300,#12925);
#10379=LINE('',#59308,#12926);
#10380=LINE('',#59313,#12927);
#10381=LINE('',#59314,#12928);
#10382=LINE('',#59343,#12929);
#10383=LINE('',#59345,#12930);
#10384=LINE('',#59346,#12931);
#10385=LINE('',#59348,#12932);
#10386=LINE('',#59349,#12933);
#10387=LINE('',#59355,#12934);
#10388=LINE('',#59356,#12935);
#10389=LINE('',#59359,#12936);
#10390=LINE('',#59361,#12937);
#10391=LINE('',#59362,#12938);
#10392=LINE('',#59365,#12939);
#10393=LINE('',#59366,#12940);
#10394=LINE('',#59369,#12941);
#10395=LINE('',#59370,#12942);
#10396=LINE('',#59373,#12943);
#10397=LINE('',#59374,#12944);
#10398=LINE('',#59377,#12945);
#10399=LINE('',#59378,#12946);
#10400=LINE('',#59380,#12947);
#10401=LINE('',#59383,#12948);
#10402=LINE('',#59385,#12949);
#10403=LINE('',#59395,#12950);
#10404=LINE('',#59397,#12951);
#10405=LINE('',#59399,#12952);
#10406=LINE('',#59401,#12953);
#10407=LINE('',#59403,#12954);
#10408=LINE('',#59404,#12955);
#10409=LINE('',#59408,#12956);
#10410=LINE('',#59409,#12957);
#10411=LINE('',#59410,#12958);
#10412=LINE('',#59413,#12959);
#10413=LINE('',#59414,#12960);
#10414=LINE('',#59417,#12961);
#10415=LINE('',#59418,#12962);
#10416=LINE('',#59421,#12963);
#10417=LINE('',#59422,#12964);
#10418=LINE('',#59425,#12965);
#10419=LINE('',#59426,#12966);
#10420=LINE('',#59428,#12967);
#10421=LINE('',#59435,#12968);
#10422=LINE('',#59437,#12969);
#10423=LINE('',#59439,#12970);
#10424=LINE('',#59441,#12971);
#10425=LINE('',#59443,#12972);
#10426=LINE('',#59444,#12973);
#10427=LINE('',#59448,#12974);
#10428=LINE('',#59449,#12975);
#10429=LINE('',#59450,#12976);
#10430=LINE('',#59453,#12977);
#10431=LINE('',#59454,#12978);
#10432=LINE('',#59457,#12979);
#10433=LINE('',#59458,#12980);
#10434=LINE('',#59461,#12981);
#10435=LINE('',#59462,#12982);
#10436=LINE('',#59465,#12983);
#10437=LINE('',#59466,#12984);
#10438=LINE('',#59468,#12985);
#10439=LINE('',#59474,#12986);
#10440=LINE('',#59475,#12987);
#10441=LINE('',#59478,#12988);
#10442=LINE('',#59479,#12989);
#10443=LINE('',#59481,#12990);
#10444=LINE('',#59486,#12991);
#10445=LINE('',#59490,#12992);
#10446=LINE('',#59496,#12993);
#10447=LINE('',#59502,#12994);
#10448=LINE('',#59507,#12995);
#10449=LINE('',#59513,#12996);
#10450=LINE('',#59519,#12997);
#10451=LINE('',#59524,#12998);
#10452=LINE('',#59530,#12999);
#10453=LINE('',#59536,#13000);
#10454=LINE('',#59544,#13001);
#10455=LINE('',#59548,#13002);
#10456=LINE('',#59554,#13003);
#10457=LINE('',#59561,#13004);
#10458=LINE('',#59565,#13005);
#10459=LINE('',#59571,#13006);
#10460=LINE('',#59578,#13007);
#10461=LINE('',#59582,#13008);
#10462=LINE('',#59588,#13009);
#10463=LINE('',#59595,#13010);
#10464=LINE('',#59599,#13011);
#10465=LINE('',#59605,#13012);
#10466=LINE('',#59608,#13013);
#10467=LINE('',#59611,#13014);
#10468=LINE('',#59614,#13015);
#10469=LINE('',#59617,#13016);
#10470=LINE('',#59620,#13017);
#10471=LINE('',#59623,#13018);
#10472=LINE('',#59626,#13019);
#10473=LINE('',#59629,#13020);
#10474=LINE('',#59632,#13021);
#10475=LINE('',#59634,#13022);
#10476=LINE('',#59635,#13023);
#10477=LINE('',#59638,#13024);
#10478=LINE('',#59639,#13025);
#10479=LINE('',#59642,#13026);
#10480=LINE('',#59644,#13027);
#10481=LINE('',#59645,#13028);
#10482=LINE('',#59648,#13029);
#10483=LINE('',#59649,#13030);
#10484=LINE('',#59652,#13031);
#10485=LINE('',#59653,#13032);
#10486=LINE('',#59656,#13033);
#10487=LINE('',#59657,#13034);
#10488=LINE('',#59660,#13035);
#10489=LINE('',#59661,#13036);
#10490=LINE('',#59663,#13037);
#10491=LINE('',#59666,#13038);
#10492=LINE('',#59667,#13039);
#10493=LINE('',#59670,#13040);
#10494=LINE('',#59672,#13041);
#10495=LINE('',#59674,#13042);
#10496=LINE('',#59676,#13043);
#10497=LINE('',#59678,#13044);
#10498=LINE('',#59680,#13045);
#10499=LINE('',#59682,#13046);
#10500=LINE('',#59683,#13047);
#10501=LINE('',#59691,#13048);
#10502=LINE('',#59698,#13049);
#10503=LINE('',#59703,#13050);
#10504=LINE('',#59706,#13051);
#10505=LINE('',#59707,#13052);
#10506=LINE('',#59710,#13053);
#10507=LINE('',#59711,#13054);
#10508=LINE('',#59714,#13055);
#10509=LINE('',#59715,#13056);
#10510=LINE('',#59718,#13057);
#10511=LINE('',#59719,#13058);
#10512=LINE('',#59722,#13059);
#10513=LINE('',#59723,#13060);
#10514=LINE('',#59725,#13061);
#10515=LINE('',#59728,#13062);
#10516=LINE('',#59737,#13063);
#10517=LINE('',#59741,#13064);
#10518=LINE('',#59821,#13065);
#10519=LINE('',#59824,#13066);
#10520=LINE('',#59825,#13067);
#10521=LINE('',#59832,#13068);
#10522=LINE('',#59840,#13069);
#10523=LINE('',#59845,#13070);
#10524=LINE('',#59847,#13071);
#10525=LINE('',#59849,#13072);
#10526=LINE('',#59851,#13073);
#10527=LINE('',#59853,#13074);
#10528=LINE('',#59854,#13075);
#10529=LINE('',#59857,#13076);
#10530=LINE('',#59859,#13077);
#10531=LINE('',#59861,#13078);
#10532=LINE('',#59863,#13079);
#10533=LINE('',#59865,#13080);
#10534=LINE('',#59866,#13081);
#10535=LINE('',#59873,#13082);
#10536=LINE('',#59881,#13083);
#10537=LINE('',#59889,#13084);
#10538=LINE('',#59894,#13085);
#10539=LINE('',#59896,#13086);
#10540=LINE('',#59899,#13087);
#10541=LINE('',#59917,#13088);
#10542=LINE('',#59920,#13089);
#10543=LINE('',#59997,#13090);
#10544=LINE('',#60000,#13091);
#10545=LINE('',#60001,#13092);
#10546=LINE('',#60005,#13093);
#10547=LINE('',#60007,#13094);
#10548=LINE('',#60009,#13095);
#10549=LINE('',#60011,#13096);
#10550=LINE('',#60013,#13097);
#10551=LINE('',#60014,#13098);
#10552=LINE('',#60018,#13099);
#10553=LINE('',#60019,#13100);
#10554=LINE('',#60020,#13101);
#10555=LINE('',#60023,#13102);
#10556=LINE('',#60024,#13103);
#10557=LINE('',#60027,#13104);
#10558=LINE('',#60028,#13105);
#10559=LINE('',#60031,#13106);
#10560=LINE('',#60032,#13107);
#10561=LINE('',#60035,#13108);
#10562=LINE('',#60036,#13109);
#10563=LINE('',#60038,#13110);
#10564=LINE('',#60042,#13111);
#10565=LINE('',#60044,#13112);
#10566=LINE('',#60046,#13113);
#10567=LINE('',#60048,#13114);
#10568=LINE('',#60050,#13115);
#10569=LINE('',#60051,#13116);
#10570=LINE('',#60055,#13117);
#10571=LINE('',#60056,#13118);
#10572=LINE('',#60057,#13119);
#10573=LINE('',#60060,#13120);
#10574=LINE('',#60061,#13121);
#10575=LINE('',#60064,#13122);
#10576=LINE('',#60065,#13123);
#10577=LINE('',#60068,#13124);
#10578=LINE('',#60069,#13125);
#10579=LINE('',#60072,#13126);
#10580=LINE('',#60073,#13127);
#10581=LINE('',#60075,#13128);
#10582=LINE('',#60084,#13129);
#10583=LINE('',#60121,#13130);
#10584=LINE('',#60128,#13131);
#10585=LINE('',#60139,#13132);
#10586=LINE('',#60143,#13133);
#10587=LINE('',#60145,#13134);
#10588=LINE('',#60147,#13135);
#10589=LINE('',#60149,#13136);
#10590=LINE('',#60151,#13137);
#10591=LINE('',#60152,#13138);
#10592=LINE('',#60156,#13139);
#10593=LINE('',#60157,#13140);
#10594=LINE('',#60158,#13141);
#10595=LINE('',#60161,#13142);
#10596=LINE('',#60162,#13143);
#10597=LINE('',#60165,#13144);
#10598=LINE('',#60166,#13145);
#10599=LINE('',#60169,#13146);
#10600=LINE('',#60170,#13147);
#10601=LINE('',#60173,#13148);
#10602=LINE('',#60174,#13149);
#10603=LINE('',#60176,#13150);
#10604=LINE('',#60180,#13151);
#10605=LINE('',#60182,#13152);
#10606=LINE('',#60184,#13153);
#10607=LINE('',#60186,#13154);
#10608=LINE('',#60188,#13155);
#10609=LINE('',#60189,#13156);
#10610=LINE('',#60193,#13157);
#10611=LINE('',#60194,#13158);
#10612=LINE('',#60195,#13159);
#10613=LINE('',#60198,#13160);
#10614=LINE('',#60199,#13161);
#10615=LINE('',#60202,#13162);
#10616=LINE('',#60203,#13163);
#10617=LINE('',#60206,#13164);
#10618=LINE('',#60207,#13165);
#10619=LINE('',#60210,#13166);
#10620=LINE('',#60211,#13167);
#10621=LINE('',#60213,#13168);
#10622=LINE('',#60222,#13169);
#10623=LINE('',#60259,#13170);
#10624=LINE('',#60266,#13171);
#10625=LINE('',#60277,#13172);
#10626=LINE('',#60314,#13173);
#10627=LINE('',#60317,#13174);
#10628=LINE('',#60321,#13175);
#10629=LINE('',#60323,#13176);
#10630=LINE('',#60328,#13177);
#10631=LINE('',#60365,#13178);
#10632=LINE('',#60372,#13179);
#10633=LINE('',#60375,#13180);
#10634=LINE('',#60390,#13181);
#10635=LINE('',#60398,#13182);
#10636=LINE('',#60401,#13183);
#10637=LINE('',#60408,#13184);
#10638=LINE('',#60414,#13185);
#10639=LINE('',#60418,#13186);
#10640=LINE('',#60422,#13187);
#10641=LINE('',#60426,#13188);
#10642=LINE('',#60430,#13189);
#10643=LINE('',#60433,#13190);
#10644=LINE('',#60451,#13191);
#10645=LINE('',#60452,#13192);
#10646=LINE('',#60461,#13193);
#10647=LINE('',#60488,#13194);
#10648=LINE('',#60490,#13195);
#10649=LINE('',#60492,#13196);
#10650=LINE('',#60499,#13197);
#10651=LINE('',#60503,#13198);
#10652=LINE('',#60507,#13199);
#10653=LINE('',#60511,#13200);
#10654=LINE('',#60515,#13201);
#10655=LINE('',#60518,#13202);
#10656=LINE('',#60536,#13203);
#10657=LINE('',#60537,#13204);
#10658=LINE('',#60546,#13205);
#10659=LINE('',#60573,#13206);
#10660=LINE('',#60575,#13207);
#10661=LINE('',#60577,#13208);
#10662=LINE('',#60592,#13209);
#10663=LINE('',#60598,#13210);
#10664=LINE('',#60603,#13211);
#10665=LINE('',#60608,#13212);
#10666=LINE('',#60614,#13213);
#10667=LINE('',#60620,#13214);
#10668=LINE('',#60626,#13215);
#10669=LINE('',#60635,#13216);
#10670=LINE('',#60643,#13217);
#10671=LINE('',#60648,#13218);
#10672=LINE('',#60650,#13219);
#10673=LINE('',#60652,#13220);
#10674=LINE('',#60653,#13221);
#10675=LINE('',#60658,#13222);
#10676=LINE('',#60664,#13223);
#10677=LINE('',#60670,#13224);
#10678=LINE('',#60674,#13225);
#10679=LINE('',#60676,#13226);
#10680=LINE('',#60677,#13227);
#10681=LINE('',#60682,#13228);
#10682=LINE('',#60688,#13229);
#10683=LINE('',#60697,#13230);
#10684=LINE('',#60699,#13231);
#10685=LINE('',#60701,#13232);
#10686=LINE('',#60702,#13233);
#10687=LINE('',#60707,#13234);
#10688=LINE('',#60713,#13235);
#10689=LINE('',#60719,#13236);
#10690=LINE('',#60723,#13237);
#10691=LINE('',#60725,#13238);
#10692=LINE('',#60726,#13239);
#10693=LINE('',#60731,#13240);
#10694=LINE('',#60737,#13241);
#10695=LINE('',#60746,#13242);
#10696=LINE('',#60748,#13243);
#10697=LINE('',#60750,#13244);
#10698=LINE('',#60751,#13245);
#10699=LINE('',#60756,#13246);
#10700=LINE('',#60762,#13247);
#10701=LINE('',#60768,#13248);
#10702=LINE('',#60772,#13249);
#10703=LINE('',#60774,#13250);
#10704=LINE('',#60775,#13251);
#10705=LINE('',#60780,#13252);
#10706=LINE('',#60786,#13253);
#10707=LINE('',#60794,#13254);
#10708=LINE('',#60798,#13255);
#10709=LINE('',#60802,#13256);
#10710=LINE('',#60814,#13257);
#10711=LINE('',#60825,#13258);
#10712=LINE('',#60836,#13259);
#10713=LINE('',#60840,#13260);
#10714=LINE('',#60842,#13261);
#10715=LINE('',#60846,#13262);
#10716=LINE('',#60848,#13263);
#10717=LINE('',#60853,#13264);
#10718=LINE('',#60857,#13265);
#10719=LINE('',#60859,#13266);
#10720=LINE('',#60862,#13267);
#10721=LINE('',#60866,#13268);
#10722=LINE('',#60870,#13269);
#10723=LINE('',#60872,#13270);
#10724=LINE('',#60875,#13271);
#10725=LINE('',#60882,#13272);
#10726=LINE('',#60888,#13273);
#10727=LINE('',#60890,#13274);
#10728=LINE('',#60891,#13275);
#10729=LINE('',#60894,#13276);
#10730=LINE('',#60896,#13277);
#10731=LINE('',#60897,#13278);
#10732=LINE('',#60900,#13279);
#10733=LINE('',#60902,#13280);
#10734=LINE('',#60903,#13281);
#10735=LINE('',#60906,#13282);
#10736=LINE('',#60908,#13283);
#10737=LINE('',#60909,#13284);
#10738=LINE('',#60912,#13285);
#10739=LINE('',#60914,#13286);
#10740=LINE('',#60915,#13287);
#10741=LINE('',#60917,#13288);
#10742=LINE('',#60919,#13289);
#10743=LINE('',#60920,#13290);
#10744=LINE('',#60921,#13291);
#10745=LINE('',#60924,#13292);
#10746=LINE('',#60928,#13293);
#10747=LINE('',#60929,#13294);
#10748=LINE('',#60931,#13295);
#10749=LINE('',#60933,#13296);
#10750=LINE('',#60934,#13297);
#10751=LINE('',#60935,#13298);
#10752=LINE('',#60938,#13299);
#10753=LINE('',#60942,#13300);
#10754=LINE('',#60943,#13301);
#10755=LINE('',#60945,#13302);
#10756=LINE('',#60947,#13303);
#10757=LINE('',#60949,#13304);
#10758=LINE('',#60951,#13305);
#10759=LINE('',#60952,#13306);
#10760=LINE('',#60957,#13307);
#10761=LINE('',#60962,#13308);
#10762=LINE('',#60966,#13309);
#10763=LINE('',#60969,#13310);
#10764=LINE('',#60971,#13311);
#10765=LINE('',#60973,#13312);
#10766=LINE('',#60975,#13313);
#10767=LINE('',#60976,#13314);
#10768=LINE('',#60977,#13315);
#10769=LINE('',#60982,#13316);
#10770=LINE('',#60984,#13317);
#10771=LINE('',#60987,#13318);
#10772=LINE('',#60989,#13319);
#10773=LINE('',#60992,#13320);
#10774=LINE('',#60994,#13321);
#10775=LINE('',#60997,#13322);
#10776=LINE('',#60999,#13323);
#10777=LINE('',#61003,#13324);
#10778=LINE('',#61004,#13325);
#10779=LINE('',#61008,#13326);
#10780=LINE('',#61010,#13327);
#10781=LINE('',#61012,#13328);
#10782=LINE('',#61014,#13329);
#10783=LINE('',#61017,#13330);
#10784=LINE('',#61019,#13331);
#10785=LINE('',#61022,#13332);
#10786=LINE('',#61024,#13333);
#10787=LINE('',#61036,#13334);
#10788=LINE('',#61039,#13335);
#10789=LINE('',#61042,#13336);
#10790=LINE('',#61044,#13337);
#10791=LINE('',#61045,#13338);
#10792=LINE('',#61050,#13339);
#10793=LINE('',#61056,#13340);
#10794=LINE('',#61062,#13341);
#10795=LINE('',#61066,#13342);
#10796=LINE('',#61068,#13343);
#10797=LINE('',#61069,#13344);
#10798=LINE('',#61074,#13345);
#10799=LINE('',#61083,#13346);
#10800=LINE('',#61085,#13347);
#10801=LINE('',#61087,#13348);
#10802=LINE('',#61088,#13349);
#10803=LINE('',#61093,#13350);
#10804=LINE('',#61099,#13351);
#10805=LINE('',#61105,#13352);
#10806=LINE('',#61109,#13353);
#10807=LINE('',#61111,#13354);
#10808=LINE('',#61112,#13355);
#10809=LINE('',#61117,#13356);
#10810=LINE('',#61123,#13357);
#10811=LINE('',#61134,#13358);
#10812=LINE('',#61137,#13359);
#10813=LINE('',#61142,#13360);
#10814=LINE('',#61146,#13361);
#10815=LINE('',#61148,#13362);
#10816=LINE('',#61149,#13363);
#10817=LINE('',#61154,#13364);
#10818=LINE('',#61160,#13365);
#10819=LINE('',#61166,#13366);
#10820=LINE('',#61170,#13367);
#10821=LINE('',#61172,#13368);
#10822=LINE('',#61173,#13369);
#10823=LINE('',#61183,#13370);
#10824=LINE('',#61186,#13371);
#10825=LINE('',#61191,#13372);
#10826=LINE('',#61195,#13373);
#10827=LINE('',#61197,#13374);
#10828=LINE('',#61198,#13375);
#10829=LINE('',#61203,#13376);
#10830=LINE('',#61209,#13377);
#10831=LINE('',#61215,#13378);
#10832=LINE('',#61219,#13379);
#10833=LINE('',#61221,#13380);
#10834=LINE('',#61222,#13381);
#10835=LINE('',#61231,#13382);
#10836=LINE('',#61232,#13383);
#10837=LINE('',#61236,#13384);
#10838=LINE('',#61239,#13385);
#10839=LINE('',#61240,#13386);
#10840=LINE('',#61244,#13387);
#10841=LINE('',#61248,#13388);
#10842=LINE('',#61252,#13389);
#10843=LINE('',#61256,#13390);
#10844=LINE('',#61258,#13391);
#10845=LINE('',#61266,#13392);
#10846=LINE('',#61268,#13393);
#10847=LINE('',#61270,#13394);
#10848=LINE('',#61272,#13395);
#10849=LINE('',#61274,#13396);
#10850=LINE('',#61276,#13397);
#10851=LINE('',#61278,#13398);
#10852=LINE('',#61279,#13399);
#10853=LINE('',#61281,#13400);
#10854=LINE('',#61282,#13401);
#10855=LINE('',#61284,#13402);
#10856=LINE('',#61285,#13403);
#10857=LINE('',#61288,#13404);
#10858=LINE('',#61289,#13405);
#10859=LINE('',#61291,#13406);
#10860=LINE('',#61294,#13407);
#10861=LINE('',#61304,#13408);
#10862=LINE('',#61308,#13409);
#10863=LINE('',#61313,#13410);
#10864=LINE('',#61317,#13411);
#10865=LINE('',#61319,#13412);
#10866=LINE('',#61321,#13413);
#10867=LINE('',#61322,#13414);
#10868=LINE('',#61325,#13415);
#10869=LINE('',#61327,#13416);
#10870=LINE('',#61328,#13417);
#10871=LINE('',#61331,#13418);
#10872=LINE('',#61333,#13419);
#10873=LINE('',#61334,#13420);
#10874=LINE('',#61337,#13421);
#10875=LINE('',#61339,#13422);
#10876=LINE('',#61340,#13423);
#10877=LINE('',#61343,#13424);
#10878=LINE('',#61345,#13425);
#10879=LINE('',#61346,#13426);
#10880=LINE('',#61348,#13427);
#10881=LINE('',#61350,#13428);
#12747=VECTOR('',#46298,3.21359174399996);
#12748=VECTOR('',#46305,0.322047616000012);
#12749=VECTOR('',#46312,3.22047616000001);
#12750=VECTOR('',#46317,3.9116);
#12751=VECTOR('',#46330,4.19099999999999);
#12752=VECTOR('',#46337,3.21359174400012);
#12753=VECTOR('',#46344,0.322047616);
#12754=VECTOR('',#46351,3.22047616000001);
#12755=VECTOR('',#46356,3.91160000000001);
#12756=VECTOR('',#46369,4.19099999999999);
#12757=VECTOR('',#46374,2.74142809600001);
#12758=VECTOR('',#46387,2.74750784000002);
#12759=VECTOR('',#46390,0.274750783999988);
#12760=VECTOR('',#46395,3.3527999999999);
#12761=VECTOR('',#46406,3.6322);
#12762=VECTOR('',#46413,3.9116);
#12763=VECTOR('',#46422,4.191);
#12764=VECTOR('',#46433,3.21359174400008);
#12765=VECTOR('',#46444,3.22047616000001);
#12766=VECTOR('',#46447,0.322047616);
#12767=VECTOR('',#46452,3.91160000000001);
#12768=VECTOR('',#46461,4.19099999999999);
#12769=VECTOR('',#46472,3.21359174399998);
#12770=VECTOR('',#46483,3.22047616000001);
#12771=VECTOR('',#46486,0.322047616000012);
#12772=VECTOR('',#46489,10.);
#12773=VECTOR('',#46490,10.);
#12774=VECTOR('',#46491,10.);
#12775=VECTOR('',#46492,10.);
#12776=VECTOR('',#46493,10.);
#12777=VECTOR('',#46494,10.);
#12778=VECTOR('',#46495,10.);
#12779=VECTOR('',#46496,10.);
#12780=VECTOR('',#46497,10.);
#12781=VECTOR('',#46498,10.);
#12782=VECTOR('',#46499,10.);
#12783=VECTOR('',#46500,10.);
#12784=VECTOR('',#46501,10.);
#12785=VECTOR('',#46502,10.);
#12786=VECTOR('',#46507,10.);
#12787=VECTOR('',#46510,10.);
#12788=VECTOR('',#46513,10.);
#12789=VECTOR('',#46514,10.);
#12790=VECTOR('',#46515,10.);
#12791=VECTOR('',#46520,10.);
#12792=VECTOR('',#46523,10.);
#12793=VECTOR('',#46526,10.);
#12794=VECTOR('',#46527,10.);
#12795=VECTOR('',#46528,10.);
#12796=VECTOR('',#46529,10.);
#12797=VECTOR('',#46530,10.);
#12798=VECTOR('',#46533,9.99999999999999);
#12799=VECTOR('',#46534,10.);
#12800=VECTOR('',#46535,10.);
#12801=VECTOR('',#46536,10.);
#12802=VECTOR('',#46539,10.);
#12803=VECTOR('',#46540,10.);
#12804=VECTOR('',#46541,10.);
#12805=VECTOR('',#46546,10.);
#12806=VECTOR('',#46549,10.);
#12807=VECTOR('',#46550,10.);
#12808=VECTOR('',#46551,10.);
#12809=VECTOR('',#46552,10.);
#12810=VECTOR('',#46555,10.);
#12811=VECTOR('',#46556,10.);
#12812=VECTOR('',#46561,10.);
#12813=VECTOR('',#46562,10.);
#12814=VECTOR('',#46563,10.);
#12815=VECTOR('',#46568,10.);
#12816=VECTOR('',#46569,10.);
#12817=VECTOR('',#46570,10.);
#12818=VECTOR('',#46579,4.70822528);
#12819=VECTOR('',#46588,10.);
#12820=VECTOR('',#46591,10.);
#12821=VECTOR('',#46592,10.);
#12822=VECTOR('',#46593,10.);
#12823=VECTOR('',#46594,10.);
#12824=VECTOR('',#46595,10.);
#12825=VECTOR('',#46596,10.);
#12826=VECTOR('',#46605,4.70822528000001);
#12827=VECTOR('',#46612,10.);
#12828=VECTOR('',#46617,10.);
#12829=VECTOR('',#46618,10.);
#12830=VECTOR('',#46621,10.);
#12831=VECTOR('',#46624,10.);
#12832=VECTOR('',#46625,10.);
#12833=VECTOR('',#46626,10.);
#12834=VECTOR('',#46627,10.);
#12835=VECTOR('',#46628,10.);
#12836=VECTOR('',#46631,4.70822528000003);
#12837=VECTOR('',#46638,10.);
#12838=VECTOR('',#46639,10.);
#12839=VECTOR('',#46642,10.);
#12840=VECTOR('',#46643,10.);
#12841=VECTOR('',#46646,4.70822527999992);
#12842=VECTOR('',#46653,10.);
#12843=VECTOR('',#46654,10.);
#12844=VECTOR('',#46655,10.);
#12845=VECTOR('',#46656,10.);
#12846=VECTOR('',#46663,10.);
#12847=VECTOR('',#46666,10.);
#12848=VECTOR('',#46667,10.);
#12849=VECTOR('',#46668,10.);
#12850=VECTOR('',#46669,10.);
#12851=VECTOR('',#46670,10.);
#12852=VECTOR('',#46671,10.);
#12853=VECTOR('',#46672,10.);
#12854=VECTOR('',#46673,10.);
#12855=VECTOR('',#46674,10.);
#12856=VECTOR('',#46679,28.8698432);
#12857=VECTOR('',#46686,10.);
#12858=VECTOR('',#46691,10.);
#12859=VECTOR('',#46696,28.8519616);
#12860=VECTOR('',#46701,10.);
#12861=VECTOR('',#46706,10.);
#12862=VECTOR('',#46709,10.);
#12863=VECTOR('',#46710,10.);
#12864=VECTOR('',#46713,10.);
#12865=VECTOR('',#46716,10.);
#12866=VECTOR('',#46717,10.);
#12867=VECTOR('',#46718,10.);
#12868=VECTOR('',#46719,10.);
#12869=VECTOR('',#46722,10.);
#12870=VECTOR('',#46723,10.);
#12871=VECTOR('',#46724,10.);
#12872=VECTOR('',#46727,10.);
#12873=VECTOR('',#46728,10.);
#12874=VECTOR('',#46729,10.);
#12875=VECTOR('',#46732,10.);
#12876=VECTOR('',#46739,10.);
#12877=VECTOR('',#46748,4.70822528000001);
#12878=VECTOR('',#46757,4.70822528);
#12879=VECTOR('',#46766,4.70822528000001);
#12880=VECTOR('',#46775,4.70822528000002);
#12881=VECTOR('',#46782,10.);
#12882=VECTOR('',#46783,10.);
#12883=VECTOR('',#46784,10.);
#12884=VECTOR('',#46785,10.);
#12885=VECTOR('',#46786,10.);
#12886=VECTOR('',#46789,10.);
#12887=VECTOR('',#46790,10.);
#12888=VECTOR('',#46791,10.);
#12889=VECTOR('',#46792,10.);
#12890=VECTOR('',#46795,10.);
#12891=VECTOR('',#46800,10.);
#12892=VECTOR('',#46801,10.);
#12893=VECTOR('',#46802,10.);
#12894=VECTOR('',#46805,10.);
#12895=VECTOR('',#46806,10.);
#12896=VECTOR('',#46809,10.);
#12897=VECTOR('',#46814,22.5);
#12898=VECTOR('',#46821,10.);
#12899=VECTOR('',#46822,10.);
#12900=VECTOR('',#46823,10.);
#12901=VECTOR('',#46824,10.);
#12902=VECTOR('',#46827,10.);
#12903=VECTOR('',#46828,10.);
#12904=VECTOR('',#46829,10.);
#12905=VECTOR('',#46832,10.);
#12906=VECTOR('',#46833,10.);
#12907=VECTOR('',#46834,10.);
#12908=VECTOR('',#46837,10.);
#12909=VECTOR('',#46838,10.);
#12910=VECTOR('',#46839,10.);
#12911=VECTOR('',#46862,10.);
#12912=VECTOR('',#46863,10.);
#12913=VECTOR('',#46864,10.);
#12914=VECTOR('',#46867,10.);
#12915=VECTOR('',#46868,10.);
#12916=VECTOR('',#46877,10.);
#12917=VECTOR('',#46878,10.);
#12918=VECTOR('',#46879,10.);
#12919=VECTOR('',#46880,10.);
#12920=VECTOR('',#46883,10.);
#12921=VECTOR('',#46884,10.);
#12922=VECTOR('',#46885,10.);
#12923=VECTOR('',#46888,10.);
#12924=VECTOR('',#46889,10.);
#12925=VECTOR('',#46890,10.);
#12926=VECTOR('',#46893,10.);
#12927=VECTOR('',#46894,10.);
#12928=VECTOR('',#46895,10.);
#12929=VECTOR('',#46918,10.);
#12930=VECTOR('',#46919,10.);
#12931=VECTOR('',#46920,10.);
#12932=VECTOR('',#46923,10.);
#12933=VECTOR('',#46924,10.);
#12934=VECTOR('',#46933,10.);
#12935=VECTOR('',#46934,10.);
#12936=VECTOR('',#46937,10.);
#12937=VECTOR('',#46938,10.);
#12938=VECTOR('',#46939,10.);
#12939=VECTOR('',#46942,10.);
#12940=VECTOR('',#46943,10.);
#12941=VECTOR('',#46946,10.);
#12942=VECTOR('',#46947,10.);
#12943=VECTOR('',#46950,10.);
#12944=VECTOR('',#46951,10.);
#12945=VECTOR('',#46954,10.);
#12946=VECTOR('',#46955,10.);
#12947=VECTOR('',#46958,10.);
#12948=VECTOR('',#46963,10.);
#12949=VECTOR('',#46966,10.);
#12950=VECTOR('',#46981,10.);
#12951=VECTOR('',#46982,10.);
#12952=VECTOR('',#46983,10.);
#12953=VECTOR('',#46984,10.);
#12954=VECTOR('',#46985,10.);
#12955=VECTOR('',#46986,10.);
#12956=VECTOR('',#46989,10.);
#12957=VECTOR('',#46990,10.);
#12958=VECTOR('',#46991,10.);
#12959=VECTOR('',#46994,10.);
#12960=VECTOR('',#46995,10.);
#12961=VECTOR('',#46998,10.);
#12962=VECTOR('',#46999,10.);
#12963=VECTOR('',#47002,10.);
#12964=VECTOR('',#47003,10.);
#12965=VECTOR('',#47006,10.);
#12966=VECTOR('',#47007,10.);
#12967=VECTOR('',#47010,10.);
#12968=VECTOR('',#47019,10.);
#12969=VECTOR('',#47020,10.);
#12970=VECTOR('',#47021,10.);
#12971=VECTOR('',#47022,10.);
#12972=VECTOR('',#47023,10.);
#12973=VECTOR('',#47024,9.99999999999999);
#12974=VECTOR('',#47027,9.99999999999999);
#12975=VECTOR('',#47028,10.);
#12976=VECTOR('',#47029,10.);
#12977=VECTOR('',#47032,10.);
#12978=VECTOR('',#47033,10.);
#12979=VECTOR('',#47036,10.);
#12980=VECTOR('',#47037,10.);
#12981=VECTOR('',#47040,10.);
#12982=VECTOR('',#47041,10.);
#12983=VECTOR('',#47044,10.);
#12984=VECTOR('',#47045,10.);
#12985=VECTOR('',#47048,10.);
#12986=VECTOR('',#47057,10.);
#12987=VECTOR('',#47058,10.);
#12988=VECTOR('',#47061,10.);
#12989=VECTOR('',#47062,10.);
#12990=VECTOR('',#47065,10.);
#12991=VECTOR('',#47072,5.83240278777977);
#12992=VECTOR('',#47075,0.274750783999998);
#12993=VECTOR('',#47082,2.74750784);
#12994=VECTOR('',#47089,2.80803705600002);
#12995=VECTOR('',#47094,0.274750783999993);
#12996=VECTOR('',#47101,2.74750784000001);
#12997=VECTOR('',#47108,2.808037056);
#12998=VECTOR('',#47113,0.274750783999995);
#12999=VECTOR('',#47120,2.74750784);
#13000=VECTOR('',#47127,2.80803705600003);
#13001=VECTOR('',#47136,3.28958854399998);
#13002=VECTOR('',#47141,3.2204761600001);
#13003=VECTOR('',#47148,0.322047616000123);
#13004=VECTOR('',#47155,3.2895885439999);
#13005=VECTOR('',#47160,3.22047616000001);
#13006=VECTOR('',#47167,0.322047615999997);
#13007=VECTOR('',#47174,3.289588544);
#13008=VECTOR('',#47179,3.22047616000007);
#13009=VECTOR('',#47186,0.322047616000094);
#13010=VECTOR('',#47193,3.2895885439999);
#13011=VECTOR('',#47198,3.22047616000001);
#13012=VECTOR('',#47205,0.32204761600005);
#13013=VECTOR('',#47208,0.470822528000023);
#13014=VECTOR('',#47211,0.470822528000024);
#13015=VECTOR('',#47214,0.470822528000001);
#13016=VECTOR('',#47217,0.470822528000002);
#13017=VECTOR('',#47220,0.47082252800002);
#13018=VECTOR('',#47223,0.470822528000018);
#13019=VECTOR('',#47226,0.470822528000013);
#13020=VECTOR('',#47229,0.470822528000016);
#13021=VECTOR('',#47232,10.);
#13022=VECTOR('',#47233,10.);
#13023=VECTOR('',#47234,10.);
#13024=VECTOR('',#47237,10.);
#13025=VECTOR('',#47238,10.);
#13026=VECTOR('',#47241,10.);
#13027=VECTOR('',#47242,10.);
#13028=VECTOR('',#47243,10.);
#13029=VECTOR('',#47246,10.);
#13030=VECTOR('',#47247,10.);
#13031=VECTOR('',#47250,10.);
#13032=VECTOR('',#47251,10.);
#13033=VECTOR('',#47254,10.);
#13034=VECTOR('',#47255,10.);
#13035=VECTOR('',#47258,10.);
#13036=VECTOR('',#47259,10.);
#13037=VECTOR('',#47262,10.);
#13038=VECTOR('',#47265,10.);
#13039=VECTOR('',#47266,10.);
#13040=VECTOR('',#47267,10.);
#13041=VECTOR('',#47268,10.);
#13042=VECTOR('',#47269,10.);
#13043=VECTOR('',#47270,10.);
#13044=VECTOR('',#47271,10.);
#13045=VECTOR('',#47272,10.);
#13046=VECTOR('',#47273,10.);
#13047=VECTOR('',#47274,10.);
#13048=VECTOR('',#47283,46.9481408);
#13049=VECTOR('',#47290,46.9997605328678);
#13050=VECTOR('',#47299,10.);
#13051=VECTOR('',#47302,10.);
#13052=VECTOR('',#47303,10.);
#13053=VECTOR('',#47306,10.);
#13054=VECTOR('',#47307,10.);
#13055=VECTOR('',#47310,10.);
#13056=VECTOR('',#47311,10.);
#13057=VECTOR('',#47314,10.);
#13058=VECTOR('',#47315,10.);
#13059=VECTOR('',#47318,10.);
#13060=VECTOR('',#47319,10.);
#13061=VECTOR('',#47322,10.);
#13062=VECTOR('',#47327,10.);
#13063=VECTOR('',#47338,67.117943679437);
#13064=VECTOR('',#47343,30.1930816);
#13065=VECTOR('',#47346,28.921462932868);
#13066=VECTOR('',#47351,67.056);
#13067=VECTOR('',#47352,67.056);
#13068=VECTOR('',#47361,46.9481408);
#13069=VECTOR('',#47370,46.9997605328686);
#13070=VECTOR('',#47375,10.);
#13071=VECTOR('',#47376,10.);
#13072=VECTOR('',#47377,10.);
#13073=VECTOR('',#47378,10.);
#13074=VECTOR('',#47379,10.);
#13075=VECTOR('',#47380,10.);
#13076=VECTOR('',#47381,10.);
#13077=VECTOR('',#47382,10.);
#13078=VECTOR('',#47383,10.);
#13079=VECTOR('',#47384,10.);
#13080=VECTOR('',#47385,10.);
#13081=VECTOR('',#47386,10.);
#13082=VECTOR('',#47395,67.0291776);
#13083=VECTOR('',#47404,2.74750783999999);
#13084=VECTOR('',#47413,37.927515520559);
#13085=VECTOR('',#47418,10.);
#13086=VECTOR('',#47419,10.);
#13087=VECTOR('',#47422,10.);
#13088=VECTOR('',#47433,10.);
#13089=VECTOR('',#47436,10.);
#13090=VECTOR('',#47443,2.74750784);
#13091=VECTOR('',#47448,10.);
#13092=VECTOR('',#47449,10.);
#13093=VECTOR('',#47452,10.);
#13094=VECTOR('',#47453,10.);
#13095=VECTOR('',#47454,10.);
#13096=VECTOR('',#47455,10.);
#13097=VECTOR('',#47456,10.);
#13098=VECTOR('',#47457,10.);
#13099=VECTOR('',#47460,10.);
#13100=VECTOR('',#47461,10.);
#13101=VECTOR('',#47462,10.);
#13102=VECTOR('',#47465,10.);
#13103=VECTOR('',#47466,10.);
#13104=VECTOR('',#47469,10.);
#13105=VECTOR('',#47470,10.);
#13106=VECTOR('',#47473,10.);
#13107=VECTOR('',#47474,10.);
#13108=VECTOR('',#47477,10.);
#13109=VECTOR('',#47478,10.);
#13110=VECTOR('',#47481,10.);
#13111=VECTOR('',#47484,10.);
#13112=VECTOR('',#47485,10.);
#13113=VECTOR('',#47486,10.);
#13114=VECTOR('',#47487,10.);
#13115=VECTOR('',#47488,10.);
#13116=VECTOR('',#47489,10.);
#13117=VECTOR('',#47492,10.);
#13118=VECTOR('',#47493,10.);
#13119=VECTOR('',#47494,10.);
#13120=VECTOR('',#47497,10.);
#13121=VECTOR('',#47498,10.);
#13122=VECTOR('',#47501,10.);
#13123=VECTOR('',#47502,10.);
#13124=VECTOR('',#47505,10.);
#13125=VECTOR('',#47506,10.);
#13126=VECTOR('',#47509,10.);
#13127=VECTOR('',#47510,10.);
#13128=VECTOR('',#47513,10.);
#13129=VECTOR('',#47524,3.2861910399999);
#13130=VECTOR('',#47527,3.3528);
#13131=VECTOR('',#47534,2.74142809599801);
#13132=VECTOR('',#47549,3.28619103999997);
#13133=VECTOR('',#47552,10.);
#13134=VECTOR('',#47553,10.);
#13135=VECTOR('',#47554,10.);
#13136=VECTOR('',#47555,10.);
#13137=VECTOR('',#47556,10.);
#13138=VECTOR('',#47557,10.);
#13139=VECTOR('',#47560,10.);
#13140=VECTOR('',#47561,10.);
#13141=VECTOR('',#47562,10.);
#13142=VECTOR('',#47565,10.);
#13143=VECTOR('',#47566,10.);
#13144=VECTOR('',#47569,10.);
#13145=VECTOR('',#47570,10.);
#13146=VECTOR('',#47573,10.);
#13147=VECTOR('',#47574,10.);
#13148=VECTOR('',#47577,10.);
#13149=VECTOR('',#47578,10.);
#13150=VECTOR('',#47581,10.);
#13151=VECTOR('',#47584,10.);
#13152=VECTOR('',#47585,10.);
#13153=VECTOR('',#47586,10.);
#13154=VECTOR('',#47587,10.);
#13155=VECTOR('',#47588,10.);
#13156=VECTOR('',#47589,9.99999999999999);
#13157=VECTOR('',#47592,10.);
#13158=VECTOR('',#47593,10.);
#13159=VECTOR('',#47594,10.);
#13160=VECTOR('',#47597,10.);
#13161=VECTOR('',#47598,10.);
#13162=VECTOR('',#47601,10.);
#13163=VECTOR('',#47602,10.);
#13164=VECTOR('',#47605,10.);
#13165=VECTOR('',#47606,10.);
#13166=VECTOR('',#47609,10.);
#13167=VECTOR('',#47610,10.);
#13168=VECTOR('',#47613,10.);
#13169=VECTOR('',#47624,3.28619104000002);
#13170=VECTOR('',#47627,3.35280000000001);
#13171=VECTOR('',#47634,2.74142809600037);
#13172=VECTOR('',#47649,3.28619104000001);
#13173=VECTOR('',#47652,3.3528);
#13174=VECTOR('',#47655,2.74142809599998);
#13175=VECTOR('',#47662,2.74750783999998);
#13176=VECTOR('',#47665,2.74750784000003);
#13177=VECTOR('',#47672,2.74142809599988);
#13178=VECTOR('',#47675,3.3528);
#13179=VECTOR('',#47682,37.9894592000001);
#13180=VECTOR('',#47687,37.0614901167744);
#13181=VECTOR('',#47698,37.9894592000001);
#13182=VECTOR('',#47709,46.9481408);
#13183=VECTOR('',#47712,37.9894592000001);
#13184=VECTOR('',#47723,46.9481408);
#13185=VECTOR('',#47728,10.);
#13186=VECTOR('',#47731,10.);
#13187=VECTOR('',#47734,10.);
#13188=VECTOR('',#47737,10.);
#13189=VECTOR('',#47740,10.);
#13190=VECTOR('',#47743,10.);
#13191=VECTOR('',#47748,10.);
#13192=VECTOR('',#47749,10.);
#13193=VECTOR('',#47752,10.);
#13194=VECTOR('',#47765,10.);
#13195=VECTOR('',#47768,10.);
#13196=VECTOR('',#47771,10.);
#13197=VECTOR('',#47778,10.);
#13198=VECTOR('',#47781,10.);
#13199=VECTOR('',#47784,10.);
#13200=VECTOR('',#47787,10.);
#13201=VECTOR('',#47790,10.);
#13202=VECTOR('',#47793,10.);
#13203=VECTOR('',#47798,10.);
#13204=VECTOR('',#47799,10.);
#13205=VECTOR('',#47802,10.);
#13206=VECTOR('',#47815,10.);
#13207=VECTOR('',#47818,10.);
#13208=VECTOR('',#47821,10.);
#13209=VECTOR('',#47840,2.74750784);
#13210=VECTOR('',#47847,2.74750784000001);
#13211=VECTOR('',#47854,21.82583392);
#13212=VECTOR('',#47859,3.63219999999997);
#13213=VECTOR('',#47866,3.63219999999997);
#13214=VECTOR('',#47873,3.63219999999999);
#13215=VECTOR('',#47880,3.63219999999999);
#13216=VECTOR('',#47889,9.99999999999999);
#13217=VECTOR('',#47896,10.);
#13218=VECTOR('',#47901,10.);
#13219=VECTOR('',#47902,10.);
#13220=VECTOR('',#47903,10.);
#13221=VECTOR('',#47904,10.);
#13222=VECTOR('',#47909,10.);
#13223=VECTOR('',#47916,10.);
#13224=VECTOR('',#47923,10.);
#13225=VECTOR('',#47928,10.);
#13226=VECTOR('',#47929,10.);
#13227=VECTOR('',#47930,10.);
#13228=VECTOR('',#47935,10.);
#13229=VECTOR('',#47942,10.);
#13230=VECTOR('',#47955,10.);
#13231=VECTOR('',#47956,10.);
#13232=VECTOR('',#47957,10.);
#13233=VECTOR('',#47958,10.);
#13234=VECTOR('',#47963,10.);
#13235=VECTOR('',#47970,10.);
#13236=VECTOR('',#47977,10.);
#13237=VECTOR('',#47982,10.);
#13238=VECTOR('',#47983,10.);
#13239=VECTOR('',#47984,10.);
#13240=VECTOR('',#47989,10.);
#13241=VECTOR('',#47996,10.);
#13242=VECTOR('',#48009,10.);
#13243=VECTOR('',#48010,10.);
#13244=VECTOR('',#48011,10.);
#13245=VECTOR('',#48012,10.);
#13246=VECTOR('',#48017,10.);
#13247=VECTOR('',#48024,10.);
#13248=VECTOR('',#48031,10.);
#13249=VECTOR('',#48036,10.);
#13250=VECTOR('',#48037,10.);
#13251=VECTOR('',#48038,10.);
#13252=VECTOR('',#48043,10.);
#13253=VECTOR('',#48050,10.);
#13254=VECTOR('',#48063,3.63219999999999);
#13255=VECTOR('',#48068,3.63220000000001);
#13256=VECTOR('',#48073,3.63220000000001);
#13257=VECTOR('',#48088,10.);
#13258=VECTOR('',#48101,10.);
#13259=VECTOR('',#48114,10.);
#13260=VECTOR('',#48117,10.);
#13261=VECTOR('',#48118,10.);
#13262=VECTOR('',#48121,10.);
#13263=VECTOR('',#48122,10.);
#13264=VECTOR('',#48127,10.);
#13265=VECTOR('',#48130,10.);
#13266=VECTOR('',#48131,10.);
#13267=VECTOR('',#48134,10.);
#13268=VECTOR('',#48137,10.);
#13269=VECTOR('',#48140,10.);
#13270=VECTOR('',#48141,10.);
#13271=VECTOR('',#48144,10.);
#13272=VECTOR('',#48151,58.1057817920919);
#13273=VECTOR('',#48158,10.);
#13274=VECTOR('',#48159,10.);
#13275=VECTOR('',#48160,10.);
#13276=VECTOR('',#48163,10.);
#13277=VECTOR('',#48164,10.);
#13278=VECTOR('',#48165,10.);
#13279=VECTOR('',#48168,10.);
#13280=VECTOR('',#48169,10.);
#13281=VECTOR('',#48170,10.);
#13282=VECTOR('',#48173,10.);
#13283=VECTOR('',#48174,10.);
#13284=VECTOR('',#48175,10.);
#13285=VECTOR('',#48178,10.);
#13286=VECTOR('',#48179,10.);
#13287=VECTOR('',#48180,10.);
#13288=VECTOR('',#48181,10.);
#13289=VECTOR('',#48182,10.);
#13290=VECTOR('',#48183,10.);
#13291=VECTOR('',#48184,10.);
#13292=VECTOR('',#48187,10.);
#13293=VECTOR('',#48192,10.);
#13294=VECTOR('',#48193,10.);
#13295=VECTOR('',#48194,10.);
#13296=VECTOR('',#48195,10.);
#13297=VECTOR('',#48196,10.);
#13298=VECTOR('',#48197,10.);
#13299=VECTOR('',#48200,10.);
#13300=VECTOR('',#48205,10.);
#13301=VECTOR('',#48206,10.);
#13302=VECTOR('',#48207,10.);
#13303=VECTOR('',#48208,10.);
#13304=VECTOR('',#48209,10.);
#13305=VECTOR('',#48210,10.);
#13306=VECTOR('',#48211,10.);
#13307=VECTOR('',#48216,10.);
#13308=VECTOR('',#48221,10.);
#13309=VECTOR('',#48224,10.);
#13310=VECTOR('',#48227,10.);
#13311=VECTOR('',#48228,10.);
#13312=VECTOR('',#48229,10.);
#13313=VECTOR('',#48230,10.);
#13314=VECTOR('',#48231,10.);
#13315=VECTOR('',#48232,10.);
#13316=VECTOR('',#48239,10.);
#13317=VECTOR('',#48240,10.);
#13318=VECTOR('',#48243,10.);
#13319=VECTOR('',#48244,10.);
#13320=VECTOR('',#48247,10.);
#13321=VECTOR('',#48248,10.);
#13322=VECTOR('',#48251,10.);
#13323=VECTOR('',#48252,10.);
#13324=VECTOR('',#48257,10.);
#13325=VECTOR('',#48258,10.);
#13326=VECTOR('',#48263,10.);
#13327=VECTOR('',#48266,10.);
#13328=VECTOR('',#48269,10.);
#13329=VECTOR('',#48272,10.);
#13330=VECTOR('',#48277,10.);
#13331=VECTOR('',#48280,10.);
#13332=VECTOR('',#48285,10.);
#13333=VECTOR('',#48288,10.);
#13334=VECTOR('',#48305,10.);
#13335=VECTOR('',#48308,10.);
#13336=VECTOR('',#48311,10.);
#13337=VECTOR('',#48312,10.);
#13338=VECTOR('',#48313,10.);
#13339=VECTOR('',#48318,10.);
#13340=VECTOR('',#48325,10.);
#13341=VECTOR('',#48332,10.);
#13342=VECTOR('',#48337,10.);
#13343=VECTOR('',#48338,10.);
#13344=VECTOR('',#48339,10.);
#13345=VECTOR('',#48344,10.);
#13346=VECTOR('',#48357,10.);
#13347=VECTOR('',#48358,10.);
#13348=VECTOR('',#48359,10.);
#13349=VECTOR('',#48360,10.);
#13350=VECTOR('',#48365,10.);
#13351=VECTOR('',#48372,10.);
#13352=VECTOR('',#48379,10.);
#13353=VECTOR('',#48384,10.);
#13354=VECTOR('',#48385,10.);
#13355=VECTOR('',#48386,10.);
#13356=VECTOR('',#48391,10.);
#13357=VECTOR('',#48398,10.);
#13358=VECTOR('',#48413,10.);
#13359=VECTOR('',#48416,10.);
#13360=VECTOR('',#48421,10.);
#13361=VECTOR('',#48426,10.);
#13362=VECTOR('',#48427,10.);
#13363=VECTOR('',#48428,10.);
#13364=VECTOR('',#48433,10.);
#13365=VECTOR('',#48440,10.);
#13366=VECTOR('',#48447,10.);
#13367=VECTOR('',#48452,10.);
#13368=VECTOR('',#48453,10.);
#13369=VECTOR('',#48454,10.);
#13370=VECTOR('',#48467,10.);
#13371=VECTOR('',#48470,10.);
#13372=VECTOR('',#48475,10.);
#13373=VECTOR('',#48480,10.);
#13374=VECTOR('',#48481,10.);
#13375=VECTOR('',#48482,10.);
#13376=VECTOR('',#48487,10.);
#13377=VECTOR('',#48494,10.);
#13378=VECTOR('',#48501,10.);
#13379=VECTOR('',#48506,10.);
#13380=VECTOR('',#48507,10.);
#13381=VECTOR('',#48508,10.);
#13382=VECTOR('',#48521,10.);
#13383=VECTOR('',#48522,10.);
#13384=VECTOR('',#48527,10.);
#13385=VECTOR('',#48530,10.);
#13386=VECTOR('',#48531,10.);
#13387=VECTOR('',#48536,10.);
#13388=VECTOR('',#48541,10.);
#13389=VECTOR('',#48546,10.);
#13390=VECTOR('',#48551,10.);
#13391=VECTOR('',#48554,9.99999999999999);
#13392=VECTOR('',#48563,10.);
#13393=VECTOR('',#48564,10.);
#13394=VECTOR('',#48565,10.);
#13395=VECTOR('',#48566,10.);
#13396=VECTOR('',#48567,10.);
#13397=VECTOR('',#48568,10.);
#13398=VECTOR('',#48569,10.);
#13399=VECTOR('',#48570,10.);
#13400=VECTOR('',#48573,10.);
#13401=VECTOR('',#48574,10.);
#13402=VECTOR('',#48577,9.99999999999999);
#13403=VECTOR('',#48578,10.);
#13404=VECTOR('',#48583,10.);
#13405=VECTOR('',#48584,10.);
#13406=VECTOR('',#48587,10.);
#13407=VECTOR('',#48592,10.);
#13408=VECTOR('',#48605,4.98002560000028);
#13409=VECTOR('',#48610,5.02472959999993);
#13410=VECTOR('',#48617,5.01355360000019);
#13411=VECTOR('',#48620,10.);
#13412=VECTOR('',#48621,10.);
#13413=VECTOR('',#48622,10.);
#13414=VECTOR('',#48623,10.);
#13415=VECTOR('',#48626,10.);
#13416=VECTOR('',#48627,10.);
#13417=VECTOR('',#48628,10.);
#13418=VECTOR('',#48631,10.);
#13419=VECTOR('',#48632,10.);
#13420=VECTOR('',#48633,10.);
#13421=VECTOR('',#48636,10.);
#13422=VECTOR('',#48637,10.);
#13423=VECTOR('',#48638,10.);
#13424=VECTOR('',#48641,10.);
#13425=VECTOR('',#48642,10.);
#13426=VECTOR('',#48643,10.);
#13427=VECTOR('',#48646,10.);
#13428=VECTOR('',#48649,10.);
#15841=VERTEX_POINT('',#58609);
#15842=VERTEX_POINT('',#58610);
#15843=VERTEX_POINT('',#58613);
#15844=VERTEX_POINT('',#58618);
#15845=VERTEX_POINT('',#58619);
#15846=VERTEX_POINT('',#58621);
#15847=VERTEX_POINT('',#58627);
#15848=VERTEX_POINT('',#58629);
#15849=VERTEX_POINT('',#58633);
#15850=VERTEX_POINT('',#58636);
#15851=VERTEX_POINT('',#58641);
#15852=VERTEX_POINT('',#58642);
#15853=VERTEX_POINT('',#58645);
#15854=VERTEX_POINT('',#58650);
#15855=VERTEX_POINT('',#58651);
#15856=VERTEX_POINT('',#58653);
#15857=VERTEX_POINT('',#58659);
#15858=VERTEX_POINT('',#58661);
#15859=VERTEX_POINT('',#58665);
#15860=VERTEX_POINT('',#58668);
#15861=VERTEX_POINT('',#58673);
#15862=VERTEX_POINT('',#58674);
#15863=VERTEX_POINT('',#58676);
#15864=VERTEX_POINT('',#58682);
#15865=VERTEX_POINT('',#58683);
#15866=VERTEX_POINT('',#58688);
#15867=VERTEX_POINT('',#58691);
#15868=VERTEX_POINT('',#58693);
#15869=VERTEX_POINT('',#58697);
#15870=VERTEX_POINT('',#58700);
#15871=VERTEX_POINT('',#58705);
#15872=VERTEX_POINT('',#58707);
#15873=VERTEX_POINT('',#58711);
#15874=VERTEX_POINT('',#58714);
#15875=VERTEX_POINT('',#58719);
#15876=VERTEX_POINT('',#58720);
#15877=VERTEX_POINT('',#58723);
#15878=VERTEX_POINT('',#58728);
#15879=VERTEX_POINT('',#58729);
#15880=VERTEX_POINT('',#58734);
#15881=VERTEX_POINT('',#58737);
#15882=VERTEX_POINT('',#58739);
#15883=VERTEX_POINT('',#58743);
#15884=VERTEX_POINT('',#58746);
#15885=VERTEX_POINT('',#58751);
#15886=VERTEX_POINT('',#58752);
#15887=VERTEX_POINT('',#58755);
#15888=VERTEX_POINT('',#58760);
#15889=VERTEX_POINT('',#58761);
#15890=VERTEX_POINT('',#58766);
#15891=VERTEX_POINT('',#58769);
#15892=VERTEX_POINT('',#58770);
#15893=VERTEX_POINT('',#58772);
#15894=VERTEX_POINT('',#58774);
#15895=VERTEX_POINT('',#58776);
#15896=VERTEX_POINT('',#58778);
#15897=VERTEX_POINT('',#58782);
#15898=VERTEX_POINT('',#58784);
#15899=VERTEX_POINT('',#58786);
#15900=VERTEX_POINT('',#58788);
#15901=VERTEX_POINT('',#58790);
#15902=VERTEX_POINT('',#58792);
#15903=VERTEX_POINT('',#58794);
#15904=VERTEX_POINT('',#58796);
#15905=VERTEX_POINT('',#58798);
#15906=VERTEX_POINT('',#58800);
#15907=VERTEX_POINT('',#58806);
#15908=VERTEX_POINT('',#58807);
#15909=VERTEX_POINT('',#58809);
#15910=VERTEX_POINT('',#58811);
#15911=VERTEX_POINT('',#58815);
#15912=VERTEX_POINT('',#58817);
#15913=VERTEX_POINT('',#58821);
#15914=VERTEX_POINT('',#58822);
#15915=VERTEX_POINT('',#58824);
#15916=VERTEX_POINT('',#58826);
#15917=VERTEX_POINT('',#58830);
#15918=VERTEX_POINT('',#58832);
#15919=VERTEX_POINT('',#58834);
#15920=VERTEX_POINT('',#58836);
#15921=VERTEX_POINT('',#58840);
#15922=VERTEX_POINT('',#58843);
#15923=VERTEX_POINT('',#58847);
#15924=VERTEX_POINT('',#58849);
#15925=VERTEX_POINT('',#58854);
#15926=VERTEX_POINT('',#58856);
#15927=VERTEX_POINT('',#58858);
#15928=VERTEX_POINT('',#58860);
#15929=VERTEX_POINT('',#58862);
#15930=VERTEX_POINT('',#58866);
#15931=VERTEX_POINT('',#58870);
#15932=VERTEX_POINT('',#58872);
#15933=VERTEX_POINT('',#58874);
#15934=VERTEX_POINT('',#58876);
#15935=VERTEX_POINT('',#58879);
#15936=VERTEX_POINT('',#58881);
#15937=VERTEX_POINT('',#58883);
#15938=VERTEX_POINT('',#58885);
#15939=VERTEX_POINT('',#58888);
#15940=VERTEX_POINT('',#58891);
#15941=VERTEX_POINT('',#58893);
#15942=VERTEX_POINT('',#58895);
#15943=VERTEX_POINT('',#58902);
#15944=VERTEX_POINT('',#58904);
#15945=VERTEX_POINT('',#58906);
#15946=VERTEX_POINT('',#58908);
#15947=VERTEX_POINT('',#58910);
#15948=VERTEX_POINT('',#58913);
#15949=VERTEX_POINT('',#58915);
#15950=VERTEX_POINT('',#58917);
#15951=VERTEX_POINT('',#58920);
#15952=VERTEX_POINT('',#58922);
#15953=VERTEX_POINT('',#58926);
#15954=VERTEX_POINT('',#58930);
#15955=VERTEX_POINT('',#58932);
#15956=VERTEX_POINT('',#58934);
#15957=VERTEX_POINT('',#58936);
#15958=VERTEX_POINT('',#58938);
#15959=VERTEX_POINT('',#58940);
#15960=VERTEX_POINT('',#58942);
#15961=VERTEX_POINT('',#58944);
#15962=VERTEX_POINT('',#58946);
#15963=VERTEX_POINT('',#58950);
#15964=VERTEX_POINT('',#58952);
#15965=VERTEX_POINT('',#58956);
#15966=VERTEX_POINT('',#58960);
#15967=VERTEX_POINT('',#58964);
#15968=VERTEX_POINT('',#58966);
#15969=VERTEX_POINT('',#58970);
#15970=VERTEX_POINT('',#58972);
#15971=VERTEX_POINT('',#58974);
#15972=VERTEX_POINT('',#58980);
#15973=VERTEX_POINT('',#58982);
#15974=VERTEX_POINT('',#58984);
#15975=VERTEX_POINT('',#58986);
#15976=VERTEX_POINT('',#58991);
#15977=VERTEX_POINT('',#58993);
#15978=VERTEX_POINT('',#58995);
#15979=VERTEX_POINT('',#58997);
#15980=VERTEX_POINT('',#58999);
#15981=VERTEX_POINT('',#59001);
#15982=VERTEX_POINT('',#59008);
#15983=VERTEX_POINT('',#59009);
#15984=VERTEX_POINT('',#59011);
#15985=VERTEX_POINT('',#59013);
#15986=VERTEX_POINT('',#59016);
#15987=VERTEX_POINT('',#59018);
#15988=VERTEX_POINT('',#59020);
#15989=VERTEX_POINT('',#59022);
#15990=VERTEX_POINT('',#59026);
#15991=VERTEX_POINT('',#59027);
#15992=VERTEX_POINT('',#59029);
#15993=VERTEX_POINT('',#59032);
#15994=VERTEX_POINT('',#59034);
#15995=VERTEX_POINT('',#59036);
#15996=VERTEX_POINT('',#59038);
#15997=VERTEX_POINT('',#59042);
#15998=VERTEX_POINT('',#59048);
#15999=VERTEX_POINT('',#59049);
#16000=VERTEX_POINT('',#59051);
#16001=VERTEX_POINT('',#59053);
#16002=VERTEX_POINT('',#59057);
#16003=VERTEX_POINT('',#59059);
#16004=VERTEX_POINT('',#59063);
#16005=VERTEX_POINT('',#59065);
#16006=VERTEX_POINT('',#59071);
#16007=VERTEX_POINT('',#59075);
#16008=VERTEX_POINT('',#59082);
#16009=VERTEX_POINT('',#59085);
#16010=VERTEX_POINT('',#59086);
#16011=VERTEX_POINT('',#59089);
#16012=VERTEX_POINT('',#59093);
#16013=VERTEX_POINT('',#59094);
#16014=VERTEX_POINT('',#59097);
#16015=VERTEX_POINT('',#59101);
#16016=VERTEX_POINT('',#59102);
#16017=VERTEX_POINT('',#59105);
#16018=VERTEX_POINT('',#59109);
#16019=VERTEX_POINT('',#59110);
#16020=VERTEX_POINT('',#59113);
#16021=VERTEX_POINT('',#59118);
#16022=VERTEX_POINT('',#59120);
#16023=VERTEX_POINT('',#59122);
#16024=VERTEX_POINT('',#59128);
#16025=VERTEX_POINT('',#59130);
#16026=VERTEX_POINT('',#59135);
#16027=VERTEX_POINT('',#59138);
#16028=VERTEX_POINT('',#59140);
#16029=VERTEX_POINT('',#59144);
#16030=VERTEX_POINT('',#59145);
#16031=VERTEX_POINT('',#59147);
#16032=VERTEX_POINT('',#59149);
#16033=VERTEX_POINT('',#59153);
#16034=VERTEX_POINT('',#59155);
#16035=VERTEX_POINT('',#59160);
#16036=VERTEX_POINT('',#59161);
#16037=VERTEX_POINT('',#59165);
#16038=VERTEX_POINT('',#59167);
#16039=VERTEX_POINT('',#59171);
#16040=VERTEX_POINT('',#59173);
#16041=VERTEX_POINT('',#59177);
#16042=VERTEX_POINT('',#59178);
#16043=VERTEX_POINT('',#59182);
#16044=VERTEX_POINT('',#59187);
#16045=VERTEX_POINT('',#59191);
#16046=VERTEX_POINT('',#59192);
#16047=VERTEX_POINT('',#59196);
#16048=VERTEX_POINT('',#59201);
#16049=VERTEX_POINT('',#59205);
#16050=VERTEX_POINT('',#59206);
#16051=VERTEX_POINT('',#59210);
#16052=VERTEX_POINT('',#59215);
#16053=VERTEX_POINT('',#59219);
#16054=VERTEX_POINT('',#59227);
#16055=VERTEX_POINT('',#59228);
#16056=VERTEX_POINT('',#59232);
#16057=VERTEX_POINT('',#59238);
#16058=VERTEX_POINT('',#59247);
#16059=VERTEX_POINT('',#59257);
#16060=VERTEX_POINT('',#59258);
#16061=VERTEX_POINT('',#59262);
#16062=VERTEX_POINT('',#59264);
#16063=VERTEX_POINT('',#59268);
#16064=VERTEX_POINT('',#59270);
#16065=VERTEX_POINT('',#59274);
#16066=VERTEX_POINT('',#59275);
#16067=VERTEX_POINT('',#59279);
#16068=VERTEX_POINT('',#59284);
#16069=VERTEX_POINT('',#59288);
#16070=VERTEX_POINT('',#59289);
#16071=VERTEX_POINT('',#59293);
#16072=VERTEX_POINT('',#59298);
#16073=VERTEX_POINT('',#59302);
#16074=VERTEX_POINT('',#59303);
#16075=VERTEX_POINT('',#59307);
#16076=VERTEX_POINT('',#59312);
#16077=VERTEX_POINT('',#59316);
#16078=VERTEX_POINT('',#59324);
#16079=VERTEX_POINT('',#59325);
#16080=VERTEX_POINT('',#59329);
#16081=VERTEX_POINT('',#59335);
#16082=VERTEX_POINT('',#59344);
#16083=VERTEX_POINT('',#59354);
#16084=VERTEX_POINT('',#59358);
#16085=VERTEX_POINT('',#59360);
#16086=VERTEX_POINT('',#59364);
#16087=VERTEX_POINT('',#59368);
#16088=VERTEX_POINT('',#59372);
#16089=VERTEX_POINT('',#59376);
#16090=VERTEX_POINT('',#59393);
#16091=VERTEX_POINT('',#59394);
#16092=VERTEX_POINT('',#59396);
#16093=VERTEX_POINT('',#59398);
#16094=VERTEX_POINT('',#59400);
#16095=VERTEX_POINT('',#59402);
#16096=VERTEX_POINT('',#59406);
#16097=VERTEX_POINT('',#59407);
#16098=VERTEX_POINT('',#59412);
#16099=VERTEX_POINT('',#59416);
#16100=VERTEX_POINT('',#59420);
#16101=VERTEX_POINT('',#59424);
#16102=VERTEX_POINT('',#59433);
#16103=VERTEX_POINT('',#59434);
#16104=VERTEX_POINT('',#59436);
#16105=VERTEX_POINT('',#59438);
#16106=VERTEX_POINT('',#59440);
#16107=VERTEX_POINT('',#59442);
#16108=VERTEX_POINT('',#59446);
#16109=VERTEX_POINT('',#59447);
#16110=VERTEX_POINT('',#59452);
#16111=VERTEX_POINT('',#59456);
#16112=VERTEX_POINT('',#59460);
#16113=VERTEX_POINT('',#59464);
#16114=VERTEX_POINT('',#59473);
#16115=VERTEX_POINT('',#59477);
#16116=VERTEX_POINT('',#59483);
#16117=VERTEX_POINT('',#59488);
#16118=VERTEX_POINT('',#59489);
#16119=VERTEX_POINT('',#59491);
#16120=VERTEX_POINT('',#59495);
#16121=VERTEX_POINT('',#59497);
#16122=VERTEX_POINT('',#59501);
#16123=VERTEX_POINT('',#59505);
#16124=VERTEX_POINT('',#59506);
#16125=VERTEX_POINT('',#59508);
#16126=VERTEX_POINT('',#59512);
#16127=VERTEX_POINT('',#59514);
#16128=VERTEX_POINT('',#59518);
#16129=VERTEX_POINT('',#59522);
#16130=VERTEX_POINT('',#59523);
#16131=VERTEX_POINT('',#59525);
#16132=VERTEX_POINT('',#59529);
#16133=VERTEX_POINT('',#59531);
#16134=VERTEX_POINT('',#59535);
#16135=VERTEX_POINT('',#59539);
#16136=VERTEX_POINT('',#59540);
#16137=VERTEX_POINT('',#59543);
#16138=VERTEX_POINT('',#59547);
#16139=VERTEX_POINT('',#59549);
#16140=VERTEX_POINT('',#59553);
#16141=VERTEX_POINT('',#59556);
#16142=VERTEX_POINT('',#59557);
#16143=VERTEX_POINT('',#59560);
#16144=VERTEX_POINT('',#59564);
#16145=VERTEX_POINT('',#59566);
#16146=VERTEX_POINT('',#59570);
#16147=VERTEX_POINT('',#59573);
#16148=VERTEX_POINT('',#59574);
#16149=VERTEX_POINT('',#59577);
#16150=VERTEX_POINT('',#59581);
#16151=VERTEX_POINT('',#59583);
#16152=VERTEX_POINT('',#59587);
#16153=VERTEX_POINT('',#59590);
#16154=VERTEX_POINT('',#59591);
#16155=VERTEX_POINT('',#59594);
#16156=VERTEX_POINT('',#59598);
#16157=VERTEX_POINT('',#59600);
#16158=VERTEX_POINT('',#59604);
#16159=VERTEX_POINT('',#59607);
#16160=VERTEX_POINT('',#59610);
#16161=VERTEX_POINT('',#59613);
#16162=VERTEX_POINT('',#59616);
#16163=VERTEX_POINT('',#59619);
#16164=VERTEX_POINT('',#59622);
#16165=VERTEX_POINT('',#59625);
#16166=VERTEX_POINT('',#59628);
#16167=VERTEX_POINT('',#59631);
#16168=VERTEX_POINT('',#59633);
#16169=VERTEX_POINT('',#59637);
#16170=VERTEX_POINT('',#59641);
#16171=VERTEX_POINT('',#59643);
#16172=VERTEX_POINT('',#59647);
#16173=VERTEX_POINT('',#59651);
#16174=VERTEX_POINT('',#59655);
#16175=VERTEX_POINT('',#59659);
#16176=VERTEX_POINT('',#59665);
#16177=VERTEX_POINT('',#59668);
#16178=VERTEX_POINT('',#59669);
#16179=VERTEX_POINT('',#59671);
#16180=VERTEX_POINT('',#59673);
#16181=VERTEX_POINT('',#59675);
#16182=VERTEX_POINT('',#59677);
#16183=VERTEX_POINT('',#59679);
#16184=VERTEX_POINT('',#59681);
#16185=VERTEX_POINT('',#59685);
#16186=VERTEX_POINT('',#59687);
#16187=VERTEX_POINT('',#59690);
#16188=VERTEX_POINT('',#59694);
#16189=VERTEX_POINT('',#59695);
#16190=VERTEX_POINT('',#59697);
#16191=VERTEX_POINT('',#59705);
#16192=VERTEX_POINT('',#59709);
#16193=VERTEX_POINT('',#59713);
#16194=VERTEX_POINT('',#59717);
#16195=VERTEX_POINT('',#59721);
#16196=VERTEX_POINT('',#59732);
#16197=VERTEX_POINT('',#59733);
#16198=VERTEX_POINT('',#59736);
#16199=VERTEX_POINT('',#59740);
#16200=VERTEX_POINT('',#59742);
#16201=VERTEX_POINT('',#59751);
#16202=VERTEX_POINT('',#59820);
#16203=VERTEX_POINT('',#59829);
#16204=VERTEX_POINT('',#59831);
#16205=VERTEX_POINT('',#59835);
#16206=VERTEX_POINT('',#59836);
#16207=VERTEX_POINT('',#59839);
#16208=VERTEX_POINT('',#59843);
#16209=VERTEX_POINT('',#59844);
#16210=VERTEX_POINT('',#59846);
#16211=VERTEX_POINT('',#59848);
#16212=VERTEX_POINT('',#59850);
#16213=VERTEX_POINT('',#59852);
#16214=VERTEX_POINT('',#59855);
#16215=VERTEX_POINT('',#59856);
#16216=VERTEX_POINT('',#59858);
#16217=VERTEX_POINT('',#59860);
#16218=VERTEX_POINT('',#59862);
#16219=VERTEX_POINT('',#59864);
#16220=VERTEX_POINT('',#59868);
#16221=VERTEX_POINT('',#59871);
#16222=VERTEX_POINT('',#59876);
#16223=VERTEX_POINT('',#59877);
#16224=VERTEX_POINT('',#59880);
#16225=VERTEX_POINT('',#59884);
#16226=VERTEX_POINT('',#59885);
#16227=VERTEX_POINT('',#59888);
#16228=VERTEX_POINT('',#59892);
#16229=VERTEX_POINT('',#59893);
#16230=VERTEX_POINT('',#59895);
#16231=VERTEX_POINT('',#59897);
#16232=VERTEX_POINT('',#59901);
#16233=VERTEX_POINT('',#59902);
#16234=VERTEX_POINT('',#59913);
#16235=VERTEX_POINT('',#59916);
#16236=VERTEX_POINT('',#59918);
#16237=VERTEX_POINT('',#59921);
#16238=VERTEX_POINT('',#59956);
#16239=VERTEX_POINT('',#59992);
#16240=VERTEX_POINT('',#59993);
#16241=VERTEX_POINT('',#59996);
#16242=VERTEX_POINT('',#60003);
#16243=VERTEX_POINT('',#60004);
#16244=VERTEX_POINT('',#60006);
#16245=VERTEX_POINT('',#60008);
#16246=VERTEX_POINT('',#60010);
#16247=VERTEX_POINT('',#60012);
#16248=VERTEX_POINT('',#60016);
#16249=VERTEX_POINT('',#60017);
#16250=VERTEX_POINT('',#60022);
#16251=VERTEX_POINT('',#60026);
#16252=VERTEX_POINT('',#60030);
#16253=VERTEX_POINT('',#60034);
#16254=VERTEX_POINT('',#60040);
#16255=VERTEX_POINT('',#60041);
#16256=VERTEX_POINT('',#60043);
#16257=VERTEX_POINT('',#60045);
#16258=VERTEX_POINT('',#60047);
#16259=VERTEX_POINT('',#60049);
#16260=VERTEX_POINT('',#60053);
#16261=VERTEX_POINT('',#60054);
#16262=VERTEX_POINT('',#60059);
#16263=VERTEX_POINT('',#60063);
#16264=VERTEX_POINT('',#60067);
#16265=VERTEX_POINT('',#60071);
#16266=VERTEX_POINT('',#60077);
#16267=VERTEX_POINT('',#60080);
#16268=VERTEX_POINT('',#60081);
#16269=VERTEX_POINT('',#60086);
#16270=VERTEX_POINT('',#60123);
#16271=VERTEX_POINT('',#60124);
#16272=VERTEX_POINT('',#60127);
#16273=VERTEX_POINT('',#60132);
#16274=VERTEX_POINT('',#60135);
#16275=VERTEX_POINT('',#60136);
#16276=VERTEX_POINT('',#60141);
#16277=VERTEX_POINT('',#60142);
#16278=VERTEX_POINT('',#60144);
#16279=VERTEX_POINT('',#60146);
#16280=VERTEX_POINT('',#60148);
#16281=VERTEX_POINT('',#60150);
#16282=VERTEX_POINT('',#60154);
#16283=VERTEX_POINT('',#60155);
#16284=VERTEX_POINT('',#60160);
#16285=VERTEX_POINT('',#60164);
#16286=VERTEX_POINT('',#60168);
#16287=VERTEX_POINT('',#60172);
#16288=VERTEX_POINT('',#60178);
#16289=VERTEX_POINT('',#60179);
#16290=VERTEX_POINT('',#60181);
#16291=VERTEX_POINT('',#60183);
#16292=VERTEX_POINT('',#60185);
#16293=VERTEX_POINT('',#60187);
#16294=VERTEX_POINT('',#60191);
#16295=VERTEX_POINT('',#60192);
#16296=VERTEX_POINT('',#60197);
#16297=VERTEX_POINT('',#60201);
#16298=VERTEX_POINT('',#60205);
#16299=VERTEX_POINT('',#60209);
#16300=VERTEX_POINT('',#60215);
#16301=VERTEX_POINT('',#60218);
#16302=VERTEX_POINT('',#60219);
#16303=VERTEX_POINT('',#60224);
#16304=VERTEX_POINT('',#60261);
#16305=VERTEX_POINT('',#60262);
#16306=VERTEX_POINT('',#60265);
#16307=VERTEX_POINT('',#60270);
#16308=VERTEX_POINT('',#60273);
#16309=VERTEX_POINT('',#60274);
#16310=VERTEX_POINT('',#60279);
#16311=VERTEX_POINT('',#60316);
#16312=VERTEX_POINT('',#60325);
#16313=VERTEX_POINT('',#60330);
#16314=VERTEX_POINT('',#60367);
#16315=VERTEX_POINT('',#60368);
#16316=VERTEX_POINT('',#60371);
#16317=VERTEX_POINT('',#60388);
#16318=VERTEX_POINT('',#60392);
#16319=VERTEX_POINT('',#60395);
#16320=VERTEX_POINT('',#60400);
#16321=VERTEX_POINT('',#60405);
#16322=VERTEX_POINT('',#60410);
#16323=VERTEX_POINT('',#60411);
#16324=VERTEX_POINT('',#60413);
#16325=VERTEX_POINT('',#60415);
#16326=VERTEX_POINT('',#60417);
#16327=VERTEX_POINT('',#60419);
#16328=VERTEX_POINT('',#60421);
#16329=VERTEX_POINT('',#60423);
#16330=VERTEX_POINT('',#60425);
#16331=VERTEX_POINT('',#60427);
#16332=VERTEX_POINT('',#60429);
#16333=VERTEX_POINT('',#60431);
#16334=VERTEX_POINT('',#60435);
#16335=VERTEX_POINT('',#60443);
#16336=VERTEX_POINT('',#60447);
#16337=VERTEX_POINT('',#60454);
#16338=VERTEX_POINT('',#60463);
#16339=VERTEX_POINT('',#60476);
#16340=VERTEX_POINT('',#60495);
#16341=VERTEX_POINT('',#60496);
#16342=VERTEX_POINT('',#60498);
#16343=VERTEX_POINT('',#60500);
#16344=VERTEX_POINT('',#60502);
#16345=VERTEX_POINT('',#60504);
#16346=VERTEX_POINT('',#60506);
#16347=VERTEX_POINT('',#60508);
#16348=VERTEX_POINT('',#60510);
#16349=VERTEX_POINT('',#60512);
#16350=VERTEX_POINT('',#60514);
#16351=VERTEX_POINT('',#60516);
#16352=VERTEX_POINT('',#60520);
#16353=VERTEX_POINT('',#60528);
#16354=VERTEX_POINT('',#60532);
#16355=VERTEX_POINT('',#60539);
#16356=VERTEX_POINT('',#60548);
#16357=VERTEX_POINT('',#60561);
#16358=VERTEX_POINT('',#60580);
#16359=VERTEX_POINT('',#60583);
#16360=VERTEX_POINT('',#60586);
#16361=VERTEX_POINT('',#60589);
#16362=VERTEX_POINT('',#60591);
#16363=VERTEX_POINT('',#60595);
#16364=VERTEX_POINT('',#60597);
#16365=VERTEX_POINT('',#60601);
#16366=VERTEX_POINT('',#60605);
#16367=VERTEX_POINT('',#60607);
#16368=VERTEX_POINT('',#60611);
#16369=VERTEX_POINT('',#60613);
#16370=VERTEX_POINT('',#60617);
#16371=VERTEX_POINT('',#60619);
#16372=VERTEX_POINT('',#60623);
#16373=VERTEX_POINT('',#60625);
#16374=VERTEX_POINT('',#60629);
#16375=VERTEX_POINT('',#60630);
#16376=VERTEX_POINT('',#60632);
#16377=VERTEX_POINT('',#60634);
#16378=VERTEX_POINT('',#60636);
#16379=VERTEX_POINT('',#60638);
#16380=VERTEX_POINT('',#60640);
#16381=VERTEX_POINT('',#60642);
#16382=VERTEX_POINT('',#60646);
#16383=VERTEX_POINT('',#60647);
#16384=VERTEX_POINT('',#60649);
#16385=VERTEX_POINT('',#60651);
#16386=VERTEX_POINT('',#60655);
#16387=VERTEX_POINT('',#60657);
#16388=VERTEX_POINT('',#60661);
#16389=VERTEX_POINT('',#60663);
#16390=VERTEX_POINT('',#60667);
#16391=VERTEX_POINT('',#60669);
#16392=VERTEX_POINT('',#60673);
#16393=VERTEX_POINT('',#60675);
#16394=VERTEX_POINT('',#60679);
#16395=VERTEX_POINT('',#60681);
#16396=VERTEX_POINT('',#60685);
#16397=VERTEX_POINT('',#60687);
#16398=VERTEX_POINT('',#60695);
#16399=VERTEX_POINT('',#60696);
#16400=VERTEX_POINT('',#60698);
#16401=VERTEX_POINT('',#60700);
#16402=VERTEX_POINT('',#60704);
#16403=VERTEX_POINT('',#60706);
#16404=VERTEX_POINT('',#60710);
#16405=VERTEX_POINT('',#60712);
#16406=VERTEX_POINT('',#60716);
#16407=VERTEX_POINT('',#60718);
#16408=VERTEX_POINT('',#60722);
#16409=VERTEX_POINT('',#60724);
#16410=VERTEX_POINT('',#60728);
#16411=VERTEX_POINT('',#60730);
#16412=VERTEX_POINT('',#60734);
#16413=VERTEX_POINT('',#60736);
#16414=VERTEX_POINT('',#60744);
#16415=VERTEX_POINT('',#60745);
#16416=VERTEX_POINT('',#60747);
#16417=VERTEX_POINT('',#60749);
#16418=VERTEX_POINT('',#60753);
#16419=VERTEX_POINT('',#60755);
#16420=VERTEX_POINT('',#60759);
#16421=VERTEX_POINT('',#60761);
#16422=VERTEX_POINT('',#60765);
#16423=VERTEX_POINT('',#60767);
#16424=VERTEX_POINT('',#60771);
#16425=VERTEX_POINT('',#60773);
#16426=VERTEX_POINT('',#60777);
#16427=VERTEX_POINT('',#60779);
#16428=VERTEX_POINT('',#60783);
#16429=VERTEX_POINT('',#60785);
#16430=VERTEX_POINT('',#60793);
#16431=VERTEX_POINT('',#60797);
#16432=VERTEX_POINT('',#60801);
#16433=VERTEX_POINT('',#60805);
#16434=VERTEX_POINT('',#60806);
#16435=VERTEX_POINT('',#60808);
#16436=VERTEX_POINT('',#60810);
#16437=VERTEX_POINT('',#60816);
#16438=VERTEX_POINT('',#60817);
#16439=VERTEX_POINT('',#60819);
#16440=VERTEX_POINT('',#60821);
#16441=VERTEX_POINT('',#60827);
#16442=VERTEX_POINT('',#60828);
#16443=VERTEX_POINT('',#60830);
#16444=VERTEX_POINT('',#60832);
#16445=VERTEX_POINT('',#60838);
#16446=VERTEX_POINT('',#60839);
#16447=VERTEX_POINT('',#60841);
#16448=VERTEX_POINT('',#60843);
#16449=VERTEX_POINT('',#60845);
#16450=VERTEX_POINT('',#60847);
#16451=VERTEX_POINT('',#60851);
#16452=VERTEX_POINT('',#60852);
#16453=VERTEX_POINT('',#60854);
#16454=VERTEX_POINT('',#60856);
#16455=VERTEX_POINT('',#60858);
#16456=VERTEX_POINT('',#60860);
#16457=VERTEX_POINT('',#60864);
#16458=VERTEX_POINT('',#60865);
#16459=VERTEX_POINT('',#60867);
#16460=VERTEX_POINT('',#60869);
#16461=VERTEX_POINT('',#60871);
#16462=VERTEX_POINT('',#60873);
#16463=VERTEX_POINT('',#60876);
#16464=VERTEX_POINT('',#60879);
#16465=VERTEX_POINT('',#60881);
#16466=VERTEX_POINT('',#60883);
#16467=VERTEX_POINT('',#60887);
#16468=VERTEX_POINT('',#60889);
#16469=VERTEX_POINT('',#60893);
#16470=VERTEX_POINT('',#60895);
#16471=VERTEX_POINT('',#60899);
#16472=VERTEX_POINT('',#60901);
#16473=VERTEX_POINT('',#60905);
#16474=VERTEX_POINT('',#60907);
#16475=VERTEX_POINT('',#60911);
#16476=VERTEX_POINT('',#60913);
#16477=VERTEX_POINT('',#60916);
#16478=VERTEX_POINT('',#60918);
#16479=VERTEX_POINT('',#60923);
#16480=VERTEX_POINT('',#60927);
#16481=VERTEX_POINT('',#60930);
#16482=VERTEX_POINT('',#60932);
#16483=VERTEX_POINT('',#60937);
#16484=VERTEX_POINT('',#60941);
#16485=VERTEX_POINT('',#60944);
#16486=VERTEX_POINT('',#60946);
#16487=VERTEX_POINT('',#60948);
#16488=VERTEX_POINT('',#60950);
#16489=VERTEX_POINT('',#60954);
#16490=VERTEX_POINT('',#60956);
#16491=VERTEX_POINT('',#60960);
#16492=VERTEX_POINT('',#60961);
#16493=VERTEX_POINT('',#60963);
#16494=VERTEX_POINT('',#60965);
#16495=VERTEX_POINT('',#60967);
#16496=VERTEX_POINT('',#60970);
#16497=VERTEX_POINT('',#60972);
#16498=VERTEX_POINT('',#60974);
#16499=VERTEX_POINT('',#60981);
#16500=VERTEX_POINT('',#60983);
#16501=VERTEX_POINT('',#60985);
#16502=VERTEX_POINT('',#60988);
#16503=VERTEX_POINT('',#60990);
#16504=VERTEX_POINT('',#60993);
#16505=VERTEX_POINT('',#60995);
#16506=VERTEX_POINT('',#60998);
#16507=VERTEX_POINT('',#61002);
#16508=VERTEX_POINT('',#61006);
#16509=VERTEX_POINT('',#61032);
#16510=VERTEX_POINT('',#61033);
#16511=VERTEX_POINT('',#61035);
#16512=VERTEX_POINT('',#61037);
#16513=VERTEX_POINT('',#61041);
#16514=VERTEX_POINT('',#61043);
#16515=VERTEX_POINT('',#61047);
#16516=VERTEX_POINT('',#61049);
#16517=VERTEX_POINT('',#61053);
#16518=VERTEX_POINT('',#61055);
#16519=VERTEX_POINT('',#61059);
#16520=VERTEX_POINT('',#61061);
#16521=VERTEX_POINT('',#61065);
#16522=VERTEX_POINT('',#61067);
#16523=VERTEX_POINT('',#61071);
#16524=VERTEX_POINT('',#61073);
#16525=VERTEX_POINT('',#61081);
#16526=VERTEX_POINT('',#61082);
#16527=VERTEX_POINT('',#61084);
#16528=VERTEX_POINT('',#61086);
#16529=VERTEX_POINT('',#61090);
#16530=VERTEX_POINT('',#61092);
#16531=VERTEX_POINT('',#61096);
#16532=VERTEX_POINT('',#61098);
#16533=VERTEX_POINT('',#61102);
#16534=VERTEX_POINT('',#61104);
#16535=VERTEX_POINT('',#61108);
#16536=VERTEX_POINT('',#61110);
#16537=VERTEX_POINT('',#61114);
#16538=VERTEX_POINT('',#61116);
#16539=VERTEX_POINT('',#61120);
#16540=VERTEX_POINT('',#61122);
#16541=VERTEX_POINT('',#61130);
#16542=VERTEX_POINT('',#61131);
#16543=VERTEX_POINT('',#61133);
#16544=VERTEX_POINT('',#61135);
#16545=VERTEX_POINT('',#61139);
#16546=VERTEX_POINT('',#61141);
#16547=VERTEX_POINT('',#61145);
#16548=VERTEX_POINT('',#61147);
#16549=VERTEX_POINT('',#61151);
#16550=VERTEX_POINT('',#61153);
#16551=VERTEX_POINT('',#61157);
#16552=VERTEX_POINT('',#61159);
#16553=VERTEX_POINT('',#61163);
#16554=VERTEX_POINT('',#61165);
#16555=VERTEX_POINT('',#61169);
#16556=VERTEX_POINT('',#61171);
#16557=VERTEX_POINT('',#61179);
#16558=VERTEX_POINT('',#61180);
#16559=VERTEX_POINT('',#61182);
#16560=VERTEX_POINT('',#61184);
#16561=VERTEX_POINT('',#61188);
#16562=VERTEX_POINT('',#61190);
#16563=VERTEX_POINT('',#61194);
#16564=VERTEX_POINT('',#61196);
#16565=VERTEX_POINT('',#61200);
#16566=VERTEX_POINT('',#61202);
#16567=VERTEX_POINT('',#61206);
#16568=VERTEX_POINT('',#61208);
#16569=VERTEX_POINT('',#61212);
#16570=VERTEX_POINT('',#61214);
#16571=VERTEX_POINT('',#61218);
#16572=VERTEX_POINT('',#61220);
#16573=VERTEX_POINT('',#61228);
#16574=VERTEX_POINT('',#61229);
#16575=VERTEX_POINT('',#61234);
#16576=VERTEX_POINT('',#61238);
#16577=VERTEX_POINT('',#61242);
#16578=VERTEX_POINT('',#61246);
#16579=VERTEX_POINT('',#61250);
#16580=VERTEX_POINT('',#61254);
#16581=VERTEX_POINT('',#61260);
#16582=VERTEX_POINT('',#61264);
#16583=VERTEX_POINT('',#61265);
#16584=VERTEX_POINT('',#61267);
#16585=VERTEX_POINT('',#61269);
#16586=VERTEX_POINT('',#61271);
#16587=VERTEX_POINT('',#61273);
#16588=VERTEX_POINT('',#61275);
#16589=VERTEX_POINT('',#61277);
#16590=VERTEX_POINT('',#61299);
#16591=VERTEX_POINT('',#61300);
#16592=VERTEX_POINT('',#61303);
#16593=VERTEX_POINT('',#61307);
#16594=VERTEX_POINT('',#61309);
#16595=VERTEX_POINT('',#61315);
#16596=VERTEX_POINT('',#61316);
#16597=VERTEX_POINT('',#61318);
#16598=VERTEX_POINT('',#61320);
#16599=VERTEX_POINT('',#61324);
#16600=VERTEX_POINT('',#61326);
#16601=VERTEX_POINT('',#61330);
#16602=VERTEX_POINT('',#61332);
#16603=VERTEX_POINT('',#61336);
#16604=VERTEX_POINT('',#61338);
#16605=VERTEX_POINT('',#61342);
#16606=VERTEX_POINT('',#61344);
#20287=EDGE_CURVE('',#15841,#15842,#3847,.T.);
#20288=EDGE_CURVE('',#15842,#15841,#3848,.T.);
#20289=EDGE_CURVE('',#15842,#15843,#10200,.T.);
#20290=EDGE_CURVE('',#15843,#15843,#3849,.T.);
#20291=EDGE_CURVE('',#15844,#15845,#10201,.T.);
#20292=EDGE_CURVE('',#15846,#15845,#3850,.T.);
#20293=EDGE_CURVE('',#15845,#15846,#3851,.T.);
#20294=EDGE_CURVE('',#15846,#15841,#10202,.T.);
#20295=EDGE_CURVE('',#15847,#15847,#3852,.T.);
#20296=EDGE_CURVE('',#15847,#15848,#10203,.T.);
#20297=EDGE_CURVE('',#15848,#15848,#3853,.T.);
#20298=EDGE_CURVE('',#15849,#15849,#3854,.T.);
#20299=EDGE_CURVE('',#15850,#15850,#3855,.T.);
#20300=EDGE_CURVE('',#15849,#15850,#10204,.T.);
#20301=EDGE_CURVE('',#15851,#15852,#3856,.T.);
#20302=EDGE_CURVE('',#15852,#15851,#3857,.T.);
#20303=EDGE_CURVE('',#15852,#15853,#10205,.T.);
#20304=EDGE_CURVE('',#15853,#15853,#3858,.T.);
#20305=EDGE_CURVE('',#15854,#15855,#10206,.T.);
#20306=EDGE_CURVE('',#15856,#15855,#3859,.T.);
#20307=EDGE_CURVE('',#15855,#15856,#3860,.T.);
#20308=EDGE_CURVE('',#15856,#15851,#10207,.T.);
#20309=EDGE_CURVE('',#15857,#15857,#3861,.T.);
#20310=EDGE_CURVE('',#15857,#15858,#10208,.T.);
#20311=EDGE_CURVE('',#15858,#15858,#3862,.T.);
#20312=EDGE_CURVE('',#15859,#15859,#3863,.T.);
#20313=EDGE_CURVE('',#15860,#15860,#3864,.T.);
#20314=EDGE_CURVE('',#15859,#15860,#10209,.T.);
#20315=EDGE_CURVE('',#15861,#15862,#3865,.T.);
#20316=EDGE_CURVE('',#15861,#15863,#10210,.T.);
#20317=EDGE_CURVE('',#15863,#15863,#3866,.T.);
#20318=EDGE_CURVE('',#15862,#15861,#3867,.T.);
#20319=EDGE_CURVE('',#15864,#15865,#3868,.T.);
#20320=EDGE_CURVE('',#15865,#15864,#3869,.T.);
#20321=EDGE_CURVE('',#15864,#15862,#10211,.T.);
#20322=EDGE_CURVE('',#15866,#15865,#10212,.T.);
#20323=EDGE_CURVE('',#15867,#15867,#3870,.T.);
#20324=EDGE_CURVE('',#15867,#15868,#10213,.T.);
#20325=EDGE_CURVE('',#15868,#15868,#3871,.T.);
#20326=EDGE_CURVE('',#15869,#15869,#3872,.T.);
#20327=EDGE_CURVE('',#15870,#15870,#3873,.T.);
#20328=EDGE_CURVE('',#15870,#15869,#10214,.T.);
#20329=EDGE_CURVE('',#15871,#15871,#3874,.T.);
#20330=EDGE_CURVE('',#15871,#15872,#10215,.T.);
#20331=EDGE_CURVE('',#15872,#15872,#3875,.T.);
#20332=EDGE_CURVE('',#15873,#15873,#3876,.T.);
#20333=EDGE_CURVE('',#15873,#15874,#10216,.T.);
#20334=EDGE_CURVE('',#15874,#15874,#3877,.T.);
#20335=EDGE_CURVE('',#15875,#15876,#3878,.T.);
#20336=EDGE_CURVE('',#15876,#15875,#3879,.T.);
#20337=EDGE_CURVE('',#15876,#15877,#10217,.T.);
#20338=EDGE_CURVE('',#15877,#15877,#3880,.T.);
#20339=EDGE_CURVE('',#15878,#15879,#3881,.T.);
#20340=EDGE_CURVE('',#15879,#15878,#3882,.T.);
#20341=EDGE_CURVE('',#15878,#15875,#10218,.T.);
#20342=EDGE_CURVE('',#15880,#15879,#10219,.T.);
#20343=EDGE_CURVE('',#15881,#15881,#3883,.T.);
#20344=EDGE_CURVE('',#15881,#15882,#10220,.T.);
#20345=EDGE_CURVE('',#15882,#15882,#3884,.T.);
#20346=EDGE_CURVE('',#15883,#15883,#3885,.T.);
#20347=EDGE_CURVE('',#15883,#15884,#10221,.T.);
#20348=EDGE_CURVE('',#15884,#15884,#3886,.T.);
#20349=EDGE_CURVE('',#15885,#15886,#3887,.T.);
#20350=EDGE_CURVE('',#15886,#15885,#3888,.T.);
#20351=EDGE_CURVE('',#15886,#15887,#10222,.T.);
#20352=EDGE_CURVE('',#15887,#15887,#3889,.T.);
#20353=EDGE_CURVE('',#15888,#15889,#3890,.T.);
#20354=EDGE_CURVE('',#15889,#15888,#3891,.T.);
#20355=EDGE_CURVE('',#15888,#15885,#10223,.T.);
#20356=EDGE_CURVE('',#15890,#15889,#10224,.T.);
#20357=EDGE_CURVE('',#15891,#15892,#10225,.T.);
#20358=EDGE_CURVE('',#15891,#15893,#10226,.T.);
#20359=EDGE_CURVE('',#15893,#15894,#10227,.T.);
#20360=EDGE_CURVE('',#15895,#15894,#10228,.T.);
#20361=EDGE_CURVE('',#15896,#15895,#511,.T.);
#20362=EDGE_CURVE('',#15897,#15896,#10229,.T.);
#20363=EDGE_CURVE('',#15898,#15897,#10230,.T.);
#20364=EDGE_CURVE('',#15899,#15898,#10231,.T.);
#20365=EDGE_CURVE('',#15900,#15899,#10232,.T.);
#20366=EDGE_CURVE('',#15901,#15900,#10233,.T.);
#20367=EDGE_CURVE('',#15902,#15901,#10234,.T.);
#20368=EDGE_CURVE('',#15903,#15902,#10235,.T.);
#20369=EDGE_CURVE('',#15904,#15903,#10236,.T.);
#20370=EDGE_CURVE('',#15905,#15904,#10237,.T.);
#20371=EDGE_CURVE('',#15906,#15905,#512,.T.);
#20372=EDGE_CURVE('',#15892,#15906,#10238,.T.);
#20373=EDGE_CURVE('',#15907,#15908,#3892,.T.);
#20374=EDGE_CURVE('',#15908,#15909,#10239,.T.);
#20375=EDGE_CURVE('',#15909,#15910,#3893,.T.);
#20376=EDGE_CURVE('',#15910,#15907,#10240,.T.);
#20377=EDGE_CURVE('',#15910,#15911,#10241,.T.);
#20378=EDGE_CURVE('',#15911,#15912,#10242,.T.);
#20379=EDGE_CURVE('',#15912,#15907,#10243,.T.);
#20380=EDGE_CURVE('',#15913,#15914,#3894,.T.);
#20381=EDGE_CURVE('',#15914,#15915,#10244,.T.);
#20382=EDGE_CURVE('',#15915,#15916,#3895,.T.);
#20383=EDGE_CURVE('',#15916,#15913,#10245,.T.);
#20384=EDGE_CURVE('',#15916,#15917,#10246,.T.);
#20385=EDGE_CURVE('',#15917,#15918,#10247,.T.);
#20386=EDGE_CURVE('',#15918,#15919,#10248,.T.);
#20387=EDGE_CURVE('',#15919,#15920,#10249,.T.);
#20388=EDGE_CURVE('',#15920,#15913,#10250,.T.);
#20389=EDGE_CURVE('',#15908,#15921,#10251,.T.);
#20390=EDGE_CURVE('',#15905,#15921,#10252,.T.);
#20391=EDGE_CURVE('',#15904,#15922,#10253,.T.);
#20392=EDGE_CURVE('',#15922,#15909,#10254,.T.);
#20393=EDGE_CURVE('',#15922,#15923,#10255,.T.);
#20394=EDGE_CURVE('',#15923,#15924,#10256,.T.);
#20395=EDGE_CURVE('',#15897,#15924,#10257,.T.);
#20396=EDGE_CURVE('',#15911,#15896,#3896,.T.);
#20397=EDGE_CURVE('',#15925,#15915,#10258,.T.);
#20398=EDGE_CURVE('',#15926,#15925,#3897,.T.);
#20399=EDGE_CURVE('',#15926,#15927,#10259,.T.);
#20400=EDGE_CURVE('',#15928,#15927,#10260,.T.);
#20401=EDGE_CURVE('',#15929,#15928,#10261,.T.);
#20402=EDGE_CURVE('',#15929,#15917,#10262,.T.);
#20403=EDGE_CURVE('',#15914,#15930,#10263,.T.);
#20404=EDGE_CURVE('',#15925,#15930,#10264,.T.);
#20405=EDGE_CURVE('',#15931,#15912,#3898,.T.);
#20406=EDGE_CURVE('',#15932,#15931,#10265,.T.);
#20407=EDGE_CURVE('',#15933,#15932,#10266,.T.);
#20408=EDGE_CURVE('',#15934,#15933,#10267,.T.);
#20409=EDGE_CURVE('',#15930,#15934,#3899,.T.);
#20410=EDGE_CURVE('',#15935,#15920,#3900,.T.);
#20411=EDGE_CURVE('',#15936,#15935,#10268,.T.);
#20412=EDGE_CURVE('',#15937,#15936,#10269,.T.);
#20413=EDGE_CURVE('',#15938,#15937,#10270,.T.);
#20414=EDGE_CURVE('',#15921,#15938,#3901,.T.);
#20415=EDGE_CURVE('',#15939,#15939,#3902,.T.);
#20416=EDGE_CURVE('',#15940,#15940,#3903,.T.);
#20417=EDGE_CURVE('',#15940,#15941,#10271,.T.);
#20418=EDGE_CURVE('',#15942,#15941,#3904,.T.);
#20419=EDGE_CURVE('',#15941,#15942,#3905,.T.);
#20420=EDGE_CURVE('',#15895,#15931,#458,.T.);
#20421=EDGE_CURVE('',#15932,#15894,#10272,.T.);
#20422=EDGE_CURVE('',#15893,#15943,#10273,.T.);
#20423=EDGE_CURVE('',#15944,#15943,#10274,.T.);
#20424=EDGE_CURVE('',#15945,#15944,#10275,.T.);
#20425=EDGE_CURVE('',#15945,#15946,#10276,.T.);
#20426=EDGE_CURVE('',#15947,#15946,#10277,.T.);
#20427=EDGE_CURVE('',#15933,#15947,#10278,.T.);
#20428=EDGE_CURVE('',#15948,#15948,#3906,.T.);
#20429=EDGE_CURVE('',#15949,#15949,#3907,.T.);
#20430=EDGE_CURVE('',#15950,#15950,#3908,.T.);
#20431=EDGE_CURVE('',#15948,#15951,#10279,.T.);
#20432=EDGE_CURVE('',#15952,#15951,#3909,.T.);
#20433=EDGE_CURVE('',#15951,#15952,#3910,.T.);
#20434=EDGE_CURVE('',#15953,#15947,#10280,.T.);
#20435=EDGE_CURVE('',#15934,#15953,#459,.T.);
#20436=EDGE_CURVE('',#15954,#15945,#10281,.T.);
#20437=EDGE_CURVE('',#15955,#15944,#10282,.T.);
#20438=EDGE_CURVE('',#15956,#15955,#460,.T.);
#20439=EDGE_CURVE('',#15957,#15956,#10283,.T.);
#20440=EDGE_CURVE('',#15958,#15957,#461,.T.);
#20441=EDGE_CURVE('',#15959,#15958,#10284,.T.);
#20442=EDGE_CURVE('',#15960,#15959,#10285,.T.);
#20443=EDGE_CURVE('',#15961,#15960,#10286,.T.);
#20444=EDGE_CURVE('',#15962,#15961,#10287,.T.);
#20445=EDGE_CURVE('',#15954,#15962,#10288,.T.);
#20446=EDGE_CURVE('',#15950,#15963,#10289,.T.);
#20447=EDGE_CURVE('',#15964,#15963,#3911,.T.);
#20448=EDGE_CURVE('',#15963,#15964,#3912,.T.);
#20449=EDGE_CURVE('',#15965,#15954,#10290,.T.);
#20450=EDGE_CURVE('',#15965,#15946,#10291,.T.);
#20451=EDGE_CURVE('',#15966,#15891,#10292,.T.);
#20452=EDGE_CURVE('',#15966,#15943,#10293,.T.);
#20453=EDGE_CURVE('',#15949,#15967,#10294,.T.);
#20454=EDGE_CURVE('',#15968,#15967,#3913,.T.);
#20455=EDGE_CURVE('',#15967,#15968,#3914,.T.);
#20456=EDGE_CURVE('',#15969,#15966,#10295,.T.);
#20457=EDGE_CURVE('',#15970,#15969,#10296,.T.);
#20458=EDGE_CURVE('',#15971,#15970,#10297,.T.);
#20459=EDGE_CURVE('',#15959,#15971,#10298,.T.);
#20460=EDGE_CURVE('',#15957,#15958,#462,.T.);
#20461=EDGE_CURVE('',#15955,#15956,#463,.T.);
#20462=EDGE_CURVE('',#15972,#15965,#10299,.T.);
#20463=EDGE_CURVE('',#15973,#15972,#3915,.T.);
#20464=EDGE_CURVE('',#15974,#15973,#10300,.T.);
#20465=EDGE_CURVE('',#15974,#15975,#10301,.T.);
#20466=EDGE_CURVE('',#15919,#15975,#513,.T.);
#20467=EDGE_CURVE('',#15976,#15918,#10302,.T.);
#20468=EDGE_CURVE('',#15977,#15976,#10303,.T.);
#20469=EDGE_CURVE('',#15978,#15977,#10304,.T.);
#20470=EDGE_CURVE('',#15979,#15978,#10305,.T.);
#20471=EDGE_CURVE('',#15980,#15979,#10306,.T.);
#20472=EDGE_CURVE('',#15981,#15980,#10307,.T.);
#20473=EDGE_CURVE('',#15927,#15981,#10308,.T.);
#20474=EDGE_CURVE('',#15953,#15926,#514,.T.);
#20475=EDGE_CURVE('',#15982,#15983,#3916,.T.);
#20476=EDGE_CURVE('',#15983,#15984,#10309,.T.);
#20477=EDGE_CURVE('',#15985,#15984,#3917,.T.);
#20478=EDGE_CURVE('',#15984,#15985,#3918,.T.);
#20479=EDGE_CURVE('',#15983,#15986,#3919,.T.);
#20480=EDGE_CURVE('',#15987,#15986,#10310,.T.);
#20481=EDGE_CURVE('',#15988,#15987,#464,.T.);
#20482=EDGE_CURVE('',#15989,#15988,#465,.T.);
#20483=EDGE_CURVE('',#15982,#15989,#10311,.T.);
#20484=EDGE_CURVE('',#15990,#15991,#3920,.T.);
#20485=EDGE_CURVE('',#15991,#15992,#10312,.T.);
#20486=EDGE_CURVE('',#15992,#15992,#3921,.T.);
#20487=EDGE_CURVE('',#15991,#15993,#3922,.T.);
#20488=EDGE_CURVE('',#15994,#15993,#10313,.T.);
#20489=EDGE_CURVE('',#15995,#15994,#466,.T.);
#20490=EDGE_CURVE('',#15996,#15995,#467,.T.);
#20491=EDGE_CURVE('',#15990,#15996,#10314,.T.);
#20492=EDGE_CURVE('',#15997,#15994,#10315,.T.);
#20493=EDGE_CURVE('',#15997,#15995,#10316,.T.);
#20494=EDGE_CURVE('',#15996,#15997,#10317,.T.);
#20495=EDGE_CURVE('',#15998,#15999,#10318,.T.);
#20496=EDGE_CURVE('',#15998,#16000,#10319,.T.);
#20497=EDGE_CURVE('',#16000,#16001,#10320,.T.);
#20498=EDGE_CURVE('',#15999,#16001,#10321,.T.);
#20499=EDGE_CURVE('',#16002,#15998,#10322,.T.);
#20500=EDGE_CURVE('',#16002,#16003,#10323,.T.);
#20501=EDGE_CURVE('',#16003,#16000,#10324,.T.);
#20502=EDGE_CURVE('',#16004,#16002,#10325,.T.);
#20503=EDGE_CURVE('',#16004,#16005,#10326,.T.);
#20504=EDGE_CURVE('',#16005,#16003,#10327,.T.);
#20505=EDGE_CURVE('',#15986,#15982,#10328,.T.);
#20506=EDGE_CURVE('',#16006,#15990,#515,.T.);
#20507=EDGE_CURVE('',#16006,#16007,#3923,.T.);
#20508=EDGE_CURVE('',#15993,#16007,#516,.T.);
#20509=EDGE_CURVE('',#16007,#16006,#10329,.T.);
#20510=EDGE_CURVE('',#16008,#16008,#3924,.T.);
#20511=EDGE_CURVE('',#16009,#16010,#3925,.T.);
#20512=EDGE_CURVE('',#16010,#16009,#3926,.T.);
#20513=EDGE_CURVE('',#16009,#16011,#10330,.T.);
#20514=EDGE_CURVE('',#16011,#16011,#3927,.T.);
#20515=EDGE_CURVE('',#16012,#16013,#3928,.T.);
#20516=EDGE_CURVE('',#16013,#16012,#3929,.T.);
#20517=EDGE_CURVE('',#16012,#16014,#10331,.T.);
#20518=EDGE_CURVE('',#16014,#16014,#3930,.T.);
#20519=EDGE_CURVE('',#16015,#16016,#3931,.T.);
#20520=EDGE_CURVE('',#16016,#16015,#3932,.T.);
#20521=EDGE_CURVE('',#16015,#16017,#10332,.T.);
#20522=EDGE_CURVE('',#16017,#16017,#3933,.T.);
#20523=EDGE_CURVE('',#16018,#16019,#3934,.T.);
#20524=EDGE_CURVE('',#16019,#16018,#3935,.T.);
#20525=EDGE_CURVE('',#16018,#16020,#10333,.T.);
#20526=EDGE_CURVE('',#16020,#16020,#3936,.T.);
#20527=EDGE_CURVE('',#15988,#16021,#10334,.T.);
#20528=EDGE_CURVE('',#16022,#16021,#10335,.T.);
#20529=EDGE_CURVE('',#16023,#16022,#10336,.T.);
#20530=EDGE_CURVE('',#15969,#16023,#10337,.T.);
#20531=EDGE_CURVE('',#15989,#15969,#10338,.T.);
#20532=EDGE_CURVE('',#15962,#15987,#10339,.T.);
#20533=EDGE_CURVE('',#16024,#15962,#10340,.T.);
#20534=EDGE_CURVE('',#16025,#16024,#10341,.T.);
#20535=EDGE_CURVE('',#16021,#16025,#10342,.T.);
#20536=EDGE_CURVE('',#15973,#15972,#10343,.T.);
#20537=EDGE_CURVE('',#16026,#15973,#3937,.T.);
#20538=EDGE_CURVE('',#15972,#16026,#3938,.T.);
#20539=EDGE_CURVE('',#15999,#16027,#10344,.T.);
#20540=EDGE_CURVE('',#16027,#16028,#10345,.T.);
#20541=EDGE_CURVE('',#16028,#16004,#10346,.T.);
#20542=EDGE_CURVE('',#16029,#16030,#10347,.T.);
#20543=EDGE_CURVE('',#16030,#16031,#10348,.T.);
#20544=EDGE_CURVE('',#16031,#16032,#3939,.T.);
#20545=EDGE_CURVE('',#16032,#16029,#10349,.T.);
#20546=EDGE_CURVE('',#16033,#16033,#3940,.T.);
#20547=EDGE_CURVE('',#16033,#16034,#10350,.T.);
#20548=EDGE_CURVE('',#16034,#16034,#3941,.T.);
#20549=EDGE_CURVE('',#16035,#16036,#517,.T.);
#20550=EDGE_CURVE('',#16036,#16037,#10351,.T.);
#20551=EDGE_CURVE('',#16037,#16038,#518,.T.);
#20552=EDGE_CURVE('',#16038,#16039,#10352,.T.);
#20553=EDGE_CURVE('',#16040,#16039,#10353,.T.);
#20554=EDGE_CURVE('',#16035,#16040,#10354,.T.);
#20555=EDGE_CURVE('',#16041,#16042,#519,.T.);
#20556=EDGE_CURVE('',#16042,#16043,#10355,.T.);
#20557=EDGE_CURVE('',#16043,#16035,#520,.T.);
#20558=EDGE_CURVE('',#16044,#16040,#10356,.T.);
#20559=EDGE_CURVE('',#16041,#16044,#10357,.T.);
#20560=EDGE_CURVE('',#16045,#16046,#521,.T.);
#20561=EDGE_CURVE('',#16046,#16047,#10358,.T.);
#20562=EDGE_CURVE('',#16047,#16041,#522,.T.);
#20563=EDGE_CURVE('',#16048,#16044,#10359,.T.);
#20564=EDGE_CURVE('',#16045,#16048,#10360,.T.);
#20565=EDGE_CURVE('',#16049,#16050,#523,.T.);
#20566=EDGE_CURVE('',#16050,#16051,#10361,.T.);
#20567=EDGE_CURVE('',#16051,#16045,#524,.T.);
#20568=EDGE_CURVE('',#16052,#16048,#10362,.T.);
#20569=EDGE_CURVE('',#16049,#16052,#10363,.T.);
#20570=EDGE_CURVE('',#16053,#16049,#525,.T.);
#20571=EDGE_CURVE('',#16053,#16050,#3942,.T.);
#20572=EDGE_CURVE('',#16051,#16046,#3943,.T.);
#20573=EDGE_CURVE('',#16054,#16055,#526,.T.);
#20574=EDGE_CURVE('',#16056,#16054,#527,.T.);
#20575=EDGE_CURVE('',#16056,#16055,#3944,.T.);
#20576=EDGE_CURVE('',#16038,#16057,#528,.T.);
#20577=EDGE_CURVE('',#16037,#16057,#3945,.T.);
#20578=EDGE_CURVE('',#16043,#16036,#3946,.T.);
#20579=EDGE_CURVE('',#16057,#16056,#10364,.T.);
#20580=EDGE_CURVE('',#16054,#16058,#10365,.T.);
#20581=EDGE_CURVE('',#16039,#16058,#10366,.T.);
#20582=EDGE_CURVE('',#16055,#16053,#10367,.T.);
#20583=EDGE_CURVE('',#16058,#16052,#10368,.T.);
#20584=EDGE_CURVE('',#16047,#16042,#3947,.T.);
#20585=EDGE_CURVE('',#16059,#16060,#529,.T.);
#20586=EDGE_CURVE('',#16060,#16061,#10369,.T.);
#20587=EDGE_CURVE('',#16061,#16062,#530,.T.);
#20588=EDGE_CURVE('',#16062,#16063,#10370,.T.);
#20589=EDGE_CURVE('',#16064,#16063,#10371,.T.);
#20590=EDGE_CURVE('',#16059,#16064,#10372,.T.);
#20591=EDGE_CURVE('',#16065,#16066,#531,.T.);
#20592=EDGE_CURVE('',#16066,#16067,#10373,.T.);
#20593=EDGE_CURVE('',#16067,#16059,#532,.T.);
#20594=EDGE_CURVE('',#16068,#16064,#10374,.T.);
#20595=EDGE_CURVE('',#16065,#16068,#10375,.T.);
#20596=EDGE_CURVE('',#16069,#16070,#533,.T.);
#20597=EDGE_CURVE('',#16070,#16071,#10376,.T.);
#20598=EDGE_CURVE('',#16071,#16065,#534,.T.);
#20599=EDGE_CURVE('',#16072,#16068,#10377,.T.);
#20600=EDGE_CURVE('',#16069,#16072,#10378,.T.);
#20601=EDGE_CURVE('',#16073,#16074,#535,.T.);
#20602=EDGE_CURVE('',#16074,#16075,#10379,.T.);
#20603=EDGE_CURVE('',#16075,#16069,#536,.T.);
#20604=EDGE_CURVE('',#16076,#16072,#10380,.T.);
#20605=EDGE_CURVE('',#16073,#16076,#10381,.T.);
#20606=EDGE_CURVE('',#16077,#16073,#537,.T.);
#20607=EDGE_CURVE('',#16077,#16074,#3948,.T.);
#20608=EDGE_CURVE('',#16075,#16070,#3949,.T.);
#20609=EDGE_CURVE('',#16078,#16079,#538,.T.);
#20610=EDGE_CURVE('',#16080,#16078,#539,.T.);
#20611=EDGE_CURVE('',#16080,#16079,#3950,.T.);
#20612=EDGE_CURVE('',#16062,#16081,#540,.T.);
#20613=EDGE_CURVE('',#16061,#16081,#3951,.T.);
#20614=EDGE_CURVE('',#16067,#16060,#3952,.T.);
#20615=EDGE_CURVE('',#16081,#16080,#10382,.T.);
#20616=EDGE_CURVE('',#16078,#16082,#10383,.T.);
#20617=EDGE_CURVE('',#16063,#16082,#10384,.T.);
#20618=EDGE_CURVE('',#16079,#16077,#10385,.T.);
#20619=EDGE_CURVE('',#16082,#16076,#10386,.T.);
#20620=EDGE_CURVE('',#16071,#16066,#3953,.T.);
#20621=EDGE_CURVE('',#16083,#15929,#10387,.T.);
#20622=EDGE_CURVE('',#16083,#15976,#10388,.T.);
#20623=EDGE_CURVE('',#15903,#16084,#10389,.T.);
#20624=EDGE_CURVE('',#15902,#16085,#10390,.T.);
#20625=EDGE_CURVE('',#16085,#16084,#10391,.T.);
#20626=EDGE_CURVE('',#15901,#16086,#10392,.T.);
#20627=EDGE_CURVE('',#16086,#16085,#10393,.T.);
#20628=EDGE_CURVE('',#15900,#16087,#10394,.T.);
#20629=EDGE_CURVE('',#16087,#16086,#10395,.T.);
#20630=EDGE_CURVE('',#15899,#16088,#10396,.T.);
#20631=EDGE_CURVE('',#16088,#16087,#10397,.T.);
#20632=EDGE_CURVE('',#15898,#16089,#10398,.T.);
#20633=EDGE_CURVE('',#16089,#16088,#10399,.T.);
#20634=EDGE_CURVE('',#15924,#16089,#10400,.T.);
#20635=EDGE_CURVE('',#15975,#15935,#468,.T.);
#20636=EDGE_CURVE('',#15936,#15974,#10401,.T.);
#20637=EDGE_CURVE('',#15892,#15937,#10402,.T.);
#20638=EDGE_CURVE('',#15938,#15906,#469,.T.);
#20639=EDGE_CURVE('',#15956,#15955,#3954,.T.);
#20640=EDGE_CURVE('',#15958,#15957,#3955,.T.);
#20641=EDGE_CURVE('',#16090,#16091,#10403,.T.);
#20642=EDGE_CURVE('',#16091,#16092,#10404,.T.);
#20643=EDGE_CURVE('',#16092,#16093,#10405,.T.);
#20644=EDGE_CURVE('',#16093,#16094,#10406,.T.);
#20645=EDGE_CURVE('',#16094,#16095,#10407,.T.);
#20646=EDGE_CURVE('',#16095,#16090,#10408,.T.);
#20647=EDGE_CURVE('',#16096,#16097,#10409,.T.);
#20648=EDGE_CURVE('',#16090,#16097,#10410,.T.);
#20649=EDGE_CURVE('',#16095,#16096,#10411,.T.);
#20650=EDGE_CURVE('',#16098,#16096,#10412,.T.);
#20651=EDGE_CURVE('',#16094,#16098,#10413,.T.);
#20652=EDGE_CURVE('',#16093,#16099,#10414,.T.);
#20653=EDGE_CURVE('',#16098,#16099,#10415,.T.);
#20654=EDGE_CURVE('',#16100,#16099,#10416,.T.);
#20655=EDGE_CURVE('',#16092,#16100,#10417,.T.);
#20656=EDGE_CURVE('',#16101,#16100,#10418,.T.);
#20657=EDGE_CURVE('',#16091,#16101,#10419,.T.);
#20658=EDGE_CURVE('',#16097,#16101,#10420,.T.);
#20659=EDGE_CURVE('',#15955,#15956,#3956,.T.);
#20660=EDGE_CURVE('',#16102,#16103,#10421,.T.);
#20661=EDGE_CURVE('',#16103,#16104,#10422,.T.);
#20662=EDGE_CURVE('',#16104,#16105,#10423,.T.);
#20663=EDGE_CURVE('',#16105,#16106,#10424,.T.);
#20664=EDGE_CURVE('',#16106,#16107,#10425,.T.);
#20665=EDGE_CURVE('',#16107,#16102,#10426,.T.);
#20666=EDGE_CURVE('',#16108,#16109,#10427,.T.);
#20667=EDGE_CURVE('',#16102,#16109,#10428,.T.);
#20668=EDGE_CURVE('',#16107,#16108,#10429,.T.);
#20669=EDGE_CURVE('',#16110,#16108,#10430,.T.);
#20670=EDGE_CURVE('',#16106,#16110,#10431,.T.);
#20671=EDGE_CURVE('',#16105,#16111,#10432,.T.);
#20672=EDGE_CURVE('',#16110,#16111,#10433,.T.);
#20673=EDGE_CURVE('',#16112,#16111,#10434,.T.);
#20674=EDGE_CURVE('',#16104,#16112,#10435,.T.);
#20675=EDGE_CURVE('',#16113,#16112,#10436,.T.);
#20676=EDGE_CURVE('',#16103,#16113,#10437,.T.);
#20677=EDGE_CURVE('',#16109,#16113,#10438,.T.);
#20678=EDGE_CURVE('',#15957,#15958,#3957,.T.);
#20679=EDGE_CURVE('',#16028,#16114,#10439,.T.);
#20680=EDGE_CURVE('',#16114,#16005,#10440,.T.);
#20681=EDGE_CURVE('',#16027,#16115,#10441,.T.);
#20682=EDGE_CURVE('',#16114,#16115,#10442,.T.);
#20683=EDGE_CURVE('',#16001,#16115,#10443,.T.);
#20684=EDGE_CURVE('',#16116,#16116,#3958,.T.);
#20685=EDGE_CURVE('',#16026,#16116,#10444,.T.);
#20686=EDGE_CURVE('',#16117,#16118,#10445,.T.);
#20687=EDGE_CURVE('',#16119,#16118,#3959,.T.);
#20688=EDGE_CURVE('',#16118,#16119,#3960,.T.);
#20689=EDGE_CURVE('',#16119,#16120,#10446,.T.);
#20690=EDGE_CURVE('',#16121,#16120,#3961,.T.);
#20691=EDGE_CURVE('',#16120,#16121,#3962,.T.);
#20692=EDGE_CURVE('',#16121,#16122,#10447,.T.);
#20693=EDGE_CURVE('',#16122,#16122,#3963,.T.);
#20694=EDGE_CURVE('',#16123,#16124,#10448,.T.);
#20695=EDGE_CURVE('',#16125,#16124,#3964,.T.);
#20696=EDGE_CURVE('',#16124,#16125,#3965,.T.);
#20697=EDGE_CURVE('',#16125,#16126,#10449,.T.);
#20698=EDGE_CURVE('',#16127,#16126,#3966,.T.);
#20699=EDGE_CURVE('',#16126,#16127,#3967,.T.);
#20700=EDGE_CURVE('',#16127,#16128,#10450,.T.);
#20701=EDGE_CURVE('',#16128,#16128,#3968,.T.);
#20702=EDGE_CURVE('',#16129,#16130,#10451,.T.);
#20703=EDGE_CURVE('',#16131,#16130,#3969,.T.);
#20704=EDGE_CURVE('',#16130,#16131,#3970,.T.);
#20705=EDGE_CURVE('',#16131,#16132,#10452,.T.);
#20706=EDGE_CURVE('',#16133,#16132,#3971,.T.);
#20707=EDGE_CURVE('',#16132,#16133,#3972,.T.);
#20708=EDGE_CURVE('',#16133,#16134,#10453,.T.);
#20709=EDGE_CURVE('',#16134,#16134,#3973,.T.);
#20710=EDGE_CURVE('',#16135,#16136,#3974,.T.);
#20711=EDGE_CURVE('',#16136,#16135,#3975,.T.);
#20712=EDGE_CURVE('',#16136,#16137,#10454,.T.);
#20713=EDGE_CURVE('',#16137,#16137,#3976,.T.);
#20714=EDGE_CURVE('',#16135,#16138,#10455,.T.);
#20715=EDGE_CURVE('',#16139,#16138,#3977,.T.);
#20716=EDGE_CURVE('',#16138,#16139,#3978,.T.);
#20717=EDGE_CURVE('',#16140,#16139,#10456,.T.);
#20718=EDGE_CURVE('',#16141,#16142,#3979,.T.);
#20719=EDGE_CURVE('',#16142,#16141,#3980,.T.);
#20720=EDGE_CURVE('',#16142,#16143,#10457,.T.);
#20721=EDGE_CURVE('',#16143,#16143,#3981,.T.);
#20722=EDGE_CURVE('',#16141,#16144,#10458,.T.);
#20723=EDGE_CURVE('',#16145,#16144,#3982,.T.);
#20724=EDGE_CURVE('',#16144,#16145,#3983,.T.);
#20725=EDGE_CURVE('',#16146,#16145,#10459,.T.);
#20726=EDGE_CURVE('',#16147,#16148,#3984,.T.);
#20727=EDGE_CURVE('',#16148,#16147,#3985,.T.);
#20728=EDGE_CURVE('',#16148,#16149,#10460,.T.);
#20729=EDGE_CURVE('',#16149,#16149,#3986,.T.);
#20730=EDGE_CURVE('',#16147,#16150,#10461,.T.);
#20731=EDGE_CURVE('',#16151,#16150,#3987,.T.);
#20732=EDGE_CURVE('',#16150,#16151,#3988,.T.);
#20733=EDGE_CURVE('',#16152,#16151,#10462,.T.);
#20734=EDGE_CURVE('',#16153,#16154,#3989,.T.);
#20735=EDGE_CURVE('',#16154,#16153,#3990,.T.);
#20736=EDGE_CURVE('',#16154,#16155,#10463,.T.);
#20737=EDGE_CURVE('',#16155,#16155,#3991,.T.);
#20738=EDGE_CURVE('',#16153,#16156,#10464,.T.);
#20739=EDGE_CURVE('',#16157,#16156,#3992,.T.);
#20740=EDGE_CURVE('',#16156,#16157,#3993,.T.);
#20741=EDGE_CURVE('',#16158,#16157,#10465,.T.);
#20742=EDGE_CURVE('',#16159,#15968,#10466,.T.);
#20743=EDGE_CURVE('',#16160,#15942,#10467,.T.);
#20744=EDGE_CURVE('',#16161,#16010,#10468,.T.);
#20745=EDGE_CURVE('',#16162,#16013,#10469,.T.);
#20746=EDGE_CURVE('',#16163,#16016,#10470,.T.);
#20747=EDGE_CURVE('',#16164,#16019,#10471,.T.);
#20748=EDGE_CURVE('',#16165,#15952,#10472,.T.);
#20749=EDGE_CURVE('',#16166,#15964,#10473,.T.);
#20750=EDGE_CURVE('',#16167,#15961,#10474,.T.);
#20751=EDGE_CURVE('',#16168,#15960,#10475,.T.);
#20752=EDGE_CURVE('',#16167,#16168,#10476,.T.);
#20753=EDGE_CURVE('',#16169,#15959,#10477,.T.);
#20754=EDGE_CURVE('',#16168,#16169,#10478,.T.);
#20755=EDGE_CURVE('',#16170,#16021,#10479,.T.);
#20756=EDGE_CURVE('',#16171,#16025,#10480,.T.);
#20757=EDGE_CURVE('',#16170,#16171,#10481,.T.);
#20758=EDGE_CURVE('',#16172,#15971,#10482,.T.);
#20759=EDGE_CURVE('',#16169,#16172,#10483,.T.);
#20760=EDGE_CURVE('',#16173,#15970,#10484,.T.);
#20761=EDGE_CURVE('',#16172,#16173,#10485,.T.);
#20762=EDGE_CURVE('',#16174,#16023,#10486,.T.);
#20763=EDGE_CURVE('',#16173,#16174,#10487,.T.);
#20764=EDGE_CURVE('',#16175,#16022,#10488,.T.);
#20765=EDGE_CURVE('',#16174,#16175,#10489,.T.);
#20766=EDGE_CURVE('',#16175,#16170,#10490,.T.);
#20767=EDGE_CURVE('',#16171,#16176,#10491,.T.);
#20768=EDGE_CURVE('',#16176,#16167,#10492,.T.);
#20769=EDGE_CURVE('',#16177,#16178,#10493,.T.);
#20770=EDGE_CURVE('',#16178,#16179,#10494,.T.);
#20771=EDGE_CURVE('',#16179,#16180,#10495,.T.);
#20772=EDGE_CURVE('',#16180,#16181,#10496,.T.);
#20773=EDGE_CURVE('',#16181,#16182,#10497,.T.);
#20774=EDGE_CURVE('',#16182,#16183,#10498,.T.);
#20775=EDGE_CURVE('',#16183,#16184,#10499,.T.);
#20776=EDGE_CURVE('',#16184,#16177,#10500,.T.);
#20777=EDGE_CURVE('',#16185,#16185,#3994,.T.);
#20778=EDGE_CURVE('',#16186,#16186,#3995,.T.);
#20779=EDGE_CURVE('',#16186,#16187,#10501,.T.);
#20780=EDGE_CURVE('',#16187,#16187,#3996,.T.);
#20781=EDGE_CURVE('',#16188,#16189,#3997,.T.);
#20782=EDGE_CURVE('',#16189,#16190,#10502,.T.);
#20783=EDGE_CURVE('',#16190,#16190,#3998,.T.);
#20784=EDGE_CURVE('',#16189,#16188,#3999,.T.);
#20785=EDGE_CURVE('',#16084,#15923,#10503,.T.);
#20786=EDGE_CURVE('',#16191,#15981,#10504,.T.);
#20787=EDGE_CURVE('',#15928,#16191,#10505,.T.);
#20788=EDGE_CURVE('',#16192,#15980,#10506,.T.);
#20789=EDGE_CURVE('',#16191,#16192,#10507,.T.);
#20790=EDGE_CURVE('',#16193,#15979,#10508,.T.);
#20791=EDGE_CURVE('',#16192,#16193,#10509,.T.);
#20792=EDGE_CURVE('',#16194,#15978,#10510,.T.);
#20793=EDGE_CURVE('',#16193,#16194,#10511,.T.);
#20794=EDGE_CURVE('',#16195,#15977,#10512,.T.);
#20795=EDGE_CURVE('',#16194,#16195,#10513,.T.);
#20796=EDGE_CURVE('',#16195,#16083,#10514,.T.);
#20797=EDGE_CURVE('',#16176,#16024,#10515,.T.);
#20798=EDGE_CURVE('',#16196,#16197,#4000,.T.);
#20799=EDGE_CURVE('',#16197,#16196,#4001,.T.);
#20800=EDGE_CURVE('',#16197,#16198,#10516,.T.);
#20801=EDGE_CURVE('',#16198,#16198,#4002,.T.);
#20802=EDGE_CURVE('',#15939,#16199,#10517,.T.);
#20803=EDGE_CURVE('',#16200,#16199,#831,.T.);
#20804=EDGE_CURVE('',#16201,#16200,#832,.T.);
#20805=EDGE_CURVE('',#16199,#16201,#833,.T.);
#20806=EDGE_CURVE('',#15985,#16202,#10518,.T.);
#20807=EDGE_CURVE('',#16202,#16202,#4003,.T.);
#20808=EDGE_CURVE('',#16196,#16201,#10519,.T.);
#20809=EDGE_CURVE('',#16200,#16185,#10520,.T.);
#20810=EDGE_CURVE('',#16203,#16203,#4004,.T.);
#20811=EDGE_CURVE('',#16203,#16204,#10521,.T.);
#20812=EDGE_CURVE('',#16204,#16204,#4005,.T.);
#20813=EDGE_CURVE('',#16205,#16206,#4006,.T.);
#20814=EDGE_CURVE('',#16206,#16205,#4007,.T.);
#20815=EDGE_CURVE('',#16205,#16207,#10522,.T.);
#20816=EDGE_CURVE('',#16207,#16207,#4008,.T.);
#20817=EDGE_CURVE('',#16208,#16209,#10523,.T.);
#20818=EDGE_CURVE('',#16209,#16210,#10524,.T.);
#20819=EDGE_CURVE('',#16210,#16211,#10525,.T.);
#20820=EDGE_CURVE('',#16211,#16212,#10526,.T.);
#20821=EDGE_CURVE('',#16212,#16213,#10527,.T.);
#20822=EDGE_CURVE('',#16213,#16208,#10528,.T.);
#20823=EDGE_CURVE('',#16214,#16215,#10529,.T.);
#20824=EDGE_CURVE('',#16215,#16216,#10530,.T.);
#20825=EDGE_CURVE('',#16216,#16217,#10531,.T.);
#20826=EDGE_CURVE('',#16217,#16218,#10532,.T.);
#20827=EDGE_CURVE('',#16218,#16219,#10533,.T.);
#20828=EDGE_CURVE('',#16219,#16214,#10534,.T.);
#20829=EDGE_CURVE('',#16220,#16220,#4009,.T.);
#20830=EDGE_CURVE('',#16221,#16221,#4010,.T.);
#20831=EDGE_CURVE('',#16221,#16220,#10535,.T.);
#20832=EDGE_CURVE('',#16222,#16223,#4011,.T.);
#20833=EDGE_CURVE('',#16223,#16222,#4012,.T.);
#20834=EDGE_CURVE('',#16222,#16224,#10536,.T.);
#20835=EDGE_CURVE('',#16224,#16224,#4013,.T.);
#20836=EDGE_CURVE('',#16225,#16226,#4014,.T.);
#20837=EDGE_CURVE('',#16226,#16225,#4015,.T.);
#20838=EDGE_CURVE('',#16225,#16227,#10537,.T.);
#20839=EDGE_CURVE('',#16227,#16227,#4016,.T.);
#20840=EDGE_CURVE('',#16228,#16229,#10538,.T.);
#20841=EDGE_CURVE('',#16228,#16230,#10539,.T.);
#20842=EDGE_CURVE('',#16231,#16230,#4017,.T.);
#20843=EDGE_CURVE('',#16229,#16231,#10540,.T.);
#20844=EDGE_CURVE('',#16232,#16233,#4018,.T.);
#20845=EDGE_CURVE('',#16232,#16231,#834,.T.);
#20846=EDGE_CURVE('',#16230,#16233,#835,.T.);
#20847=EDGE_CURVE('',#16234,#16234,#4019,.T.);
#20848=EDGE_CURVE('',#16233,#16235,#10541,.T.);
#20849=EDGE_CURVE('',#16236,#16235,#4020,.T.);
#20850=EDGE_CURVE('',#16236,#16232,#10542,.T.);
#20851=EDGE_CURVE('',#16237,#16237,#836,.T.);
#20852=EDGE_CURVE('',#16238,#16238,#837,.T.);
#20853=EDGE_CURVE('',#16239,#16240,#4021,.T.);
#20854=EDGE_CURVE('',#16240,#16239,#4022,.T.);
#20855=EDGE_CURVE('',#16239,#16241,#10543,.T.);
#20856=EDGE_CURVE('',#16241,#16241,#4023,.T.);
#20857=EDGE_CURVE('',#16228,#16029,#10544,.T.);
#20858=EDGE_CURVE('',#16229,#16030,#10545,.T.);
#20859=EDGE_CURVE('',#16242,#16243,#10546,.T.);
#20860=EDGE_CURVE('',#16243,#16244,#10547,.T.);
#20861=EDGE_CURVE('',#16244,#16245,#10548,.T.);
#20862=EDGE_CURVE('',#16245,#16246,#10549,.T.);
#20863=EDGE_CURVE('',#16246,#16247,#10550,.T.);
#20864=EDGE_CURVE('',#16247,#16242,#10551,.T.);
#20865=EDGE_CURVE('',#16248,#16249,#10552,.T.);
#20866=EDGE_CURVE('',#16242,#16249,#10553,.T.);
#20867=EDGE_CURVE('',#16247,#16248,#10554,.T.);
#20868=EDGE_CURVE('',#16250,#16248,#10555,.T.);
#20869=EDGE_CURVE('',#16246,#16250,#10556,.T.);
#20870=EDGE_CURVE('',#16245,#16251,#10557,.T.);
#20871=EDGE_CURVE('',#16250,#16251,#10558,.T.);
#20872=EDGE_CURVE('',#16252,#16251,#10559,.T.);
#20873=EDGE_CURVE('',#16244,#16252,#10560,.T.);
#20874=EDGE_CURVE('',#16253,#16252,#10561,.T.);
#20875=EDGE_CURVE('',#16243,#16253,#10562,.T.);
#20876=EDGE_CURVE('',#16249,#16253,#10563,.T.);
#20877=EDGE_CURVE('',#16254,#16255,#10564,.T.);
#20878=EDGE_CURVE('',#16255,#16256,#10565,.T.);
#20879=EDGE_CURVE('',#16256,#16257,#10566,.T.);
#20880=EDGE_CURVE('',#16257,#16258,#10567,.T.);
#20881=EDGE_CURVE('',#16258,#16259,#10568,.T.);
#20882=EDGE_CURVE('',#16259,#16254,#10569,.T.);
#20883=EDGE_CURVE('',#16260,#16261,#10570,.T.);
#20884=EDGE_CURVE('',#16254,#16261,#10571,.T.);
#20885=EDGE_CURVE('',#16259,#16260,#10572,.T.);
#20886=EDGE_CURVE('',#16262,#16260,#10573,.T.);
#20887=EDGE_CURVE('',#16258,#16262,#10574,.T.);
#20888=EDGE_CURVE('',#16257,#16263,#10575,.T.);
#20889=EDGE_CURVE('',#16262,#16263,#10576,.T.);
#20890=EDGE_CURVE('',#16264,#16263,#10577,.T.);
#20891=EDGE_CURVE('',#16256,#16264,#10578,.T.);
#20892=EDGE_CURVE('',#16265,#16264,#10579,.T.);
#20893=EDGE_CURVE('',#16255,#16265,#10580,.T.);
#20894=EDGE_CURVE('',#16261,#16265,#10581,.T.);
#20895=EDGE_CURVE('',#16266,#16266,#4024,.T.);
#20896=EDGE_CURVE('',#16267,#16268,#4025,.T.);
#20897=EDGE_CURVE('',#16268,#16267,#4026,.T.);
#20898=EDGE_CURVE('',#16267,#16266,#10582,.T.);
#20899=EDGE_CURVE('',#16269,#16269,#838,.T.);
#20900=EDGE_CURVE('',#16269,#16268,#10583,.T.);
#20901=EDGE_CURVE('',#16270,#16271,#4027,.T.);
#20902=EDGE_CURVE('',#16271,#16270,#4028,.T.);
#20903=EDGE_CURVE('',#16271,#16272,#10584,.T.);
#20904=EDGE_CURVE('',#16272,#16272,#4029,.T.);
#20905=EDGE_CURVE('',#16273,#16273,#4030,.T.);
#20906=EDGE_CURVE('',#16274,#16275,#4031,.T.);
#20907=EDGE_CURVE('',#16275,#16274,#4032,.T.);
#20908=EDGE_CURVE('',#16274,#16273,#10585,.T.);
#20909=EDGE_CURVE('',#16276,#16277,#10586,.T.);
#20910=EDGE_CURVE('',#16277,#16278,#10587,.T.);
#20911=EDGE_CURVE('',#16278,#16279,#10588,.T.);
#20912=EDGE_CURVE('',#16279,#16280,#10589,.T.);
#20913=EDGE_CURVE('',#16280,#16281,#10590,.T.);
#20914=EDGE_CURVE('',#16281,#16276,#10591,.T.);
#20915=EDGE_CURVE('',#16282,#16283,#10592,.T.);
#20916=EDGE_CURVE('',#16276,#16283,#10593,.T.);
#20917=EDGE_CURVE('',#16281,#16282,#10594,.T.);
#20918=EDGE_CURVE('',#16284,#16282,#10595,.T.);
#20919=EDGE_CURVE('',#16280,#16284,#10596,.T.);
#20920=EDGE_CURVE('',#16279,#16285,#10597,.T.);
#20921=EDGE_CURVE('',#16284,#16285,#10598,.T.);
#20922=EDGE_CURVE('',#16286,#16285,#10599,.T.);
#20923=EDGE_CURVE('',#16278,#16286,#10600,.T.);
#20924=EDGE_CURVE('',#16287,#16286,#10601,.T.);
#20925=EDGE_CURVE('',#16277,#16287,#10602,.T.);
#20926=EDGE_CURVE('',#16283,#16287,#10603,.T.);
#20927=EDGE_CURVE('',#16288,#16289,#10604,.T.);
#20928=EDGE_CURVE('',#16289,#16290,#10605,.T.);
#20929=EDGE_CURVE('',#16290,#16291,#10606,.T.);
#20930=EDGE_CURVE('',#16291,#16292,#10607,.T.);
#20931=EDGE_CURVE('',#16292,#16293,#10608,.T.);
#20932=EDGE_CURVE('',#16293,#16288,#10609,.T.);
#20933=EDGE_CURVE('',#16294,#16295,#10610,.T.);
#20934=EDGE_CURVE('',#16288,#16295,#10611,.T.);
#20935=EDGE_CURVE('',#16293,#16294,#10612,.T.);
#20936=EDGE_CURVE('',#16296,#16294,#10613,.T.);
#20937=EDGE_CURVE('',#16292,#16296,#10614,.T.);
#20938=EDGE_CURVE('',#16291,#16297,#10615,.T.);
#20939=EDGE_CURVE('',#16296,#16297,#10616,.T.);
#20940=EDGE_CURVE('',#16298,#16297,#10617,.T.);
#20941=EDGE_CURVE('',#16290,#16298,#10618,.T.);
#20942=EDGE_CURVE('',#16299,#16298,#10619,.T.);
#20943=EDGE_CURVE('',#16289,#16299,#10620,.T.);
#20944=EDGE_CURVE('',#16295,#16299,#10621,.T.);
#20945=EDGE_CURVE('',#16300,#16300,#4033,.T.);
#20946=EDGE_CURVE('',#16301,#16302,#4034,.T.);
#20947=EDGE_CURVE('',#16302,#16301,#4035,.T.);
#20948=EDGE_CURVE('',#16301,#16300,#10622,.T.);
#20949=EDGE_CURVE('',#16303,#16303,#839,.T.);
#20950=EDGE_CURVE('',#16303,#16302,#10623,.T.);
#20951=EDGE_CURVE('',#16304,#16305,#4036,.T.);
#20952=EDGE_CURVE('',#16305,#16304,#4037,.T.);
#20953=EDGE_CURVE('',#16305,#16306,#10624,.T.);
#20954=EDGE_CURVE('',#16306,#16306,#4038,.T.);
#20955=EDGE_CURVE('',#16307,#16307,#4039,.T.);
#20956=EDGE_CURVE('',#16308,#16309,#4040,.T.);
#20957=EDGE_CURVE('',#16309,#16308,#4041,.T.);
#20958=EDGE_CURVE('',#16308,#16307,#10625,.T.);
#20959=EDGE_CURVE('',#16310,#16310,#840,.T.);
#20960=EDGE_CURVE('',#16310,#16309,#10626,.T.);
#20961=EDGE_CURVE('',#16240,#16311,#10627,.T.);
#20962=EDGE_CURVE('',#16311,#16311,#4042,.T.);
#20963=EDGE_CURVE('',#16304,#16237,#10628,.T.);
#20964=EDGE_CURVE('',#16270,#16238,#10629,.T.);
#20965=EDGE_CURVE('',#16312,#16312,#4043,.T.);
#20966=EDGE_CURVE('',#16223,#16312,#10630,.T.);
#20967=EDGE_CURVE('',#16313,#16313,#841,.T.);
#20968=EDGE_CURVE('',#16313,#16275,#10631,.T.);
#20969=EDGE_CURVE('',#16314,#16315,#4044,.T.);
#20970=EDGE_CURVE('',#16315,#16314,#4045,.T.);
#20971=EDGE_CURVE('',#16314,#16316,#10632,.T.);
#20972=EDGE_CURVE('',#16316,#16316,#4046,.T.);
#20973=EDGE_CURVE('',#16315,#16234,#10633,.T.);
#20974=EDGE_CURVE('',#16235,#16032,#842,.T.);
#20975=EDGE_CURVE('',#16031,#16236,#843,.T.);
#20976=EDGE_CURVE('',#16317,#16317,#4047,.T.);
#20977=EDGE_CURVE('',#16317,#16226,#10634,.T.);
#20978=EDGE_CURVE('',#16318,#16318,#4048,.T.);
#20979=EDGE_CURVE('',#16319,#16319,#4049,.T.);
#20980=EDGE_CURVE('',#16188,#16319,#10635,.T.);
#20981=EDGE_CURVE('',#16318,#16320,#10636,.T.);
#20982=EDGE_CURVE('',#16320,#16320,#4050,.T.);
#20983=EDGE_CURVE('',#16321,#16321,#4051,.T.);
#20984=EDGE_CURVE('',#16206,#16321,#10637,.T.);
#20985=EDGE_CURVE('',#16322,#16323,#4052,.T.);
#20986=EDGE_CURVE('',#16324,#16322,#10638,.T.);
#20987=EDGE_CURVE('',#16325,#16324,#4053,.T.);
#20988=EDGE_CURVE('',#16326,#16325,#10639,.T.);
#20989=EDGE_CURVE('',#16327,#16326,#4054,.T.);
#20990=EDGE_CURVE('',#16328,#16327,#10640,.T.);
#20991=EDGE_CURVE('',#16329,#16328,#4055,.T.);
#20992=EDGE_CURVE('',#16330,#16329,#10641,.T.);
#20993=EDGE_CURVE('',#16331,#16330,#4056,.T.);
#20994=EDGE_CURVE('',#16332,#16331,#10642,.T.);
#20995=EDGE_CURVE('',#16333,#16332,#4057,.T.);
#20996=EDGE_CURVE('',#16323,#16333,#10643,.T.);
#20997=EDGE_CURVE('',#16334,#16332,#541,.T.);
#20998=EDGE_CURVE('',#16333,#16334,#542,.T.);
#20999=EDGE_CURVE('',#16335,#16326,#543,.T.);
#21000=EDGE_CURVE('',#16325,#16336,#544,.T.);
#21001=EDGE_CURVE('',#16336,#16217,#10644,.T.);
#21002=EDGE_CURVE('',#16335,#16216,#10645,.T.);
#21003=EDGE_CURVE('',#16337,#16328,#545,.T.);
#21004=EDGE_CURVE('',#16327,#16335,#546,.T.);
#21005=EDGE_CURVE('',#16337,#16215,#10646,.T.);
#21006=EDGE_CURVE('',#16331,#16338,#547,.T.);
#21007=EDGE_CURVE('',#16338,#16330,#548,.T.);
#21008=EDGE_CURVE('',#16329,#16337,#549,.T.);
#21009=EDGE_CURVE('',#16322,#16339,#550,.T.);
#21010=EDGE_CURVE('',#16339,#16323,#551,.T.);
#21011=EDGE_CURVE('',#16336,#16324,#552,.T.);
#21012=EDGE_CURVE('',#16339,#16218,#10647,.T.);
#21013=EDGE_CURVE('',#16334,#16219,#10648,.T.);
#21014=EDGE_CURVE('',#16338,#16214,#10649,.T.);
#21015=EDGE_CURVE('',#16340,#16341,#4058,.T.);
#21016=EDGE_CURVE('',#16342,#16340,#10650,.T.);
#21017=EDGE_CURVE('',#16343,#16342,#4059,.T.);
#21018=EDGE_CURVE('',#16344,#16343,#10651,.T.);
#21019=EDGE_CURVE('',#16345,#16344,#4060,.T.);
#21020=EDGE_CURVE('',#16346,#16345,#10652,.T.);
#21021=EDGE_CURVE('',#16347,#16346,#4061,.T.);
#21022=EDGE_CURVE('',#16348,#16347,#10653,.T.);
#21023=EDGE_CURVE('',#16349,#16348,#4062,.T.);
#21024=EDGE_CURVE('',#16350,#16349,#10654,.T.);
#21025=EDGE_CURVE('',#16351,#16350,#4063,.T.);
#21026=EDGE_CURVE('',#16341,#16351,#10655,.T.);
#21027=EDGE_CURVE('',#16352,#16350,#553,.T.);
#21028=EDGE_CURVE('',#16351,#16352,#554,.T.);
#21029=EDGE_CURVE('',#16353,#16344,#555,.T.);
#21030=EDGE_CURVE('',#16343,#16354,#556,.T.);
#21031=EDGE_CURVE('',#16354,#16211,#10656,.T.);
#21032=EDGE_CURVE('',#16353,#16210,#10657,.T.);
#21033=EDGE_CURVE('',#16355,#16346,#557,.T.);
#21034=EDGE_CURVE('',#16345,#16353,#558,.T.);
#21035=EDGE_CURVE('',#16355,#16209,#10658,.T.);
#21036=EDGE_CURVE('',#16349,#16356,#559,.T.);
#21037=EDGE_CURVE('',#16356,#16348,#560,.T.);
#21038=EDGE_CURVE('',#16347,#16355,#561,.T.);
#21039=EDGE_CURVE('',#16340,#16357,#562,.T.);
#21040=EDGE_CURVE('',#16357,#16341,#563,.T.);
#21041=EDGE_CURVE('',#16354,#16342,#564,.T.);
#21042=EDGE_CURVE('',#16357,#16212,#10659,.T.);
#21043=EDGE_CURVE('',#16352,#16213,#10660,.T.);
#21044=EDGE_CURVE('',#16356,#16208,#10661,.T.);
#21045=EDGE_CURVE('',#16358,#16358,#4064,.T.);
#21046=EDGE_CURVE('',#16359,#16359,#4065,.T.);
#21047=EDGE_CURVE('',#16360,#16360,#4066,.T.);
#21048=EDGE_CURVE('',#16361,#16361,#4067,.T.);
#21049=EDGE_CURVE('',#16361,#16362,#10662,.T.);
#21050=EDGE_CURVE('',#16362,#16362,#4068,.T.);
#21051=EDGE_CURVE('',#16363,#16363,#4069,.T.);
#21052=EDGE_CURVE('',#16363,#16364,#10663,.T.);
#21053=EDGE_CURVE('',#16364,#16364,#4070,.T.);
#21054=EDGE_CURVE('',#16365,#16365,#4071,.T.);
#21055=EDGE_CURVE('',#16365,#16008,#10664,.T.);
#21056=EDGE_CURVE('',#16366,#16366,#4072,.T.);
#21057=EDGE_CURVE('',#16366,#16367,#10665,.T.);
#21058=EDGE_CURVE('',#16367,#16367,#4073,.T.);
#21059=EDGE_CURVE('',#16368,#16368,#4074,.T.);
#21060=EDGE_CURVE('',#16368,#16369,#10666,.T.);
#21061=EDGE_CURVE('',#16369,#16369,#4075,.T.);
#21062=EDGE_CURVE('',#16370,#16370,#4076,.T.);
#21063=EDGE_CURVE('',#16370,#16371,#10667,.T.);
#21064=EDGE_CURVE('',#16371,#16371,#4077,.T.);
#21065=EDGE_CURVE('',#16372,#16372,#4078,.T.);
#21066=EDGE_CURVE('',#16372,#16373,#10668,.T.);
#21067=EDGE_CURVE('',#16373,#16373,#4079,.T.);
#21068=EDGE_CURVE('',#16374,#16375,#4080,.T.);
#21069=EDGE_CURVE('',#16374,#16376,#4081,.T.);
#21070=EDGE_CURVE('',#16376,#16377,#10669,.T.);
#21071=EDGE_CURVE('',#16377,#16378,#4082,.T.);
#21072=EDGE_CURVE('',#16378,#16379,#4083,.T.);
#21073=EDGE_CURVE('',#16379,#16380,#4084,.T.);
#21074=EDGE_CURVE('',#16380,#16381,#10670,.T.);
#21075=EDGE_CURVE('',#16381,#16375,#4085,.T.);
#21076=EDGE_CURVE('',#16382,#16383,#10671,.T.);
#21077=EDGE_CURVE('',#16384,#16383,#10672,.T.);
#21078=EDGE_CURVE('',#16385,#16384,#10673,.T.);
#21079=EDGE_CURVE('',#16385,#16382,#10674,.T.);
#21080=EDGE_CURVE('',#16383,#16386,#4086,.T.);
#21081=EDGE_CURVE('',#16387,#16386,#10675,.T.);
#21082=EDGE_CURVE('',#16384,#16387,#4087,.T.);
#21083=EDGE_CURVE('',#16386,#16388,#4088,.T.);
#21084=EDGE_CURVE('',#16389,#16388,#10676,.T.);
#21085=EDGE_CURVE('',#16387,#16389,#4089,.T.);
#21086=EDGE_CURVE('',#16388,#16390,#4090,.T.);
#21087=EDGE_CURVE('',#16391,#16390,#10677,.T.);
#21088=EDGE_CURVE('',#16389,#16391,#4091,.T.);
#21089=EDGE_CURVE('',#16390,#16392,#10678,.T.);
#21090=EDGE_CURVE('',#16393,#16392,#10679,.T.);
#21091=EDGE_CURVE('',#16391,#16393,#10680,.T.);
#21092=EDGE_CURVE('',#16392,#16394,#4092,.T.);
#21093=EDGE_CURVE('',#16395,#16394,#10681,.T.);
#21094=EDGE_CURVE('',#16393,#16395,#4093,.T.);
#21095=EDGE_CURVE('',#16396,#16394,#4094,.T.);
#21096=EDGE_CURVE('',#16397,#16396,#10682,.T.);
#21097=EDGE_CURVE('',#16397,#16395,#4095,.T.);
#21098=EDGE_CURVE('',#16396,#16382,#4096,.T.);
#21099=EDGE_CURVE('',#16397,#16385,#4097,.T.);
#21100=EDGE_CURVE('',#16398,#16399,#10683,.T.);
#21101=EDGE_CURVE('',#16400,#16399,#10684,.T.);
#21102=EDGE_CURVE('',#16401,#16400,#10685,.T.);
#21103=EDGE_CURVE('',#16401,#16398,#10686,.T.);
#21104=EDGE_CURVE('',#16399,#16402,#4098,.T.);
#21105=EDGE_CURVE('',#16403,#16402,#10687,.T.);
#21106=EDGE_CURVE('',#16400,#16403,#4099,.T.);
#21107=EDGE_CURVE('',#16402,#16404,#4100,.T.);
#21108=EDGE_CURVE('',#16405,#16404,#10688,.T.);
#21109=EDGE_CURVE('',#16403,#16405,#4101,.T.);
#21110=EDGE_CURVE('',#16404,#16406,#4102,.T.);
#21111=EDGE_CURVE('',#16407,#16406,#10689,.T.);
#21112=EDGE_CURVE('',#16405,#16407,#4103,.T.);
#21113=EDGE_CURVE('',#16406,#16408,#10690,.T.);
#21114=EDGE_CURVE('',#16409,#16408,#10691,.T.);
#21115=EDGE_CURVE('',#16407,#16409,#10692,.T.);
#21116=EDGE_CURVE('',#16408,#16410,#4104,.T.);
#21117=EDGE_CURVE('',#16411,#16410,#10693,.T.);
#21118=EDGE_CURVE('',#16409,#16411,#4105,.T.);
#21119=EDGE_CURVE('',#16412,#16410,#4106,.T.);
#21120=EDGE_CURVE('',#16413,#16412,#10694,.T.);
#21121=EDGE_CURVE('',#16413,#16411,#4107,.T.);
#21122=EDGE_CURVE('',#16412,#16398,#4108,.T.);
#21123=EDGE_CURVE('',#16413,#16401,#4109,.T.);
#21124=EDGE_CURVE('',#16414,#16415,#10695,.T.);
#21125=EDGE_CURVE('',#16416,#16415,#10696,.T.);
#21126=EDGE_CURVE('',#16417,#16416,#10697,.T.);
#21127=EDGE_CURVE('',#16417,#16414,#10698,.T.);
#21128=EDGE_CURVE('',#16415,#16418,#4110,.T.);
#21129=EDGE_CURVE('',#16419,#16418,#10699,.T.);
#21130=EDGE_CURVE('',#16416,#16419,#4111,.T.);
#21131=EDGE_CURVE('',#16418,#16420,#4112,.T.);
#21132=EDGE_CURVE('',#16421,#16420,#10700,.T.);
#21133=EDGE_CURVE('',#16419,#16421,#4113,.T.);
#21134=EDGE_CURVE('',#16420,#16422,#4114,.T.);
#21135=EDGE_CURVE('',#16423,#16422,#10701,.T.);
#21136=EDGE_CURVE('',#16421,#16423,#4115,.T.);
#21137=EDGE_CURVE('',#16422,#16424,#10702,.T.);
#21138=EDGE_CURVE('',#16425,#16424,#10703,.T.);
#21139=EDGE_CURVE('',#16423,#16425,#10704,.T.);
#21140=EDGE_CURVE('',#16424,#16426,#4116,.T.);
#21141=EDGE_CURVE('',#16427,#16426,#10705,.T.);
#21142=EDGE_CURVE('',#16425,#16427,#4117,.T.);
#21143=EDGE_CURVE('',#16428,#16426,#4118,.T.);
#21144=EDGE_CURVE('',#16429,#16428,#10706,.T.);
#21145=EDGE_CURVE('',#16429,#16427,#4119,.T.);
#21146=EDGE_CURVE('',#16428,#16414,#4120,.T.);
#21147=EDGE_CURVE('',#16429,#16417,#4121,.T.);
#21148=EDGE_CURVE('',#16360,#16430,#10707,.T.);
#21149=EDGE_CURVE('',#16430,#16430,#4122,.T.);
#21150=EDGE_CURVE('',#16359,#16431,#10708,.T.);
#21151=EDGE_CURVE('',#16431,#16431,#4123,.T.);
#21152=EDGE_CURVE('',#16358,#16432,#10709,.T.);
#21153=EDGE_CURVE('',#16432,#16432,#4124,.T.);
#21154=EDGE_CURVE('',#16433,#16434,#4125,.T.);
#21155=EDGE_CURVE('',#16435,#16434,#470,.T.);
#21156=EDGE_CURVE('',#16436,#16435,#4126,.T.);
#21157=EDGE_CURVE('',#16433,#16436,#471,.T.);
#21158=EDGE_CURVE('',#16435,#16436,#10710,.T.);
#21159=EDGE_CURVE('',#16437,#16438,#4127,.T.);
#21160=EDGE_CURVE('',#16439,#16438,#4128,.T.);
#21161=EDGE_CURVE('',#16440,#16439,#4129,.T.);
#21162=EDGE_CURVE('',#16437,#16440,#4130,.T.);
#21163=EDGE_CURVE('',#16439,#16440,#10711,.T.);
#21164=EDGE_CURVE('',#16441,#16442,#472,.T.);
#21165=EDGE_CURVE('',#16441,#16443,#4131,.T.);
#21166=EDGE_CURVE('',#16444,#16443,#473,.T.);
#21167=EDGE_CURVE('',#16442,#16444,#4132,.T.);
#21168=EDGE_CURVE('',#16444,#16442,#10712,.T.);
#21169=EDGE_CURVE('',#16445,#16446,#10713,.T.);
#21170=EDGE_CURVE('',#16447,#16445,#10714,.T.);
#21171=EDGE_CURVE('',#16447,#16448,#4133,.T.);
#21172=EDGE_CURVE('',#16449,#16448,#10715,.T.);
#21173=EDGE_CURVE('',#16450,#16449,#10716,.T.);
#21174=EDGE_CURVE('',#16446,#16450,#4134,.T.);
#21175=EDGE_CURVE('',#16451,#16452,#10717,.T.);
#21176=EDGE_CURVE('',#16453,#16451,#4135,.T.);
#21177=EDGE_CURVE('',#16454,#16453,#10718,.T.);
#21178=EDGE_CURVE('',#16455,#16454,#10719,.T.);
#21179=EDGE_CURVE('',#16455,#16456,#4136,.T.);
#21180=EDGE_CURVE('',#16452,#16456,#10720,.T.);
#21181=EDGE_CURVE('',#16457,#16458,#10721,.T.);
#21182=EDGE_CURVE('',#16459,#16457,#4137,.T.);
#21183=EDGE_CURVE('',#16460,#16459,#10722,.T.);
#21184=EDGE_CURVE('',#16461,#16460,#10723,.T.);
#21185=EDGE_CURVE('',#16461,#16462,#4138,.T.);
#21186=EDGE_CURVE('',#16458,#16462,#10724,.T.);
#21187=EDGE_CURVE('',#16463,#16463,#4139,.T.);
#21188=EDGE_CURVE('',#16464,#16464,#4140,.T.);
#21189=EDGE_CURVE('',#16464,#16465,#10725,.T.);
#21190=EDGE_CURVE('',#16465,#16466,#4141,.T.);
#21191=EDGE_CURVE('',#16466,#16465,#4142,.T.);
#21192=EDGE_CURVE('',#16467,#16177,#10726,.T.);
#21193=EDGE_CURVE('',#16184,#16468,#10727,.T.);
#21194=EDGE_CURVE('',#16468,#16467,#10728,.T.);
#21195=EDGE_CURVE('',#16178,#16469,#10729,.T.);
#21196=EDGE_CURVE('',#16469,#16470,#10730,.T.);
#21197=EDGE_CURVE('',#16470,#16179,#10731,.T.);
#21198=EDGE_CURVE('',#16471,#16183,#10732,.T.);
#21199=EDGE_CURVE('',#16182,#16472,#10733,.T.);
#21200=EDGE_CURVE('',#16472,#16471,#10734,.T.);
#21201=EDGE_CURVE('',#16473,#16181,#10735,.T.);
#21202=EDGE_CURVE('',#16180,#16474,#10736,.T.);
#21203=EDGE_CURVE('',#16474,#16473,#10737,.T.);
#21204=EDGE_CURVE('',#16475,#16441,#10738,.T.);
#21205=EDGE_CURVE('',#16443,#16476,#10739,.T.);
#21206=EDGE_CURVE('',#16450,#16476,#10740,.T.);
#21207=EDGE_CURVE('',#16449,#16477,#10741,.T.);
#21208=EDGE_CURVE('',#16478,#16477,#10742,.T.);
#21209=EDGE_CURVE('',#16478,#16454,#10743,.T.);
#21210=EDGE_CURVE('',#16453,#16475,#10744,.T.);
#21211=EDGE_CURVE('',#16451,#16479,#10745,.T.);
#21212=EDGE_CURVE('',#16479,#16475,#4143,.T.);
#21213=EDGE_CURVE('',#16480,#16437,#10746,.T.);
#21214=EDGE_CURVE('',#16438,#16479,#10747,.T.);
#21215=EDGE_CURVE('',#16452,#16481,#10748,.T.);
#21216=EDGE_CURVE('',#16482,#16481,#10749,.T.);
#21217=EDGE_CURVE('',#16482,#16460,#10750,.T.);
#21218=EDGE_CURVE('',#16459,#16480,#10751,.T.);
#21219=EDGE_CURVE('',#16457,#16483,#10752,.T.);
#21220=EDGE_CURVE('',#16483,#16480,#4144,.T.);
#21221=EDGE_CURVE('',#16484,#16433,#10753,.T.);
#21222=EDGE_CURVE('',#16434,#16483,#10754,.T.);
#21223=EDGE_CURVE('',#16458,#16485,#10755,.T.);
#21224=EDGE_CURVE('',#16486,#16485,#10756,.T.);
#21225=EDGE_CURVE('',#16486,#16487,#10757,.T.);
#21226=EDGE_CURVE('',#16487,#16488,#10758,.T.);
#21227=EDGE_CURVE('',#16488,#16484,#10759,.T.);
#21228=EDGE_CURVE('',#16488,#16489,#4145,.T.);
#21229=EDGE_CURVE('',#16489,#16490,#10760,.T.);
#21230=EDGE_CURVE('',#16490,#16484,#4146,.T.);
#21231=EDGE_CURVE('',#16491,#16492,#10761,.T.);
#21232=EDGE_CURVE('',#16492,#16493,#4147,.T.);
#21233=EDGE_CURVE('',#16494,#16493,#10762,.T.);
#21234=EDGE_CURVE('',#16494,#16495,#4148,.T.);
#21235=EDGE_CURVE('',#16495,#16490,#10763,.T.);
#21236=EDGE_CURVE('',#16489,#16496,#10764,.T.);
#21237=EDGE_CURVE('',#16496,#16497,#10765,.T.);
#21238=EDGE_CURVE('',#16498,#16497,#10766,.T.);
#21239=EDGE_CURVE('',#16498,#16445,#10767,.T.);
#21240=EDGE_CURVE('',#16446,#16491,#10768,.T.);
#21241=EDGE_CURVE('',#16476,#16491,#4149,.T.);
#21242=EDGE_CURVE('',#16499,#16498,#10769,.T.);
#21243=EDGE_CURVE('',#16500,#16497,#10770,.T.);
#21244=EDGE_CURVE('',#16501,#16500,#4150,.T.);
#21245=EDGE_CURVE('',#16501,#16486,#10771,.T.);
#21246=EDGE_CURVE('',#16502,#16485,#10772,.T.);
#21247=EDGE_CURVE('',#16503,#16502,#4151,.T.);
#21248=EDGE_CURVE('',#16503,#16482,#10773,.T.);
#21249=EDGE_CURVE('',#16504,#16481,#10774,.T.);
#21250=EDGE_CURVE('',#16505,#16504,#4152,.T.);
#21251=EDGE_CURVE('',#16505,#16478,#10775,.T.);
#21252=EDGE_CURVE('',#16506,#16477,#10776,.T.);
#21253=EDGE_CURVE('',#16499,#16506,#4153,.T.);
#21254=EDGE_CURVE('',#16496,#16507,#10777,.T.);
#21255=EDGE_CURVE('',#16507,#16500,#10778,.T.);
#21256=EDGE_CURVE('',#16508,#16507,#4154,.T.);
#21257=EDGE_CURVE('',#16508,#16501,#10779,.T.);
#21258=EDGE_CURVE('',#16508,#16487,#10780,.T.);
#21259=EDGE_CURVE('',#16462,#16502,#10781,.T.);
#21260=EDGE_CURVE('',#16461,#16503,#10782,.T.);
#21261=EDGE_CURVE('',#16456,#16504,#10783,.T.);
#21262=EDGE_CURVE('',#16455,#16505,#10784,.T.);
#21263=EDGE_CURVE('',#16448,#16506,#10785,.T.);
#21264=EDGE_CURVE('',#16447,#16499,#10786,.T.);
#21265=EDGE_CURVE('',#16492,#16495,#4155,.T.);
#21266=EDGE_CURVE('',#16493,#16494,#4156,.T.);
#21267=EDGE_CURVE('',#16509,#16510,#4157,.T.);
#21268=EDGE_CURVE('',#16511,#16510,#10787,.T.);
#21269=EDGE_CURVE('',#16512,#16511,#4158,.T.);
#21270=EDGE_CURVE('',#16512,#16509,#10788,.T.);
#21271=EDGE_CURVE('',#16510,#16513,#10789,.T.);
#21272=EDGE_CURVE('',#16514,#16513,#10790,.T.);
#21273=EDGE_CURVE('',#16511,#16514,#10791,.T.);
#21274=EDGE_CURVE('',#16513,#16515,#4159,.T.);
#21275=EDGE_CURVE('',#16516,#16515,#10792,.T.);
#21276=EDGE_CURVE('',#16514,#16516,#4160,.T.);
#21277=EDGE_CURVE('',#16517,#16515,#4161,.T.);
#21278=EDGE_CURVE('',#16518,#16517,#10793,.T.);
#21279=EDGE_CURVE('',#16518,#16516,#4162,.T.);
#21280=EDGE_CURVE('',#16517,#16519,#4163,.T.);
#21281=EDGE_CURVE('',#16520,#16519,#10794,.T.);
#21282=EDGE_CURVE('',#16518,#16520,#4164,.T.);
#21283=EDGE_CURVE('',#16519,#16521,#10795,.T.);
#21284=EDGE_CURVE('',#16522,#16521,#10796,.T.);
#21285=EDGE_CURVE('',#16520,#16522,#10797,.T.);
#21286=EDGE_CURVE('',#16521,#16523,#4165,.T.);
#21287=EDGE_CURVE('',#16524,#16523,#10798,.T.);
#21288=EDGE_CURVE('',#16522,#16524,#4166,.T.);
#21289=EDGE_CURVE('',#16523,#16509,#4167,.T.);
#21290=EDGE_CURVE('',#16524,#16512,#4168,.T.);
#21291=EDGE_CURVE('',#16525,#16526,#10799,.T.);
#21292=EDGE_CURVE('',#16527,#16526,#10800,.T.);
#21293=EDGE_CURVE('',#16528,#16527,#10801,.T.);
#21294=EDGE_CURVE('',#16528,#16525,#10802,.T.);
#21295=EDGE_CURVE('',#16526,#16529,#4169,.T.);
#21296=EDGE_CURVE('',#16530,#16529,#10803,.T.);
#21297=EDGE_CURVE('',#16527,#16530,#4170,.T.);
#21298=EDGE_CURVE('',#16531,#16529,#4171,.T.);
#21299=EDGE_CURVE('',#16532,#16531,#10804,.T.);
#21300=EDGE_CURVE('',#16532,#16530,#4172,.T.);
#21301=EDGE_CURVE('',#16531,#16533,#4173,.T.);
#21302=EDGE_CURVE('',#16534,#16533,#10805,.T.);
#21303=EDGE_CURVE('',#16532,#16534,#4174,.T.);
#21304=EDGE_CURVE('',#16533,#16535,#10806,.T.);
#21305=EDGE_CURVE('',#16536,#16535,#10807,.T.);
#21306=EDGE_CURVE('',#16534,#16536,#10808,.T.);
#21307=EDGE_CURVE('',#16535,#16537,#4175,.T.);
#21308=EDGE_CURVE('',#16538,#16537,#10809,.T.);
#21309=EDGE_CURVE('',#16536,#16538,#4176,.T.);
#21310=EDGE_CURVE('',#16537,#16539,#4177,.T.);
#21311=EDGE_CURVE('',#16540,#16539,#10810,.T.);
#21312=EDGE_CURVE('',#16538,#16540,#4178,.T.);
#21313=EDGE_CURVE('',#16539,#16525,#4179,.T.);
#21314=EDGE_CURVE('',#16540,#16528,#4180,.T.);
#21315=EDGE_CURVE('',#16541,#16542,#4181,.T.);
#21316=EDGE_CURVE('',#16543,#16542,#10811,.T.);
#21317=EDGE_CURVE('',#16544,#16543,#4182,.T.);
#21318=EDGE_CURVE('',#16544,#16541,#10812,.T.);
#21319=EDGE_CURVE('',#16542,#16545,#4183,.T.);
#21320=EDGE_CURVE('',#16546,#16545,#10813,.T.);
#21321=EDGE_CURVE('',#16543,#16546,#4184,.T.);
#21322=EDGE_CURVE('',#16545,#16547,#10814,.T.);
#21323=EDGE_CURVE('',#16548,#16547,#10815,.T.);
#21324=EDGE_CURVE('',#16546,#16548,#10816,.T.);
#21325=EDGE_CURVE('',#16547,#16549,#4185,.T.);
#21326=EDGE_CURVE('',#16550,#16549,#10817,.T.);
#21327=EDGE_CURVE('',#16548,#16550,#4186,.T.);
#21328=EDGE_CURVE('',#16551,#16549,#4187,.T.);
#21329=EDGE_CURVE('',#16552,#16551,#10818,.T.);
#21330=EDGE_CURVE('',#16552,#16550,#4188,.T.);
#21331=EDGE_CURVE('',#16551,#16553,#4189,.T.);
#21332=EDGE_CURVE('',#16554,#16553,#10819,.T.);
#21333=EDGE_CURVE('',#16552,#16554,#4190,.T.);
#21334=EDGE_CURVE('',#16553,#16555,#10820,.T.);
#21335=EDGE_CURVE('',#16556,#16555,#10821,.T.);
#21336=EDGE_CURVE('',#16554,#16556,#10822,.T.);
#21337=EDGE_CURVE('',#16555,#16541,#4191,.T.);
#21338=EDGE_CURVE('',#16556,#16544,#4192,.T.);
#21339=EDGE_CURVE('',#16557,#16558,#4193,.T.);
#21340=EDGE_CURVE('',#16559,#16558,#10823,.T.);
#21341=EDGE_CURVE('',#16560,#16559,#4194,.T.);
#21342=EDGE_CURVE('',#16560,#16557,#10824,.T.);
#21343=EDGE_CURVE('',#16558,#16561,#4195,.T.);
#21344=EDGE_CURVE('',#16562,#16561,#10825,.T.);
#21345=EDGE_CURVE('',#16559,#16562,#4196,.T.);
#21346=EDGE_CURVE('',#16561,#16563,#10826,.T.);
#21347=EDGE_CURVE('',#16564,#16563,#10827,.T.);
#21348=EDGE_CURVE('',#16562,#16564,#10828,.T.);
#21349=EDGE_CURVE('',#16563,#16565,#4197,.T.);
#21350=EDGE_CURVE('',#16566,#16565,#10829,.T.);
#21351=EDGE_CURVE('',#16564,#16566,#4198,.T.);
#21352=EDGE_CURVE('',#16567,#16565,#4199,.T.);
#21353=EDGE_CURVE('',#16568,#16567,#10830,.T.);
#21354=EDGE_CURVE('',#16568,#16566,#4200,.T.);
#21355=EDGE_CURVE('',#16567,#16569,#4201,.T.);
#21356=EDGE_CURVE('',#16570,#16569,#10831,.T.);
#21357=EDGE_CURVE('',#16568,#16570,#4202,.T.);
#21358=EDGE_CURVE('',#16569,#16571,#10832,.T.);
#21359=EDGE_CURVE('',#16572,#16571,#10833,.T.);
#21360=EDGE_CURVE('',#16570,#16572,#10834,.T.);
#21361=EDGE_CURVE('',#16571,#16557,#4203,.T.);
#21362=EDGE_CURVE('',#16572,#16560,#4204,.T.);
#21363=EDGE_CURVE('',#16573,#16574,#4205,.T.);
#21364=EDGE_CURVE('',#16374,#16573,#10835,.T.);
#21365=EDGE_CURVE('',#16375,#16574,#10836,.T.);
#21366=EDGE_CURVE('',#16575,#16574,#4206,.T.);
#21367=EDGE_CURVE('',#16381,#16575,#10837,.T.);
#21368=EDGE_CURVE('',#16576,#16575,#10838,.T.);
#21369=EDGE_CURVE('',#16380,#16576,#10839,.T.);
#21370=EDGE_CURVE('',#16577,#16576,#4207,.T.);
#21371=EDGE_CURVE('',#16379,#16577,#10840,.T.);
#21372=EDGE_CURVE('',#16578,#16577,#4208,.T.);
#21373=EDGE_CURVE('',#16378,#16578,#10841,.T.);
#21374=EDGE_CURVE('',#16579,#16578,#4209,.T.);
#21375=EDGE_CURVE('',#16377,#16579,#10842,.T.);
#21376=EDGE_CURVE('',#16573,#16580,#4210,.T.);
#21377=EDGE_CURVE('',#16376,#16580,#10843,.T.);
#21378=EDGE_CURVE('',#16580,#16579,#10844,.T.);
#21379=EDGE_CURVE('',#16466,#16581,#4211,.T.);
#21380=EDGE_CURVE('',#16581,#16581,#4212,.T.);
#21381=EDGE_CURVE('',#16582,#16583,#10845,.T.);
#21382=EDGE_CURVE('',#16583,#16584,#10846,.T.);
#21383=EDGE_CURVE('',#16584,#16585,#10847,.T.);
#21384=EDGE_CURVE('',#16585,#16586,#10848,.T.);
#21385=EDGE_CURVE('',#16586,#16587,#10849,.T.);
#21386=EDGE_CURVE('',#16587,#16588,#10850,.T.);
#21387=EDGE_CURVE('',#16588,#16589,#10851,.T.);
#21388=EDGE_CURVE('',#16589,#16582,#10852,.T.);
#21389=EDGE_CURVE('',#16582,#16468,#10853,.T.);
#21390=EDGE_CURVE('',#16589,#16467,#10854,.T.);
#21391=EDGE_CURVE('',#16588,#16469,#10855,.T.);
#21392=EDGE_CURVE('',#16587,#16470,#10856,.T.);
#21393=EDGE_CURVE('',#16585,#16473,#10857,.T.);
#21394=EDGE_CURVE('',#16584,#16472,#10858,.T.);
#21395=EDGE_CURVE('',#16583,#16471,#10859,.T.);
#21396=EDGE_CURVE('',#16586,#16474,#10860,.T.);
#21397=EDGE_CURVE('',#16590,#16591,#4213,.T.);
#21398=EDGE_CURVE('',#16591,#16590,#4214,.T.);
#21399=EDGE_CURVE('',#16591,#16592,#10861,.T.);
#21400=EDGE_CURVE('',#16592,#16592,#4215,.T.);
#21401=EDGE_CURVE('',#16590,#16593,#10862,.T.);
#21402=EDGE_CURVE('',#16594,#16593,#4216,.T.);
#21403=EDGE_CURVE('',#16593,#16594,#4217,.T.);
#21404=EDGE_CURVE('',#16594,#16463,#10863,.T.);
#21405=EDGE_CURVE('',#16595,#16596,#10864,.T.);
#21406=EDGE_CURVE('',#16597,#16596,#10865,.T.);
#21407=EDGE_CURVE('',#16598,#16597,#10866,.T.);
#21408=EDGE_CURVE('',#16598,#16595,#10867,.T.);
#21409=EDGE_CURVE('',#16596,#16599,#10868,.T.);
#21410=EDGE_CURVE('',#16600,#16599,#10869,.T.);
#21411=EDGE_CURVE('',#16597,#16600,#10870,.T.);
#21412=EDGE_CURVE('',#16599,#16601,#10871,.T.);
#21413=EDGE_CURVE('',#16602,#16601,#10872,.T.);
#21414=EDGE_CURVE('',#16600,#16602,#10873,.T.);
#21415=EDGE_CURVE('',#16603,#16601,#10874,.T.);
#21416=EDGE_CURVE('',#16604,#16603,#10875,.T.);
#21417=EDGE_CURVE('',#16602,#16604,#10876,.T.);
#21418=EDGE_CURVE('',#16603,#16605,#10877,.T.);
#21419=EDGE_CURVE('',#16606,#16605,#10878,.T.);
#21420=EDGE_CURVE('',#16604,#16606,#10879,.T.);
#21421=EDGE_CURVE('',#16606,#16598,#10880,.T.);
#21422=EDGE_CURVE('',#16605,#16595,#10881,.T.);
#28770=ORIENTED_EDGE('',*,*,#20287,.F.);
#28771=ORIENTED_EDGE('',*,*,#20288,.F.);
#28772=ORIENTED_EDGE('',*,*,#20289,.T.);
#28773=ORIENTED_EDGE('',*,*,#20290,.F.);
#28774=ORIENTED_EDGE('',*,*,#20289,.F.);
#28775=ORIENTED_EDGE('',*,*,#20290,.T.);
#28776=ORIENTED_EDGE('',*,*,#20291,.T.);
#28777=ORIENTED_EDGE('',*,*,#20292,.F.);
#28778=ORIENTED_EDGE('',*,*,#20293,.F.);
#28779=ORIENTED_EDGE('',*,*,#20291,.F.);
#28780=ORIENTED_EDGE('',*,*,#20293,.T.);
#28781=ORIENTED_EDGE('',*,*,#20294,.T.);
#28782=ORIENTED_EDGE('',*,*,#20287,.T.);
#28783=ORIENTED_EDGE('',*,*,#20288,.T.);
#28784=ORIENTED_EDGE('',*,*,#20294,.F.);
#28785=ORIENTED_EDGE('',*,*,#20292,.T.);
#28786=ORIENTED_EDGE('',*,*,#20295,.T.);
#28787=ORIENTED_EDGE('',*,*,#20296,.T.);
#28788=ORIENTED_EDGE('',*,*,#20297,.F.);
#28789=ORIENTED_EDGE('',*,*,#20296,.F.);
#28790=ORIENTED_EDGE('',*,*,#20298,.T.);
#28791=ORIENTED_EDGE('',*,*,#20295,.F.);
#28792=ORIENTED_EDGE('',*,*,#20299,.T.);
#28793=ORIENTED_EDGE('',*,*,#20297,.T.);
#28794=ORIENTED_EDGE('',*,*,#20298,.F.);
#28795=ORIENTED_EDGE('',*,*,#20300,.T.);
#28796=ORIENTED_EDGE('',*,*,#20299,.F.);
#28797=ORIENTED_EDGE('',*,*,#20300,.F.);
#28798=ORIENTED_EDGE('',*,*,#20301,.F.);
#28799=ORIENTED_EDGE('',*,*,#20302,.F.);
#28800=ORIENTED_EDGE('',*,*,#20303,.T.);
#28801=ORIENTED_EDGE('',*,*,#20304,.F.);
#28802=ORIENTED_EDGE('',*,*,#20303,.F.);
#28803=ORIENTED_EDGE('',*,*,#20304,.T.);
#28804=ORIENTED_EDGE('',*,*,#20305,.T.);
#28805=ORIENTED_EDGE('',*,*,#20306,.F.);
#28806=ORIENTED_EDGE('',*,*,#20307,.F.);
#28807=ORIENTED_EDGE('',*,*,#20305,.F.);
#28808=ORIENTED_EDGE('',*,*,#20307,.T.);
#28809=ORIENTED_EDGE('',*,*,#20308,.T.);
#28810=ORIENTED_EDGE('',*,*,#20301,.T.);
#28811=ORIENTED_EDGE('',*,*,#20302,.T.);
#28812=ORIENTED_EDGE('',*,*,#20308,.F.);
#28813=ORIENTED_EDGE('',*,*,#20306,.T.);
#28814=ORIENTED_EDGE('',*,*,#20309,.T.);
#28815=ORIENTED_EDGE('',*,*,#20310,.T.);
#28816=ORIENTED_EDGE('',*,*,#20311,.F.);
#28817=ORIENTED_EDGE('',*,*,#20310,.F.);
#28818=ORIENTED_EDGE('',*,*,#20312,.T.);
#28819=ORIENTED_EDGE('',*,*,#20309,.F.);
#28820=ORIENTED_EDGE('',*,*,#20313,.T.);
#28821=ORIENTED_EDGE('',*,*,#20311,.T.);
#28822=ORIENTED_EDGE('',*,*,#20312,.F.);
#28823=ORIENTED_EDGE('',*,*,#20314,.T.);
#28824=ORIENTED_EDGE('',*,*,#20313,.F.);
#28825=ORIENTED_EDGE('',*,*,#20314,.F.);
#28826=ORIENTED_EDGE('',*,*,#20315,.F.);
#28827=ORIENTED_EDGE('',*,*,#20316,.T.);
#28828=ORIENTED_EDGE('',*,*,#20317,.F.);
#28829=ORIENTED_EDGE('',*,*,#20316,.F.);
#28830=ORIENTED_EDGE('',*,*,#20318,.F.);
#28831=ORIENTED_EDGE('',*,*,#20317,.T.);
#28832=ORIENTED_EDGE('',*,*,#20319,.T.);
#28833=ORIENTED_EDGE('',*,*,#20320,.T.);
#28834=ORIENTED_EDGE('',*,*,#20321,.T.);
#28835=ORIENTED_EDGE('',*,*,#20318,.T.);
#28836=ORIENTED_EDGE('',*,*,#20315,.T.);
#28837=ORIENTED_EDGE('',*,*,#20321,.F.);
#28838=ORIENTED_EDGE('',*,*,#20322,.T.);
#28839=ORIENTED_EDGE('',*,*,#20319,.F.);
#28840=ORIENTED_EDGE('',*,*,#20320,.F.);
#28841=ORIENTED_EDGE('',*,*,#20322,.F.);
#28842=ORIENTED_EDGE('',*,*,#20323,.T.);
#28843=ORIENTED_EDGE('',*,*,#20324,.T.);
#28844=ORIENTED_EDGE('',*,*,#20325,.F.);
#28845=ORIENTED_EDGE('',*,*,#20324,.F.);
#28846=ORIENTED_EDGE('',*,*,#20326,.T.);
#28847=ORIENTED_EDGE('',*,*,#20323,.F.);
#28848=ORIENTED_EDGE('',*,*,#20327,.F.);
#28849=ORIENTED_EDGE('',*,*,#20328,.T.);
#28850=ORIENTED_EDGE('',*,*,#20326,.F.);
#28851=ORIENTED_EDGE('',*,*,#20328,.F.);
#28852=ORIENTED_EDGE('',*,*,#20327,.T.);
#28853=ORIENTED_EDGE('',*,*,#20325,.T.);
#28854=ORIENTED_EDGE('',*,*,#20329,.T.);
#28855=ORIENTED_EDGE('',*,*,#20330,.T.);
#28856=ORIENTED_EDGE('',*,*,#20331,.F.);
#28857=ORIENTED_EDGE('',*,*,#20330,.F.);
#28858=ORIENTED_EDGE('',*,*,#20332,.T.);
#28859=ORIENTED_EDGE('',*,*,#20329,.F.);
#28860=ORIENTED_EDGE('',*,*,#20332,.F.);
#28861=ORIENTED_EDGE('',*,*,#20333,.T.);
#28862=ORIENTED_EDGE('',*,*,#20334,.F.);
#28863=ORIENTED_EDGE('',*,*,#20333,.F.);
#28864=ORIENTED_EDGE('',*,*,#20334,.T.);
#28865=ORIENTED_EDGE('',*,*,#20331,.T.);
#28866=ORIENTED_EDGE('',*,*,#20335,.F.);
#28867=ORIENTED_EDGE('',*,*,#20336,.F.);
#28868=ORIENTED_EDGE('',*,*,#20337,.T.);
#28869=ORIENTED_EDGE('',*,*,#20338,.F.);
#28870=ORIENTED_EDGE('',*,*,#20337,.F.);
#28871=ORIENTED_EDGE('',*,*,#20338,.T.);
#28872=ORIENTED_EDGE('',*,*,#20339,.T.);
#28873=ORIENTED_EDGE('',*,*,#20340,.T.);
#28874=ORIENTED_EDGE('',*,*,#20341,.T.);
#28875=ORIENTED_EDGE('',*,*,#20335,.T.);
#28876=ORIENTED_EDGE('',*,*,#20336,.T.);
#28877=ORIENTED_EDGE('',*,*,#20341,.F.);
#28878=ORIENTED_EDGE('',*,*,#20342,.T.);
#28879=ORIENTED_EDGE('',*,*,#20339,.F.);
#28880=ORIENTED_EDGE('',*,*,#20340,.F.);
#28881=ORIENTED_EDGE('',*,*,#20342,.F.);
#28882=ORIENTED_EDGE('',*,*,#20343,.T.);
#28883=ORIENTED_EDGE('',*,*,#20344,.T.);
#28884=ORIENTED_EDGE('',*,*,#20345,.F.);
#28885=ORIENTED_EDGE('',*,*,#20344,.F.);
#28886=ORIENTED_EDGE('',*,*,#20346,.T.);
#28887=ORIENTED_EDGE('',*,*,#20343,.F.);
#28888=ORIENTED_EDGE('',*,*,#20346,.F.);
#28889=ORIENTED_EDGE('',*,*,#20347,.T.);
#28890=ORIENTED_EDGE('',*,*,#20348,.F.);
#28891=ORIENTED_EDGE('',*,*,#20347,.F.);
#28892=ORIENTED_EDGE('',*,*,#20348,.T.);
#28893=ORIENTED_EDGE('',*,*,#20345,.T.);
#28894=ORIENTED_EDGE('',*,*,#20349,.F.);
#28895=ORIENTED_EDGE('',*,*,#20350,.F.);
#28896=ORIENTED_EDGE('',*,*,#20351,.T.);
#28897=ORIENTED_EDGE('',*,*,#20352,.F.);
#28898=ORIENTED_EDGE('',*,*,#20351,.F.);
#28899=ORIENTED_EDGE('',*,*,#20352,.T.);
#28900=ORIENTED_EDGE('',*,*,#20353,.T.);
#28901=ORIENTED_EDGE('',*,*,#20354,.T.);
#28902=ORIENTED_EDGE('',*,*,#20355,.T.);
#28903=ORIENTED_EDGE('',*,*,#20349,.T.);
#28904=ORIENTED_EDGE('',*,*,#20350,.T.);
#28905=ORIENTED_EDGE('',*,*,#20355,.F.);
#28906=ORIENTED_EDGE('',*,*,#20356,.T.);
#28907=ORIENTED_EDGE('',*,*,#20353,.F.);
#28908=ORIENTED_EDGE('',*,*,#20354,.F.);
#28909=ORIENTED_EDGE('',*,*,#20356,.F.);
#28910=ORIENTED_EDGE('',*,*,#20357,.F.);
#28911=ORIENTED_EDGE('',*,*,#20358,.T.);
#28912=ORIENTED_EDGE('',*,*,#20359,.T.);
#28913=ORIENTED_EDGE('',*,*,#20360,.F.);
#28914=ORIENTED_EDGE('',*,*,#20361,.F.);
#28915=ORIENTED_EDGE('',*,*,#20362,.F.);
#28916=ORIENTED_EDGE('',*,*,#20363,.F.);
#28917=ORIENTED_EDGE('',*,*,#20364,.F.);
#28918=ORIENTED_EDGE('',*,*,#20365,.F.);
#28919=ORIENTED_EDGE('',*,*,#20366,.F.);
#28920=ORIENTED_EDGE('',*,*,#20367,.F.);
#28921=ORIENTED_EDGE('',*,*,#20368,.F.);
#28922=ORIENTED_EDGE('',*,*,#20369,.F.);
#28923=ORIENTED_EDGE('',*,*,#20370,.F.);
#28924=ORIENTED_EDGE('',*,*,#20371,.F.);
#28925=ORIENTED_EDGE('',*,*,#20372,.F.);
#28926=ORIENTED_EDGE('',*,*,#20373,.T.);
#28927=ORIENTED_EDGE('',*,*,#20374,.T.);
#28928=ORIENTED_EDGE('',*,*,#20375,.T.);
#28929=ORIENTED_EDGE('',*,*,#20376,.T.);
#28930=ORIENTED_EDGE('',*,*,#20376,.F.);
#28931=ORIENTED_EDGE('',*,*,#20377,.T.);
#28932=ORIENTED_EDGE('',*,*,#20378,.T.);
#28933=ORIENTED_EDGE('',*,*,#20379,.T.);
#28934=ORIENTED_EDGE('',*,*,#20380,.T.);
#28935=ORIENTED_EDGE('',*,*,#20381,.T.);
#28936=ORIENTED_EDGE('',*,*,#20382,.T.);
#28937=ORIENTED_EDGE('',*,*,#20383,.T.);
#28938=ORIENTED_EDGE('',*,*,#20383,.F.);
#28939=ORIENTED_EDGE('',*,*,#20384,.T.);
#28940=ORIENTED_EDGE('',*,*,#20385,.T.);
#28941=ORIENTED_EDGE('',*,*,#20386,.T.);
#28942=ORIENTED_EDGE('',*,*,#20387,.T.);
#28943=ORIENTED_EDGE('',*,*,#20388,.T.);
#28944=ORIENTED_EDGE('',*,*,#20374,.F.);
#28945=ORIENTED_EDGE('',*,*,#20389,.T.);
#28946=ORIENTED_EDGE('',*,*,#20390,.F.);
#28947=ORIENTED_EDGE('',*,*,#20370,.T.);
#28948=ORIENTED_EDGE('',*,*,#20391,.T.);
#28949=ORIENTED_EDGE('',*,*,#20392,.T.);
#28950=ORIENTED_EDGE('',*,*,#20375,.F.);
#28951=ORIENTED_EDGE('',*,*,#20392,.F.);
#28952=ORIENTED_EDGE('',*,*,#20393,.T.);
#28953=ORIENTED_EDGE('',*,*,#20394,.T.);
#28954=ORIENTED_EDGE('',*,*,#20395,.F.);
#28955=ORIENTED_EDGE('',*,*,#20362,.T.);
#28956=ORIENTED_EDGE('',*,*,#20396,.F.);
#28957=ORIENTED_EDGE('',*,*,#20377,.F.);
#28958=ORIENTED_EDGE('',*,*,#20382,.F.);
#28959=ORIENTED_EDGE('',*,*,#20397,.F.);
#28960=ORIENTED_EDGE('',*,*,#20398,.F.);
#28961=ORIENTED_EDGE('',*,*,#20399,.T.);
#28962=ORIENTED_EDGE('',*,*,#20400,.F.);
#28963=ORIENTED_EDGE('',*,*,#20401,.F.);
#28964=ORIENTED_EDGE('',*,*,#20402,.T.);
#28965=ORIENTED_EDGE('',*,*,#20384,.F.);
#28966=ORIENTED_EDGE('',*,*,#20381,.F.);
#28967=ORIENTED_EDGE('',*,*,#20403,.T.);
#28968=ORIENTED_EDGE('',*,*,#20404,.F.);
#28969=ORIENTED_EDGE('',*,*,#20397,.T.);
#28970=ORIENTED_EDGE('',*,*,#20373,.F.);
#28971=ORIENTED_EDGE('',*,*,#20379,.F.);
#28972=ORIENTED_EDGE('',*,*,#20405,.F.);
#28973=ORIENTED_EDGE('',*,*,#20406,.F.);
#28974=ORIENTED_EDGE('',*,*,#20407,.F.);
#28975=ORIENTED_EDGE('',*,*,#20408,.F.);
#28976=ORIENTED_EDGE('',*,*,#20409,.F.);
#28977=ORIENTED_EDGE('',*,*,#20403,.F.);
#28978=ORIENTED_EDGE('',*,*,#20380,.F.);
#28979=ORIENTED_EDGE('',*,*,#20388,.F.);
#28980=ORIENTED_EDGE('',*,*,#20410,.F.);
#28981=ORIENTED_EDGE('',*,*,#20411,.F.);
#28982=ORIENTED_EDGE('',*,*,#20412,.F.);
#28983=ORIENTED_EDGE('',*,*,#20413,.F.);
#28984=ORIENTED_EDGE('',*,*,#20414,.F.);
#28985=ORIENTED_EDGE('',*,*,#20389,.F.);
#28986=ORIENTED_EDGE('',*,*,#20415,.F.);
#28987=ORIENTED_EDGE('',*,*,#20416,.F.);
#28988=ORIENTED_EDGE('',*,*,#20417,.T.);
#28989=ORIENTED_EDGE('',*,*,#20418,.F.);
#28990=ORIENTED_EDGE('',*,*,#20419,.F.);
#28991=ORIENTED_EDGE('',*,*,#20417,.F.);
#28992=ORIENTED_EDGE('',*,*,#20406,.T.);
#28993=ORIENTED_EDGE('',*,*,#20420,.F.);
#28994=ORIENTED_EDGE('',*,*,#20360,.T.);
#28995=ORIENTED_EDGE('',*,*,#20421,.F.);
#28996=ORIENTED_EDGE('',*,*,#20421,.T.);
#28997=ORIENTED_EDGE('',*,*,#20359,.F.);
#28998=ORIENTED_EDGE('',*,*,#20422,.T.);
#28999=ORIENTED_EDGE('',*,*,#20423,.F.);
#29000=ORIENTED_EDGE('',*,*,#20424,.F.);
#29001=ORIENTED_EDGE('',*,*,#20425,.T.);
#29002=ORIENTED_EDGE('',*,*,#20426,.F.);
#29003=ORIENTED_EDGE('',*,*,#20427,.F.);
#29004=ORIENTED_EDGE('',*,*,#20407,.T.);
#29005=ORIENTED_EDGE('',*,*,#20416,.T.);
#29006=ORIENTED_EDGE('',*,*,#20428,.T.);
#29007=ORIENTED_EDGE('',*,*,#20429,.T.);
#29008=ORIENTED_EDGE('',*,*,#20430,.T.);
#29009=ORIENTED_EDGE('',*,*,#20428,.F.);
#29010=ORIENTED_EDGE('',*,*,#20431,.T.);
#29011=ORIENTED_EDGE('',*,*,#20432,.F.);
#29012=ORIENTED_EDGE('',*,*,#20433,.F.);
#29013=ORIENTED_EDGE('',*,*,#20431,.F.);
#29014=ORIENTED_EDGE('',*,*,#20434,.F.);
#29015=ORIENTED_EDGE('',*,*,#20435,.F.);
#29016=ORIENTED_EDGE('',*,*,#20408,.T.);
#29017=ORIENTED_EDGE('',*,*,#20427,.T.);
#29018=ORIENTED_EDGE('',*,*,#20436,.T.);
#29019=ORIENTED_EDGE('',*,*,#20424,.T.);
#29020=ORIENTED_EDGE('',*,*,#20437,.F.);
#29021=ORIENTED_EDGE('',*,*,#20438,.F.);
#29022=ORIENTED_EDGE('',*,*,#20439,.F.);
#29023=ORIENTED_EDGE('',*,*,#20440,.F.);
#29024=ORIENTED_EDGE('',*,*,#20441,.F.);
#29025=ORIENTED_EDGE('',*,*,#20442,.F.);
#29026=ORIENTED_EDGE('',*,*,#20443,.F.);
#29027=ORIENTED_EDGE('',*,*,#20444,.F.);
#29028=ORIENTED_EDGE('',*,*,#20445,.F.);
#29029=ORIENTED_EDGE('',*,*,#20430,.F.);
#29030=ORIENTED_EDGE('',*,*,#20446,.T.);
#29031=ORIENTED_EDGE('',*,*,#20447,.F.);
#29032=ORIENTED_EDGE('',*,*,#20448,.F.);
#29033=ORIENTED_EDGE('',*,*,#20446,.F.);
#29034=ORIENTED_EDGE('',*,*,#20436,.F.);
#29035=ORIENTED_EDGE('',*,*,#20449,.F.);
#29036=ORIENTED_EDGE('',*,*,#20450,.T.);
#29037=ORIENTED_EDGE('',*,*,#20425,.F.);
#29038=ORIENTED_EDGE('',*,*,#20358,.F.);
#29039=ORIENTED_EDGE('',*,*,#20451,.F.);
#29040=ORIENTED_EDGE('',*,*,#20452,.T.);
#29041=ORIENTED_EDGE('',*,*,#20422,.F.);
#29042=ORIENTED_EDGE('',*,*,#20429,.F.);
#29043=ORIENTED_EDGE('',*,*,#20453,.T.);
#29044=ORIENTED_EDGE('',*,*,#20454,.F.);
#29045=ORIENTED_EDGE('',*,*,#20455,.F.);
#29046=ORIENTED_EDGE('',*,*,#20453,.F.);
#29047=ORIENTED_EDGE('',*,*,#20452,.F.);
#29048=ORIENTED_EDGE('',*,*,#20456,.F.);
#29049=ORIENTED_EDGE('',*,*,#20457,.F.);
#29050=ORIENTED_EDGE('',*,*,#20458,.F.);
#29051=ORIENTED_EDGE('',*,*,#20459,.F.);
#29052=ORIENTED_EDGE('',*,*,#20441,.T.);
#29053=ORIENTED_EDGE('',*,*,#20460,.F.);
#29054=ORIENTED_EDGE('',*,*,#20439,.T.);
#29055=ORIENTED_EDGE('',*,*,#20461,.F.);
#29056=ORIENTED_EDGE('',*,*,#20437,.T.);
#29057=ORIENTED_EDGE('',*,*,#20423,.T.);
#29058=ORIENTED_EDGE('',*,*,#20426,.T.);
#29059=ORIENTED_EDGE('',*,*,#20450,.F.);
#29060=ORIENTED_EDGE('',*,*,#20462,.F.);
#29061=ORIENTED_EDGE('',*,*,#20463,.F.);
#29062=ORIENTED_EDGE('',*,*,#20464,.F.);
#29063=ORIENTED_EDGE('',*,*,#20465,.T.);
#29064=ORIENTED_EDGE('',*,*,#20466,.F.);
#29065=ORIENTED_EDGE('',*,*,#20386,.F.);
#29066=ORIENTED_EDGE('',*,*,#20467,.F.);
#29067=ORIENTED_EDGE('',*,*,#20468,.F.);
#29068=ORIENTED_EDGE('',*,*,#20469,.F.);
#29069=ORIENTED_EDGE('',*,*,#20470,.F.);
#29070=ORIENTED_EDGE('',*,*,#20471,.F.);
#29071=ORIENTED_EDGE('',*,*,#20472,.F.);
#29072=ORIENTED_EDGE('',*,*,#20473,.F.);
#29073=ORIENTED_EDGE('',*,*,#20399,.F.);
#29074=ORIENTED_EDGE('',*,*,#20474,.F.);
#29075=ORIENTED_EDGE('',*,*,#20434,.T.);
#29076=ORIENTED_EDGE('',*,*,#20475,.T.);
#29077=ORIENTED_EDGE('',*,*,#20476,.T.);
#29078=ORIENTED_EDGE('',*,*,#20477,.F.);
#29079=ORIENTED_EDGE('',*,*,#20478,.F.);
#29080=ORIENTED_EDGE('',*,*,#20476,.F.);
#29081=ORIENTED_EDGE('',*,*,#20479,.T.);
#29082=ORIENTED_EDGE('',*,*,#20480,.F.);
#29083=ORIENTED_EDGE('',*,*,#20481,.F.);
#29084=ORIENTED_EDGE('',*,*,#20482,.F.);
#29085=ORIENTED_EDGE('',*,*,#20483,.F.);
#29086=ORIENTED_EDGE('',*,*,#20484,.T.);
#29087=ORIENTED_EDGE('',*,*,#20485,.T.);
#29088=ORIENTED_EDGE('',*,*,#20486,.T.);
#29089=ORIENTED_EDGE('',*,*,#20485,.F.);
#29090=ORIENTED_EDGE('',*,*,#20487,.T.);
#29091=ORIENTED_EDGE('',*,*,#20488,.F.);
#29092=ORIENTED_EDGE('',*,*,#20489,.F.);
#29093=ORIENTED_EDGE('',*,*,#20490,.F.);
#29094=ORIENTED_EDGE('',*,*,#20491,.F.);
#29095=ORIENTED_EDGE('',*,*,#20489,.T.);
#29096=ORIENTED_EDGE('',*,*,#20492,.F.);
#29097=ORIENTED_EDGE('',*,*,#20493,.T.);
#29098=ORIENTED_EDGE('',*,*,#20490,.T.);
#29099=ORIENTED_EDGE('',*,*,#20493,.F.);
#29100=ORIENTED_EDGE('',*,*,#20494,.F.);
#29101=ORIENTED_EDGE('',*,*,#20495,.F.);
#29102=ORIENTED_EDGE('',*,*,#20496,.T.);
#29103=ORIENTED_EDGE('',*,*,#20497,.T.);
#29104=ORIENTED_EDGE('',*,*,#20498,.F.);
#29105=ORIENTED_EDGE('',*,*,#20499,.F.);
#29106=ORIENTED_EDGE('',*,*,#20500,.T.);
#29107=ORIENTED_EDGE('',*,*,#20501,.T.);
#29108=ORIENTED_EDGE('',*,*,#20496,.F.);
#29109=ORIENTED_EDGE('',*,*,#20502,.F.);
#29110=ORIENTED_EDGE('',*,*,#20503,.T.);
#29111=ORIENTED_EDGE('',*,*,#20504,.T.);
#29112=ORIENTED_EDGE('',*,*,#20500,.F.);
#29113=ORIENTED_EDGE('',*,*,#20505,.F.);
#29114=ORIENTED_EDGE('',*,*,#20479,.F.);
#29115=ORIENTED_EDGE('',*,*,#20475,.F.);
#29116=ORIENTED_EDGE('',*,*,#20506,.F.);
#29117=ORIENTED_EDGE('',*,*,#20507,.T.);
#29118=ORIENTED_EDGE('',*,*,#20508,.F.);
#29119=ORIENTED_EDGE('',*,*,#20487,.F.);
#29120=ORIENTED_EDGE('',*,*,#20484,.F.);
#29121=ORIENTED_EDGE('',*,*,#20509,.F.);
#29122=ORIENTED_EDGE('',*,*,#20507,.F.);
#29123=ORIENTED_EDGE('',*,*,#20510,.T.);
#29124=ORIENTED_EDGE('',*,*,#20511,.T.);
#29125=ORIENTED_EDGE('',*,*,#20512,.T.);
#29126=ORIENTED_EDGE('',*,*,#20513,.T.);
#29127=ORIENTED_EDGE('',*,*,#20514,.F.);
#29128=ORIENTED_EDGE('',*,*,#20513,.F.);
#29129=ORIENTED_EDGE('',*,*,#20515,.T.);
#29130=ORIENTED_EDGE('',*,*,#20516,.T.);
#29131=ORIENTED_EDGE('',*,*,#20517,.T.);
#29132=ORIENTED_EDGE('',*,*,#20518,.F.);
#29133=ORIENTED_EDGE('',*,*,#20517,.F.);
#29134=ORIENTED_EDGE('',*,*,#20519,.T.);
#29135=ORIENTED_EDGE('',*,*,#20520,.T.);
#29136=ORIENTED_EDGE('',*,*,#20521,.T.);
#29137=ORIENTED_EDGE('',*,*,#20522,.F.);
#29138=ORIENTED_EDGE('',*,*,#20521,.F.);
#29139=ORIENTED_EDGE('',*,*,#20523,.T.);
#29140=ORIENTED_EDGE('',*,*,#20524,.T.);
#29141=ORIENTED_EDGE('',*,*,#20525,.T.);
#29142=ORIENTED_EDGE('',*,*,#20526,.F.);
#29143=ORIENTED_EDGE('',*,*,#20525,.F.);
#29144=ORIENTED_EDGE('',*,*,#20491,.T.);
#29145=ORIENTED_EDGE('',*,*,#20494,.T.);
#29146=ORIENTED_EDGE('',*,*,#20492,.T.);
#29147=ORIENTED_EDGE('',*,*,#20488,.T.);
#29148=ORIENTED_EDGE('',*,*,#20508,.T.);
#29149=ORIENTED_EDGE('',*,*,#20509,.T.);
#29150=ORIENTED_EDGE('',*,*,#20506,.T.);
#29151=ORIENTED_EDGE('',*,*,#20482,.T.);
#29152=ORIENTED_EDGE('',*,*,#20527,.T.);
#29153=ORIENTED_EDGE('',*,*,#20528,.F.);
#29154=ORIENTED_EDGE('',*,*,#20529,.F.);
#29155=ORIENTED_EDGE('',*,*,#20530,.F.);
#29156=ORIENTED_EDGE('',*,*,#20531,.F.);
#29157=ORIENTED_EDGE('',*,*,#20481,.T.);
#29158=ORIENTED_EDGE('',*,*,#20532,.F.);
#29159=ORIENTED_EDGE('',*,*,#20533,.F.);
#29160=ORIENTED_EDGE('',*,*,#20534,.F.);
#29161=ORIENTED_EDGE('',*,*,#20535,.F.);
#29162=ORIENTED_EDGE('',*,*,#20527,.F.);
#29163=ORIENTED_EDGE('',*,*,#20536,.F.);
#29164=ORIENTED_EDGE('',*,*,#20537,.F.);
#29165=ORIENTED_EDGE('',*,*,#20538,.F.);
#29166=ORIENTED_EDGE('',*,*,#20502,.T.);
#29167=ORIENTED_EDGE('',*,*,#20499,.T.);
#29168=ORIENTED_EDGE('',*,*,#20495,.T.);
#29169=ORIENTED_EDGE('',*,*,#20539,.T.);
#29170=ORIENTED_EDGE('',*,*,#20540,.T.);
#29171=ORIENTED_EDGE('',*,*,#20541,.T.);
#29172=ORIENTED_EDGE('',*,*,#20542,.T.);
#29173=ORIENTED_EDGE('',*,*,#20543,.T.);
#29174=ORIENTED_EDGE('',*,*,#20544,.T.);
#29175=ORIENTED_EDGE('',*,*,#20545,.T.);
#29176=ORIENTED_EDGE('',*,*,#20546,.F.);
#29177=ORIENTED_EDGE('',*,*,#20547,.T.);
#29178=ORIENTED_EDGE('',*,*,#20548,.F.);
#29179=ORIENTED_EDGE('',*,*,#20547,.F.);
#29180=ORIENTED_EDGE('',*,*,#20546,.T.);
#29181=ORIENTED_EDGE('',*,*,#20549,.T.);
#29182=ORIENTED_EDGE('',*,*,#20550,.T.);
#29183=ORIENTED_EDGE('',*,*,#20551,.T.);
#29184=ORIENTED_EDGE('',*,*,#20552,.T.);
#29185=ORIENTED_EDGE('',*,*,#20553,.F.);
#29186=ORIENTED_EDGE('',*,*,#20554,.F.);
#29187=ORIENTED_EDGE('',*,*,#20555,.T.);
#29188=ORIENTED_EDGE('',*,*,#20556,.T.);
#29189=ORIENTED_EDGE('',*,*,#20557,.T.);
#29190=ORIENTED_EDGE('',*,*,#20554,.T.);
#29191=ORIENTED_EDGE('',*,*,#20558,.F.);
#29192=ORIENTED_EDGE('',*,*,#20559,.F.);
#29193=ORIENTED_EDGE('',*,*,#20560,.T.);
#29194=ORIENTED_EDGE('',*,*,#20561,.T.);
#29195=ORIENTED_EDGE('',*,*,#20562,.T.);
#29196=ORIENTED_EDGE('',*,*,#20559,.T.);
#29197=ORIENTED_EDGE('',*,*,#20563,.F.);
#29198=ORIENTED_EDGE('',*,*,#20564,.F.);
#29199=ORIENTED_EDGE('',*,*,#20565,.T.);
#29200=ORIENTED_EDGE('',*,*,#20566,.T.);
#29201=ORIENTED_EDGE('',*,*,#20567,.T.);
#29202=ORIENTED_EDGE('',*,*,#20564,.T.);
#29203=ORIENTED_EDGE('',*,*,#20568,.F.);
#29204=ORIENTED_EDGE('',*,*,#20569,.F.);
#29205=ORIENTED_EDGE('',*,*,#20565,.F.);
#29206=ORIENTED_EDGE('',*,*,#20570,.F.);
#29207=ORIENTED_EDGE('',*,*,#20571,.T.);
#29208=ORIENTED_EDGE('',*,*,#20567,.F.);
#29209=ORIENTED_EDGE('',*,*,#20572,.T.);
#29210=ORIENTED_EDGE('',*,*,#20560,.F.);
#29211=ORIENTED_EDGE('',*,*,#20573,.F.);
#29212=ORIENTED_EDGE('',*,*,#20574,.F.);
#29213=ORIENTED_EDGE('',*,*,#20575,.T.);
#29214=ORIENTED_EDGE('',*,*,#20576,.F.);
#29215=ORIENTED_EDGE('',*,*,#20551,.F.);
#29216=ORIENTED_EDGE('',*,*,#20577,.T.);
#29217=ORIENTED_EDGE('',*,*,#20557,.F.);
#29218=ORIENTED_EDGE('',*,*,#20578,.T.);
#29219=ORIENTED_EDGE('',*,*,#20549,.F.);
#29220=ORIENTED_EDGE('',*,*,#20576,.T.);
#29221=ORIENTED_EDGE('',*,*,#20579,.T.);
#29222=ORIENTED_EDGE('',*,*,#20574,.T.);
#29223=ORIENTED_EDGE('',*,*,#20580,.T.);
#29224=ORIENTED_EDGE('',*,*,#20581,.F.);
#29225=ORIENTED_EDGE('',*,*,#20552,.F.);
#29226=ORIENTED_EDGE('',*,*,#20573,.T.);
#29227=ORIENTED_EDGE('',*,*,#20582,.T.);
#29228=ORIENTED_EDGE('',*,*,#20570,.T.);
#29229=ORIENTED_EDGE('',*,*,#20569,.T.);
#29230=ORIENTED_EDGE('',*,*,#20583,.F.);
#29231=ORIENTED_EDGE('',*,*,#20580,.F.);
#29232=ORIENTED_EDGE('',*,*,#20555,.F.);
#29233=ORIENTED_EDGE('',*,*,#20562,.F.);
#29234=ORIENTED_EDGE('',*,*,#20584,.T.);
#29235=ORIENTED_EDGE('',*,*,#20572,.F.);
#29236=ORIENTED_EDGE('',*,*,#20566,.F.);
#29237=ORIENTED_EDGE('',*,*,#20571,.F.);
#29238=ORIENTED_EDGE('',*,*,#20582,.F.);
#29239=ORIENTED_EDGE('',*,*,#20575,.F.);
#29240=ORIENTED_EDGE('',*,*,#20579,.F.);
#29241=ORIENTED_EDGE('',*,*,#20577,.F.);
#29242=ORIENTED_EDGE('',*,*,#20550,.F.);
#29243=ORIENTED_EDGE('',*,*,#20578,.F.);
#29244=ORIENTED_EDGE('',*,*,#20556,.F.);
#29245=ORIENTED_EDGE('',*,*,#20584,.F.);
#29246=ORIENTED_EDGE('',*,*,#20561,.F.);
#29247=ORIENTED_EDGE('',*,*,#20585,.T.);
#29248=ORIENTED_EDGE('',*,*,#20586,.T.);
#29249=ORIENTED_EDGE('',*,*,#20587,.T.);
#29250=ORIENTED_EDGE('',*,*,#20588,.T.);
#29251=ORIENTED_EDGE('',*,*,#20589,.F.);
#29252=ORIENTED_EDGE('',*,*,#20590,.F.);
#29253=ORIENTED_EDGE('',*,*,#20591,.T.);
#29254=ORIENTED_EDGE('',*,*,#20592,.T.);
#29255=ORIENTED_EDGE('',*,*,#20593,.T.);
#29256=ORIENTED_EDGE('',*,*,#20590,.T.);
#29257=ORIENTED_EDGE('',*,*,#20594,.F.);
#29258=ORIENTED_EDGE('',*,*,#20595,.F.);
#29259=ORIENTED_EDGE('',*,*,#20596,.T.);
#29260=ORIENTED_EDGE('',*,*,#20597,.T.);
#29261=ORIENTED_EDGE('',*,*,#20598,.T.);
#29262=ORIENTED_EDGE('',*,*,#20595,.T.);
#29263=ORIENTED_EDGE('',*,*,#20599,.F.);
#29264=ORIENTED_EDGE('',*,*,#20600,.F.);
#29265=ORIENTED_EDGE('',*,*,#20601,.T.);
#29266=ORIENTED_EDGE('',*,*,#20602,.T.);
#29267=ORIENTED_EDGE('',*,*,#20603,.T.);
#29268=ORIENTED_EDGE('',*,*,#20600,.T.);
#29269=ORIENTED_EDGE('',*,*,#20604,.F.);
#29270=ORIENTED_EDGE('',*,*,#20605,.F.);
#29271=ORIENTED_EDGE('',*,*,#20601,.F.);
#29272=ORIENTED_EDGE('',*,*,#20606,.F.);
#29273=ORIENTED_EDGE('',*,*,#20607,.T.);
#29274=ORIENTED_EDGE('',*,*,#20603,.F.);
#29275=ORIENTED_EDGE('',*,*,#20608,.T.);
#29276=ORIENTED_EDGE('',*,*,#20596,.F.);
#29277=ORIENTED_EDGE('',*,*,#20609,.F.);
#29278=ORIENTED_EDGE('',*,*,#20610,.F.);
#29279=ORIENTED_EDGE('',*,*,#20611,.T.);
#29280=ORIENTED_EDGE('',*,*,#20612,.F.);
#29281=ORIENTED_EDGE('',*,*,#20587,.F.);
#29282=ORIENTED_EDGE('',*,*,#20613,.T.);
#29283=ORIENTED_EDGE('',*,*,#20593,.F.);
#29284=ORIENTED_EDGE('',*,*,#20614,.T.);
#29285=ORIENTED_EDGE('',*,*,#20585,.F.);
#29286=ORIENTED_EDGE('',*,*,#20612,.T.);
#29287=ORIENTED_EDGE('',*,*,#20615,.T.);
#29288=ORIENTED_EDGE('',*,*,#20610,.T.);
#29289=ORIENTED_EDGE('',*,*,#20616,.T.);
#29290=ORIENTED_EDGE('',*,*,#20617,.F.);
#29291=ORIENTED_EDGE('',*,*,#20588,.F.);
#29292=ORIENTED_EDGE('',*,*,#20609,.T.);
#29293=ORIENTED_EDGE('',*,*,#20618,.T.);
#29294=ORIENTED_EDGE('',*,*,#20606,.T.);
#29295=ORIENTED_EDGE('',*,*,#20605,.T.);
#29296=ORIENTED_EDGE('',*,*,#20619,.F.);
#29297=ORIENTED_EDGE('',*,*,#20616,.F.);
#29298=ORIENTED_EDGE('',*,*,#20591,.F.);
#29299=ORIENTED_EDGE('',*,*,#20598,.F.);
#29300=ORIENTED_EDGE('',*,*,#20620,.T.);
#29301=ORIENTED_EDGE('',*,*,#20608,.F.);
#29302=ORIENTED_EDGE('',*,*,#20602,.F.);
#29303=ORIENTED_EDGE('',*,*,#20607,.F.);
#29304=ORIENTED_EDGE('',*,*,#20618,.F.);
#29305=ORIENTED_EDGE('',*,*,#20611,.F.);
#29306=ORIENTED_EDGE('',*,*,#20615,.F.);
#29307=ORIENTED_EDGE('',*,*,#20613,.F.);
#29308=ORIENTED_EDGE('',*,*,#20586,.F.);
#29309=ORIENTED_EDGE('',*,*,#20614,.F.);
#29310=ORIENTED_EDGE('',*,*,#20592,.F.);
#29311=ORIENTED_EDGE('',*,*,#20620,.F.);
#29312=ORIENTED_EDGE('',*,*,#20597,.F.);
#29313=ORIENTED_EDGE('',*,*,#20385,.F.);
#29314=ORIENTED_EDGE('',*,*,#20402,.F.);
#29315=ORIENTED_EDGE('',*,*,#20621,.F.);
#29316=ORIENTED_EDGE('',*,*,#20622,.T.);
#29317=ORIENTED_EDGE('',*,*,#20467,.T.);
#29318=ORIENTED_EDGE('',*,*,#20623,.F.);
#29319=ORIENTED_EDGE('',*,*,#20368,.T.);
#29320=ORIENTED_EDGE('',*,*,#20624,.T.);
#29321=ORIENTED_EDGE('',*,*,#20625,.T.);
#29322=ORIENTED_EDGE('',*,*,#20624,.F.);
#29323=ORIENTED_EDGE('',*,*,#20367,.T.);
#29324=ORIENTED_EDGE('',*,*,#20626,.T.);
#29325=ORIENTED_EDGE('',*,*,#20627,.T.);
#29326=ORIENTED_EDGE('',*,*,#20626,.F.);
#29327=ORIENTED_EDGE('',*,*,#20366,.T.);
#29328=ORIENTED_EDGE('',*,*,#20628,.T.);
#29329=ORIENTED_EDGE('',*,*,#20629,.T.);
#29330=ORIENTED_EDGE('',*,*,#20628,.F.);
#29331=ORIENTED_EDGE('',*,*,#20365,.T.);
#29332=ORIENTED_EDGE('',*,*,#20630,.T.);
#29333=ORIENTED_EDGE('',*,*,#20631,.T.);
#29334=ORIENTED_EDGE('',*,*,#20630,.F.);
#29335=ORIENTED_EDGE('',*,*,#20364,.T.);
#29336=ORIENTED_EDGE('',*,*,#20632,.T.);
#29337=ORIENTED_EDGE('',*,*,#20633,.T.);
#29338=ORIENTED_EDGE('',*,*,#20632,.F.);
#29339=ORIENTED_EDGE('',*,*,#20363,.T.);
#29340=ORIENTED_EDGE('',*,*,#20395,.T.);
#29341=ORIENTED_EDGE('',*,*,#20634,.T.);
#29342=ORIENTED_EDGE('',*,*,#20411,.T.);
#29343=ORIENTED_EDGE('',*,*,#20635,.F.);
#29344=ORIENTED_EDGE('',*,*,#20465,.F.);
#29345=ORIENTED_EDGE('',*,*,#20636,.F.);
#29346=ORIENTED_EDGE('',*,*,#20413,.T.);
#29347=ORIENTED_EDGE('',*,*,#20637,.F.);
#29348=ORIENTED_EDGE('',*,*,#20372,.T.);
#29349=ORIENTED_EDGE('',*,*,#20638,.F.);
#29350=ORIENTED_EDGE('',*,*,#20414,.T.);
#29351=ORIENTED_EDGE('',*,*,#20638,.T.);
#29352=ORIENTED_EDGE('',*,*,#20371,.T.);
#29353=ORIENTED_EDGE('',*,*,#20390,.T.);
#29354=ORIENTED_EDGE('',*,*,#20639,.T.);
#29355=ORIENTED_EDGE('',*,*,#20461,.T.);
#29356=ORIENTED_EDGE('',*,*,#20640,.T.);
#29357=ORIENTED_EDGE('',*,*,#20460,.T.);
#29358=ORIENTED_EDGE('',*,*,#20641,.T.);
#29359=ORIENTED_EDGE('',*,*,#20642,.T.);
#29360=ORIENTED_EDGE('',*,*,#20643,.T.);
#29361=ORIENTED_EDGE('',*,*,#20644,.T.);
#29362=ORIENTED_EDGE('',*,*,#20645,.T.);
#29363=ORIENTED_EDGE('',*,*,#20646,.T.);
#29364=ORIENTED_EDGE('',*,*,#20647,.T.);
#29365=ORIENTED_EDGE('',*,*,#20648,.F.);
#29366=ORIENTED_EDGE('',*,*,#20646,.F.);
#29367=ORIENTED_EDGE('',*,*,#20649,.T.);
#29368=ORIENTED_EDGE('',*,*,#20650,.T.);
#29369=ORIENTED_EDGE('',*,*,#20649,.F.);
#29370=ORIENTED_EDGE('',*,*,#20645,.F.);
#29371=ORIENTED_EDGE('',*,*,#20651,.T.);
#29372=ORIENTED_EDGE('',*,*,#20652,.T.);
#29373=ORIENTED_EDGE('',*,*,#20653,.F.);
#29374=ORIENTED_EDGE('',*,*,#20651,.F.);
#29375=ORIENTED_EDGE('',*,*,#20644,.F.);
#29376=ORIENTED_EDGE('',*,*,#20654,.T.);
#29377=ORIENTED_EDGE('',*,*,#20652,.F.);
#29378=ORIENTED_EDGE('',*,*,#20643,.F.);
#29379=ORIENTED_EDGE('',*,*,#20655,.T.);
#29380=ORIENTED_EDGE('',*,*,#20656,.T.);
#29381=ORIENTED_EDGE('',*,*,#20655,.F.);
#29382=ORIENTED_EDGE('',*,*,#20642,.F.);
#29383=ORIENTED_EDGE('',*,*,#20657,.T.);
#29384=ORIENTED_EDGE('',*,*,#20658,.T.);
#29385=ORIENTED_EDGE('',*,*,#20657,.F.);
#29386=ORIENTED_EDGE('',*,*,#20641,.F.);
#29387=ORIENTED_EDGE('',*,*,#20648,.T.);
#29388=ORIENTED_EDGE('',*,*,#20659,.T.);
#29389=ORIENTED_EDGE('',*,*,#20438,.T.);
#29390=ORIENTED_EDGE('',*,*,#20639,.F.);
#29391=ORIENTED_EDGE('',*,*,#20659,.F.);
#29392=ORIENTED_EDGE('',*,*,#20654,.F.);
#29393=ORIENTED_EDGE('',*,*,#20656,.F.);
#29394=ORIENTED_EDGE('',*,*,#20658,.F.);
#29395=ORIENTED_EDGE('',*,*,#20647,.F.);
#29396=ORIENTED_EDGE('',*,*,#20650,.F.);
#29397=ORIENTED_EDGE('',*,*,#20653,.T.);
#29398=ORIENTED_EDGE('',*,*,#20660,.T.);
#29399=ORIENTED_EDGE('',*,*,#20661,.T.);
#29400=ORIENTED_EDGE('',*,*,#20662,.T.);
#29401=ORIENTED_EDGE('',*,*,#20663,.T.);
#29402=ORIENTED_EDGE('',*,*,#20664,.T.);
#29403=ORIENTED_EDGE('',*,*,#20665,.T.);
#29404=ORIENTED_EDGE('',*,*,#20666,.T.);
#29405=ORIENTED_EDGE('',*,*,#20667,.F.);
#29406=ORIENTED_EDGE('',*,*,#20665,.F.);
#29407=ORIENTED_EDGE('',*,*,#20668,.T.);
#29408=ORIENTED_EDGE('',*,*,#20669,.T.);
#29409=ORIENTED_EDGE('',*,*,#20668,.F.);
#29410=ORIENTED_EDGE('',*,*,#20664,.F.);
#29411=ORIENTED_EDGE('',*,*,#20670,.T.);
#29412=ORIENTED_EDGE('',*,*,#20671,.T.);
#29413=ORIENTED_EDGE('',*,*,#20672,.F.);
#29414=ORIENTED_EDGE('',*,*,#20670,.F.);
#29415=ORIENTED_EDGE('',*,*,#20663,.F.);
#29416=ORIENTED_EDGE('',*,*,#20673,.T.);
#29417=ORIENTED_EDGE('',*,*,#20671,.F.);
#29418=ORIENTED_EDGE('',*,*,#20662,.F.);
#29419=ORIENTED_EDGE('',*,*,#20674,.T.);
#29420=ORIENTED_EDGE('',*,*,#20675,.T.);
#29421=ORIENTED_EDGE('',*,*,#20674,.F.);
#29422=ORIENTED_EDGE('',*,*,#20661,.F.);
#29423=ORIENTED_EDGE('',*,*,#20676,.T.);
#29424=ORIENTED_EDGE('',*,*,#20677,.T.);
#29425=ORIENTED_EDGE('',*,*,#20676,.F.);
#29426=ORIENTED_EDGE('',*,*,#20660,.F.);
#29427=ORIENTED_EDGE('',*,*,#20667,.T.);
#29428=ORIENTED_EDGE('',*,*,#20678,.T.);
#29429=ORIENTED_EDGE('',*,*,#20440,.T.);
#29430=ORIENTED_EDGE('',*,*,#20640,.F.);
#29431=ORIENTED_EDGE('',*,*,#20678,.F.);
#29432=ORIENTED_EDGE('',*,*,#20673,.F.);
#29433=ORIENTED_EDGE('',*,*,#20675,.F.);
#29434=ORIENTED_EDGE('',*,*,#20677,.F.);
#29435=ORIENTED_EDGE('',*,*,#20666,.F.);
#29436=ORIENTED_EDGE('',*,*,#20669,.F.);
#29437=ORIENTED_EDGE('',*,*,#20672,.T.);
#29438=ORIENTED_EDGE('',*,*,#20541,.F.);
#29439=ORIENTED_EDGE('',*,*,#20679,.T.);
#29440=ORIENTED_EDGE('',*,*,#20680,.T.);
#29441=ORIENTED_EDGE('',*,*,#20503,.F.);
#29442=ORIENTED_EDGE('',*,*,#20540,.F.);
#29443=ORIENTED_EDGE('',*,*,#20681,.T.);
#29444=ORIENTED_EDGE('',*,*,#20682,.F.);
#29445=ORIENTED_EDGE('',*,*,#20679,.F.);
#29446=ORIENTED_EDGE('',*,*,#20539,.F.);
#29447=ORIENTED_EDGE('',*,*,#20498,.T.);
#29448=ORIENTED_EDGE('',*,*,#20683,.T.);
#29449=ORIENTED_EDGE('',*,*,#20681,.F.);
#29450=ORIENTED_EDGE('',*,*,#20684,.T.);
#29451=ORIENTED_EDGE('',*,*,#20682,.T.);
#29452=ORIENTED_EDGE('',*,*,#20683,.F.);
#29453=ORIENTED_EDGE('',*,*,#20497,.F.);
#29454=ORIENTED_EDGE('',*,*,#20501,.F.);
#29455=ORIENTED_EDGE('',*,*,#20504,.F.);
#29456=ORIENTED_EDGE('',*,*,#20680,.F.);
#29457=ORIENTED_EDGE('',*,*,#20538,.T.);
#29458=ORIENTED_EDGE('',*,*,#20685,.T.);
#29459=ORIENTED_EDGE('',*,*,#20684,.F.);
#29460=ORIENTED_EDGE('',*,*,#20685,.F.);
#29461=ORIENTED_EDGE('',*,*,#20537,.T.);
#29462=ORIENTED_EDGE('',*,*,#20463,.T.);
#29463=ORIENTED_EDGE('',*,*,#20686,.T.);
#29464=ORIENTED_EDGE('',*,*,#20687,.F.);
#29465=ORIENTED_EDGE('',*,*,#20688,.F.);
#29466=ORIENTED_EDGE('',*,*,#20686,.F.);
#29467=ORIENTED_EDGE('',*,*,#20688,.T.);
#29468=ORIENTED_EDGE('',*,*,#20689,.T.);
#29469=ORIENTED_EDGE('',*,*,#20690,.F.);
#29470=ORIENTED_EDGE('',*,*,#20691,.F.);
#29471=ORIENTED_EDGE('',*,*,#20689,.F.);
#29472=ORIENTED_EDGE('',*,*,#20687,.T.);
#29473=ORIENTED_EDGE('',*,*,#20691,.T.);
#29474=ORIENTED_EDGE('',*,*,#20692,.T.);
#29475=ORIENTED_EDGE('',*,*,#20693,.F.);
#29476=ORIENTED_EDGE('',*,*,#20692,.F.);
#29477=ORIENTED_EDGE('',*,*,#20690,.T.);
#29478=ORIENTED_EDGE('',*,*,#20694,.T.);
#29479=ORIENTED_EDGE('',*,*,#20695,.F.);
#29480=ORIENTED_EDGE('',*,*,#20696,.F.);
#29481=ORIENTED_EDGE('',*,*,#20694,.F.);
#29482=ORIENTED_EDGE('',*,*,#20696,.T.);
#29483=ORIENTED_EDGE('',*,*,#20697,.T.);
#29484=ORIENTED_EDGE('',*,*,#20698,.F.);
#29485=ORIENTED_EDGE('',*,*,#20699,.F.);
#29486=ORIENTED_EDGE('',*,*,#20697,.F.);
#29487=ORIENTED_EDGE('',*,*,#20695,.T.);
#29488=ORIENTED_EDGE('',*,*,#20699,.T.);
#29489=ORIENTED_EDGE('',*,*,#20700,.T.);
#29490=ORIENTED_EDGE('',*,*,#20701,.F.);
#29491=ORIENTED_EDGE('',*,*,#20700,.F.);
#29492=ORIENTED_EDGE('',*,*,#20698,.T.);
#29493=ORIENTED_EDGE('',*,*,#20702,.T.);
#29494=ORIENTED_EDGE('',*,*,#20703,.F.);
#29495=ORIENTED_EDGE('',*,*,#20704,.F.);
#29496=ORIENTED_EDGE('',*,*,#20702,.F.);
#29497=ORIENTED_EDGE('',*,*,#20704,.T.);
#29498=ORIENTED_EDGE('',*,*,#20705,.T.);
#29499=ORIENTED_EDGE('',*,*,#20706,.F.);
#29500=ORIENTED_EDGE('',*,*,#20707,.F.);
#29501=ORIENTED_EDGE('',*,*,#20705,.F.);
#29502=ORIENTED_EDGE('',*,*,#20703,.T.);
#29503=ORIENTED_EDGE('',*,*,#20707,.T.);
#29504=ORIENTED_EDGE('',*,*,#20708,.T.);
#29505=ORIENTED_EDGE('',*,*,#20709,.F.);
#29506=ORIENTED_EDGE('',*,*,#20708,.F.);
#29507=ORIENTED_EDGE('',*,*,#20706,.T.);
#29508=ORIENTED_EDGE('',*,*,#20710,.F.);
#29509=ORIENTED_EDGE('',*,*,#20711,.F.);
#29510=ORIENTED_EDGE('',*,*,#20712,.T.);
#29511=ORIENTED_EDGE('',*,*,#20713,.T.);
#29512=ORIENTED_EDGE('',*,*,#20712,.F.);
#29513=ORIENTED_EDGE('',*,*,#20710,.T.);
#29514=ORIENTED_EDGE('',*,*,#20711,.T.);
#29515=ORIENTED_EDGE('',*,*,#20714,.T.);
#29516=ORIENTED_EDGE('',*,*,#20715,.F.);
#29517=ORIENTED_EDGE('',*,*,#20716,.F.);
#29518=ORIENTED_EDGE('',*,*,#20714,.F.);
#29519=ORIENTED_EDGE('',*,*,#20717,.T.);
#29520=ORIENTED_EDGE('',*,*,#20715,.T.);
#29521=ORIENTED_EDGE('',*,*,#20716,.T.);
#29522=ORIENTED_EDGE('',*,*,#20717,.F.);
#29523=ORIENTED_EDGE('',*,*,#20718,.F.);
#29524=ORIENTED_EDGE('',*,*,#20719,.F.);
#29525=ORIENTED_EDGE('',*,*,#20720,.T.);
#29526=ORIENTED_EDGE('',*,*,#20721,.T.);
#29527=ORIENTED_EDGE('',*,*,#20720,.F.);
#29528=ORIENTED_EDGE('',*,*,#20718,.T.);
#29529=ORIENTED_EDGE('',*,*,#20719,.T.);
#29530=ORIENTED_EDGE('',*,*,#20722,.T.);
#29531=ORIENTED_EDGE('',*,*,#20723,.F.);
#29532=ORIENTED_EDGE('',*,*,#20724,.F.);
#29533=ORIENTED_EDGE('',*,*,#20722,.F.);
#29534=ORIENTED_EDGE('',*,*,#20725,.T.);
#29535=ORIENTED_EDGE('',*,*,#20723,.T.);
#29536=ORIENTED_EDGE('',*,*,#20724,.T.);
#29537=ORIENTED_EDGE('',*,*,#20725,.F.);
#29538=ORIENTED_EDGE('',*,*,#20726,.F.);
#29539=ORIENTED_EDGE('',*,*,#20727,.F.);
#29540=ORIENTED_EDGE('',*,*,#20728,.T.);
#29541=ORIENTED_EDGE('',*,*,#20729,.T.);
#29542=ORIENTED_EDGE('',*,*,#20728,.F.);
#29543=ORIENTED_EDGE('',*,*,#20726,.T.);
#29544=ORIENTED_EDGE('',*,*,#20727,.T.);
#29545=ORIENTED_EDGE('',*,*,#20730,.T.);
#29546=ORIENTED_EDGE('',*,*,#20731,.F.);
#29547=ORIENTED_EDGE('',*,*,#20732,.F.);
#29548=ORIENTED_EDGE('',*,*,#20730,.F.);
#29549=ORIENTED_EDGE('',*,*,#20733,.T.);
#29550=ORIENTED_EDGE('',*,*,#20731,.T.);
#29551=ORIENTED_EDGE('',*,*,#20732,.T.);
#29552=ORIENTED_EDGE('',*,*,#20733,.F.);
#29553=ORIENTED_EDGE('',*,*,#20734,.F.);
#29554=ORIENTED_EDGE('',*,*,#20735,.F.);
#29555=ORIENTED_EDGE('',*,*,#20736,.T.);
#29556=ORIENTED_EDGE('',*,*,#20737,.T.);
#29557=ORIENTED_EDGE('',*,*,#20736,.F.);
#29558=ORIENTED_EDGE('',*,*,#20734,.T.);
#29559=ORIENTED_EDGE('',*,*,#20735,.T.);
#29560=ORIENTED_EDGE('',*,*,#20738,.T.);
#29561=ORIENTED_EDGE('',*,*,#20739,.F.);
#29562=ORIENTED_EDGE('',*,*,#20740,.F.);
#29563=ORIENTED_EDGE('',*,*,#20738,.F.);
#29564=ORIENTED_EDGE('',*,*,#20741,.T.);
#29565=ORIENTED_EDGE('',*,*,#20739,.T.);
#29566=ORIENTED_EDGE('',*,*,#20740,.T.);
#29567=ORIENTED_EDGE('',*,*,#20741,.F.);
#29568=ORIENTED_EDGE('',*,*,#20742,.T.);
#29569=ORIENTED_EDGE('',*,*,#20454,.T.);
#29570=ORIENTED_EDGE('',*,*,#20455,.T.);
#29571=ORIENTED_EDGE('',*,*,#20742,.F.);
#29572=ORIENTED_EDGE('',*,*,#20743,.T.);
#29573=ORIENTED_EDGE('',*,*,#20418,.T.);
#29574=ORIENTED_EDGE('',*,*,#20419,.T.);
#29575=ORIENTED_EDGE('',*,*,#20743,.F.);
#29576=ORIENTED_EDGE('',*,*,#20744,.T.);
#29577=ORIENTED_EDGE('',*,*,#20511,.F.);
#29578=ORIENTED_EDGE('',*,*,#20512,.F.);
#29579=ORIENTED_EDGE('',*,*,#20744,.F.);
#29580=ORIENTED_EDGE('',*,*,#20745,.T.);
#29581=ORIENTED_EDGE('',*,*,#20515,.F.);
#29582=ORIENTED_EDGE('',*,*,#20516,.F.);
#29583=ORIENTED_EDGE('',*,*,#20745,.F.);
#29584=ORIENTED_EDGE('',*,*,#20746,.T.);
#29585=ORIENTED_EDGE('',*,*,#20519,.F.);
#29586=ORIENTED_EDGE('',*,*,#20520,.F.);
#29587=ORIENTED_EDGE('',*,*,#20746,.F.);
#29588=ORIENTED_EDGE('',*,*,#20747,.T.);
#29589=ORIENTED_EDGE('',*,*,#20523,.F.);
#29590=ORIENTED_EDGE('',*,*,#20524,.F.);
#29591=ORIENTED_EDGE('',*,*,#20747,.F.);
#29592=ORIENTED_EDGE('',*,*,#20748,.T.);
#29593=ORIENTED_EDGE('',*,*,#20432,.T.);
#29594=ORIENTED_EDGE('',*,*,#20433,.T.);
#29595=ORIENTED_EDGE('',*,*,#20748,.F.);
#29596=ORIENTED_EDGE('',*,*,#20749,.T.);
#29597=ORIENTED_EDGE('',*,*,#20447,.T.);
#29598=ORIENTED_EDGE('',*,*,#20448,.T.);
#29599=ORIENTED_EDGE('',*,*,#20749,.F.);
#29600=ORIENTED_EDGE('',*,*,#20750,.T.);
#29601=ORIENTED_EDGE('',*,*,#20443,.T.);
#29602=ORIENTED_EDGE('',*,*,#20751,.F.);
#29603=ORIENTED_EDGE('',*,*,#20752,.F.);
#29604=ORIENTED_EDGE('',*,*,#20751,.T.);
#29605=ORIENTED_EDGE('',*,*,#20442,.T.);
#29606=ORIENTED_EDGE('',*,*,#20753,.F.);
#29607=ORIENTED_EDGE('',*,*,#20754,.F.);
#29608=ORIENTED_EDGE('',*,*,#20755,.T.);
#29609=ORIENTED_EDGE('',*,*,#20535,.T.);
#29610=ORIENTED_EDGE('',*,*,#20756,.F.);
#29611=ORIENTED_EDGE('',*,*,#20757,.F.);
#29612=ORIENTED_EDGE('',*,*,#20753,.T.);
#29613=ORIENTED_EDGE('',*,*,#20459,.T.);
#29614=ORIENTED_EDGE('',*,*,#20758,.F.);
#29615=ORIENTED_EDGE('',*,*,#20759,.F.);
#29616=ORIENTED_EDGE('',*,*,#20758,.T.);
#29617=ORIENTED_EDGE('',*,*,#20458,.T.);
#29618=ORIENTED_EDGE('',*,*,#20760,.F.);
#29619=ORIENTED_EDGE('',*,*,#20761,.F.);
#29620=ORIENTED_EDGE('',*,*,#20760,.T.);
#29621=ORIENTED_EDGE('',*,*,#20457,.T.);
#29622=ORIENTED_EDGE('',*,*,#20530,.T.);
#29623=ORIENTED_EDGE('',*,*,#20762,.F.);
#29624=ORIENTED_EDGE('',*,*,#20763,.F.);
#29625=ORIENTED_EDGE('',*,*,#20762,.T.);
#29626=ORIENTED_EDGE('',*,*,#20529,.T.);
#29627=ORIENTED_EDGE('',*,*,#20764,.F.);
#29628=ORIENTED_EDGE('',*,*,#20765,.F.);
#29629=ORIENTED_EDGE('',*,*,#20764,.T.);
#29630=ORIENTED_EDGE('',*,*,#20528,.T.);
#29631=ORIENTED_EDGE('',*,*,#20755,.F.);
#29632=ORIENTED_EDGE('',*,*,#20766,.F.);
#29633=ORIENTED_EDGE('',*,*,#20767,.T.);
#29634=ORIENTED_EDGE('',*,*,#20768,.T.);
#29635=ORIENTED_EDGE('',*,*,#20752,.T.);
#29636=ORIENTED_EDGE('',*,*,#20754,.T.);
#29637=ORIENTED_EDGE('',*,*,#20759,.T.);
#29638=ORIENTED_EDGE('',*,*,#20761,.T.);
#29639=ORIENTED_EDGE('',*,*,#20763,.T.);
#29640=ORIENTED_EDGE('',*,*,#20765,.T.);
#29641=ORIENTED_EDGE('',*,*,#20766,.T.);
#29642=ORIENTED_EDGE('',*,*,#20757,.T.);
#29643=ORIENTED_EDGE('',*,*,#20769,.T.);
#29644=ORIENTED_EDGE('',*,*,#20770,.T.);
#29645=ORIENTED_EDGE('',*,*,#20771,.T.);
#29646=ORIENTED_EDGE('',*,*,#20772,.T.);
#29647=ORIENTED_EDGE('',*,*,#20773,.T.);
#29648=ORIENTED_EDGE('',*,*,#20774,.T.);
#29649=ORIENTED_EDGE('',*,*,#20775,.T.);
#29650=ORIENTED_EDGE('',*,*,#20776,.T.);
#29651=ORIENTED_EDGE('',*,*,#20777,.T.);
#29652=ORIENTED_EDGE('',*,*,#20778,.F.);
#29653=ORIENTED_EDGE('',*,*,#20778,.T.);
#29654=ORIENTED_EDGE('',*,*,#20779,.T.);
#29655=ORIENTED_EDGE('',*,*,#20780,.T.);
#29656=ORIENTED_EDGE('',*,*,#20779,.F.);
#29657=ORIENTED_EDGE('',*,*,#20781,.T.);
#29658=ORIENTED_EDGE('',*,*,#20782,.T.);
#29659=ORIENTED_EDGE('',*,*,#20783,.F.);
#29660=ORIENTED_EDGE('',*,*,#20782,.F.);
#29661=ORIENTED_EDGE('',*,*,#20784,.T.);
#29662=ORIENTED_EDGE('',*,*,#20483,.T.);
#29663=ORIENTED_EDGE('',*,*,#20531,.T.);
#29664=ORIENTED_EDGE('',*,*,#20456,.T.);
#29665=ORIENTED_EDGE('',*,*,#20451,.T.);
#29666=ORIENTED_EDGE('',*,*,#20357,.T.);
#29667=ORIENTED_EDGE('',*,*,#20637,.T.);
#29668=ORIENTED_EDGE('',*,*,#20412,.T.);
#29669=ORIENTED_EDGE('',*,*,#20636,.T.);
#29670=ORIENTED_EDGE('',*,*,#20464,.T.);
#29671=ORIENTED_EDGE('',*,*,#20536,.T.);
#29672=ORIENTED_EDGE('',*,*,#20462,.T.);
#29673=ORIENTED_EDGE('',*,*,#20449,.T.);
#29674=ORIENTED_EDGE('',*,*,#20445,.T.);
#29675=ORIENTED_EDGE('',*,*,#20532,.T.);
#29676=ORIENTED_EDGE('',*,*,#20480,.T.);
#29677=ORIENTED_EDGE('',*,*,#20505,.T.);
#29678=ORIENTED_EDGE('',*,*,#20514,.T.);
#29679=ORIENTED_EDGE('',*,*,#20518,.T.);
#29680=ORIENTED_EDGE('',*,*,#20522,.T.);
#29681=ORIENTED_EDGE('',*,*,#20526,.T.);
#29682=ORIENTED_EDGE('',*,*,#20391,.F.);
#29683=ORIENTED_EDGE('',*,*,#20369,.T.);
#29684=ORIENTED_EDGE('',*,*,#20623,.T.);
#29685=ORIENTED_EDGE('',*,*,#20785,.T.);
#29686=ORIENTED_EDGE('',*,*,#20393,.F.);
#29687=ORIENTED_EDGE('',*,*,#20400,.T.);
#29688=ORIENTED_EDGE('',*,*,#20473,.T.);
#29689=ORIENTED_EDGE('',*,*,#20786,.F.);
#29690=ORIENTED_EDGE('',*,*,#20787,.F.);
#29691=ORIENTED_EDGE('',*,*,#20786,.T.);
#29692=ORIENTED_EDGE('',*,*,#20472,.T.);
#29693=ORIENTED_EDGE('',*,*,#20788,.F.);
#29694=ORIENTED_EDGE('',*,*,#20789,.F.);
#29695=ORIENTED_EDGE('',*,*,#20788,.T.);
#29696=ORIENTED_EDGE('',*,*,#20471,.T.);
#29697=ORIENTED_EDGE('',*,*,#20790,.F.);
#29698=ORIENTED_EDGE('',*,*,#20791,.F.);
#29699=ORIENTED_EDGE('',*,*,#20790,.T.);
#29700=ORIENTED_EDGE('',*,*,#20470,.T.);
#29701=ORIENTED_EDGE('',*,*,#20792,.F.);
#29702=ORIENTED_EDGE('',*,*,#20793,.F.);
#29703=ORIENTED_EDGE('',*,*,#20792,.T.);
#29704=ORIENTED_EDGE('',*,*,#20469,.T.);
#29705=ORIENTED_EDGE('',*,*,#20794,.F.);
#29706=ORIENTED_EDGE('',*,*,#20795,.F.);
#29707=ORIENTED_EDGE('',*,*,#20794,.T.);
#29708=ORIENTED_EDGE('',*,*,#20468,.T.);
#29709=ORIENTED_EDGE('',*,*,#20622,.F.);
#29710=ORIENTED_EDGE('',*,*,#20796,.F.);
#29711=ORIENTED_EDGE('',*,*,#20621,.T.);
#29712=ORIENTED_EDGE('',*,*,#20401,.T.);
#29713=ORIENTED_EDGE('',*,*,#20787,.T.);
#29714=ORIENTED_EDGE('',*,*,#20789,.T.);
#29715=ORIENTED_EDGE('',*,*,#20791,.T.);
#29716=ORIENTED_EDGE('',*,*,#20793,.T.);
#29717=ORIENTED_EDGE('',*,*,#20795,.T.);
#29718=ORIENTED_EDGE('',*,*,#20796,.T.);
#29719=ORIENTED_EDGE('',*,*,#20713,.F.);
#29720=ORIENTED_EDGE('',*,*,#20721,.F.);
#29721=ORIENTED_EDGE('',*,*,#20729,.F.);
#29722=ORIENTED_EDGE('',*,*,#20737,.F.);
#29723=ORIENTED_EDGE('',*,*,#20783,.T.);
#29724=ORIENTED_EDGE('',*,*,#20797,.T.);
#29725=ORIENTED_EDGE('',*,*,#20533,.T.);
#29726=ORIENTED_EDGE('',*,*,#20444,.T.);
#29727=ORIENTED_EDGE('',*,*,#20750,.F.);
#29728=ORIENTED_EDGE('',*,*,#20768,.F.);
#29729=ORIENTED_EDGE('',*,*,#20756,.T.);
#29730=ORIENTED_EDGE('',*,*,#20534,.T.);
#29731=ORIENTED_EDGE('',*,*,#20797,.F.);
#29732=ORIENTED_EDGE('',*,*,#20767,.F.);
#29733=ORIENTED_EDGE('',*,*,#20410,.T.);
#29734=ORIENTED_EDGE('',*,*,#20387,.F.);
#29735=ORIENTED_EDGE('',*,*,#20466,.T.);
#29736=ORIENTED_EDGE('',*,*,#20635,.T.);
#29737=ORIENTED_EDGE('',*,*,#20798,.F.);
#29738=ORIENTED_EDGE('',*,*,#20799,.F.);
#29739=ORIENTED_EDGE('',*,*,#20800,.T.);
#29740=ORIENTED_EDGE('',*,*,#20801,.T.);
#29741=ORIENTED_EDGE('',*,*,#20800,.F.);
#29742=ORIENTED_EDGE('',*,*,#20415,.T.);
#29743=ORIENTED_EDGE('',*,*,#20802,.T.);
#29744=ORIENTED_EDGE('',*,*,#20803,.F.);
#29745=ORIENTED_EDGE('',*,*,#20804,.F.);
#29746=ORIENTED_EDGE('',*,*,#20805,.F.);
#29747=ORIENTED_EDGE('',*,*,#20802,.F.);
#29748=ORIENTED_EDGE('',*,*,#20478,.T.);
#29749=ORIENTED_EDGE('',*,*,#20806,.T.);
#29750=ORIENTED_EDGE('',*,*,#20807,.F.);
#29751=ORIENTED_EDGE('',*,*,#20806,.F.);
#29752=ORIENTED_EDGE('',*,*,#20477,.T.);
#29753=ORIENTED_EDGE('',*,*,#20798,.T.);
#29754=ORIENTED_EDGE('',*,*,#20799,.T.);
#29755=ORIENTED_EDGE('',*,*,#20808,.T.);
#29756=ORIENTED_EDGE('',*,*,#20804,.T.);
#29757=ORIENTED_EDGE('',*,*,#20809,.T.);
#29758=ORIENTED_EDGE('',*,*,#20777,.F.);
#29759=ORIENTED_EDGE('',*,*,#20809,.F.);
#29760=ORIENTED_EDGE('',*,*,#20803,.T.);
#29761=ORIENTED_EDGE('',*,*,#20805,.T.);
#29762=ORIENTED_EDGE('',*,*,#20808,.F.);
#29763=ORIENTED_EDGE('',*,*,#20405,.T.);
#29764=ORIENTED_EDGE('',*,*,#20378,.F.);
#29765=ORIENTED_EDGE('',*,*,#20396,.T.);
#29766=ORIENTED_EDGE('',*,*,#20361,.T.);
#29767=ORIENTED_EDGE('',*,*,#20420,.T.);
#29768=ORIENTED_EDGE('',*,*,#20409,.T.);
#29769=ORIENTED_EDGE('',*,*,#20435,.T.);
#29770=ORIENTED_EDGE('',*,*,#20474,.T.);
#29771=ORIENTED_EDGE('',*,*,#20398,.T.);
#29772=ORIENTED_EDGE('',*,*,#20404,.T.);
#29773=ORIENTED_EDGE('',*,*,#20810,.T.);
#29774=ORIENTED_EDGE('',*,*,#20811,.T.);
#29775=ORIENTED_EDGE('',*,*,#20812,.T.);
#29776=ORIENTED_EDGE('',*,*,#20811,.F.);
#29777=ORIENTED_EDGE('',*,*,#20813,.T.);
#29778=ORIENTED_EDGE('',*,*,#20814,.T.);
#29779=ORIENTED_EDGE('',*,*,#20815,.T.);
#29780=ORIENTED_EDGE('',*,*,#20816,.F.);
#29781=ORIENTED_EDGE('',*,*,#20815,.F.);
#29782=ORIENTED_EDGE('',*,*,#20785,.F.);
#29783=ORIENTED_EDGE('',*,*,#20625,.F.);
#29784=ORIENTED_EDGE('',*,*,#20627,.F.);
#29785=ORIENTED_EDGE('',*,*,#20629,.F.);
#29786=ORIENTED_EDGE('',*,*,#20631,.F.);
#29787=ORIENTED_EDGE('',*,*,#20633,.F.);
#29788=ORIENTED_EDGE('',*,*,#20634,.F.);
#29789=ORIENTED_EDGE('',*,*,#20394,.F.);
#29790=ORIENTED_EDGE('',*,*,#20553,.T.);
#29791=ORIENTED_EDGE('',*,*,#20581,.T.);
#29792=ORIENTED_EDGE('',*,*,#20583,.T.);
#29793=ORIENTED_EDGE('',*,*,#20568,.T.);
#29794=ORIENTED_EDGE('',*,*,#20563,.T.);
#29795=ORIENTED_EDGE('',*,*,#20558,.T.);
#29796=ORIENTED_EDGE('',*,*,#20817,.T.);
#29797=ORIENTED_EDGE('',*,*,#20818,.T.);
#29798=ORIENTED_EDGE('',*,*,#20819,.T.);
#29799=ORIENTED_EDGE('',*,*,#20820,.T.);
#29800=ORIENTED_EDGE('',*,*,#20821,.T.);
#29801=ORIENTED_EDGE('',*,*,#20822,.T.);
#29802=ORIENTED_EDGE('',*,*,#20589,.T.);
#29803=ORIENTED_EDGE('',*,*,#20617,.T.);
#29804=ORIENTED_EDGE('',*,*,#20619,.T.);
#29805=ORIENTED_EDGE('',*,*,#20604,.T.);
#29806=ORIENTED_EDGE('',*,*,#20599,.T.);
#29807=ORIENTED_EDGE('',*,*,#20594,.T.);
#29808=ORIENTED_EDGE('',*,*,#20823,.T.);
#29809=ORIENTED_EDGE('',*,*,#20824,.T.);
#29810=ORIENTED_EDGE('',*,*,#20825,.T.);
#29811=ORIENTED_EDGE('',*,*,#20826,.T.);
#29812=ORIENTED_EDGE('',*,*,#20827,.T.);
#29813=ORIENTED_EDGE('',*,*,#20828,.T.);
#29814=ORIENTED_EDGE('',*,*,#20816,.T.);
#29815=ORIENTED_EDGE('',*,*,#20829,.T.);
#29816=ORIENTED_EDGE('',*,*,#20810,.F.);
#29817=ORIENTED_EDGE('',*,*,#20830,.F.);
#29818=ORIENTED_EDGE('',*,*,#20831,.T.);
#29819=ORIENTED_EDGE('',*,*,#20829,.F.);
#29820=ORIENTED_EDGE('',*,*,#20831,.F.);
#29821=ORIENTED_EDGE('',*,*,#20801,.F.);
#29822=ORIENTED_EDGE('',*,*,#20830,.T.);
#29823=ORIENTED_EDGE('',*,*,#20832,.T.);
#29824=ORIENTED_EDGE('',*,*,#20833,.T.);
#29825=ORIENTED_EDGE('',*,*,#20834,.T.);
#29826=ORIENTED_EDGE('',*,*,#20835,.F.);
#29827=ORIENTED_EDGE('',*,*,#20834,.F.);
#29828=ORIENTED_EDGE('',*,*,#20836,.T.);
#29829=ORIENTED_EDGE('',*,*,#20837,.T.);
#29830=ORIENTED_EDGE('',*,*,#20838,.T.);
#29831=ORIENTED_EDGE('',*,*,#20839,.F.);
#29832=ORIENTED_EDGE('',*,*,#20838,.F.);
#29833=ORIENTED_EDGE('',*,*,#20839,.T.);
#29834=ORIENTED_EDGE('',*,*,#20840,.F.);
#29835=ORIENTED_EDGE('',*,*,#20841,.T.);
#29836=ORIENTED_EDGE('',*,*,#20842,.F.);
#29837=ORIENTED_EDGE('',*,*,#20843,.F.);
#29838=ORIENTED_EDGE('',*,*,#20844,.F.);
#29839=ORIENTED_EDGE('',*,*,#20845,.T.);
#29840=ORIENTED_EDGE('',*,*,#20842,.T.);
#29841=ORIENTED_EDGE('',*,*,#20846,.T.);
#29842=ORIENTED_EDGE('',*,*,#20847,.F.);
#29843=ORIENTED_EDGE('',*,*,#20548,.T.);
#29844=ORIENTED_EDGE('',*,*,#20844,.T.);
#29845=ORIENTED_EDGE('',*,*,#20848,.T.);
#29846=ORIENTED_EDGE('',*,*,#20849,.F.);
#29847=ORIENTED_EDGE('',*,*,#20850,.T.);
#29848=ORIENTED_EDGE('',*,*,#20851,.T.);
#29849=ORIENTED_EDGE('',*,*,#20852,.T.);
#29850=ORIENTED_EDGE('',*,*,#20853,.T.);
#29851=ORIENTED_EDGE('',*,*,#20854,.T.);
#29852=ORIENTED_EDGE('',*,*,#20855,.T.);
#29853=ORIENTED_EDGE('',*,*,#20856,.F.);
#29854=ORIENTED_EDGE('',*,*,#20855,.F.);
#29855=ORIENTED_EDGE('',*,*,#20542,.F.);
#29856=ORIENTED_EDGE('',*,*,#20857,.F.);
#29857=ORIENTED_EDGE('',*,*,#20840,.T.);
#29858=ORIENTED_EDGE('',*,*,#20858,.T.);
#29859=ORIENTED_EDGE('',*,*,#20835,.T.);
#29860=ORIENTED_EDGE('',*,*,#20856,.T.);
#29861=ORIENTED_EDGE('',*,*,#20859,.T.);
#29862=ORIENTED_EDGE('',*,*,#20860,.T.);
#29863=ORIENTED_EDGE('',*,*,#20861,.T.);
#29864=ORIENTED_EDGE('',*,*,#20862,.T.);
#29865=ORIENTED_EDGE('',*,*,#20863,.T.);
#29866=ORIENTED_EDGE('',*,*,#20864,.T.);
#29867=ORIENTED_EDGE('',*,*,#20865,.T.);
#29868=ORIENTED_EDGE('',*,*,#20866,.F.);
#29869=ORIENTED_EDGE('',*,*,#20864,.F.);
#29870=ORIENTED_EDGE('',*,*,#20867,.T.);
#29871=ORIENTED_EDGE('',*,*,#20868,.T.);
#29872=ORIENTED_EDGE('',*,*,#20867,.F.);
#29873=ORIENTED_EDGE('',*,*,#20863,.F.);
#29874=ORIENTED_EDGE('',*,*,#20869,.T.);
#29875=ORIENTED_EDGE('',*,*,#20870,.T.);
#29876=ORIENTED_EDGE('',*,*,#20871,.F.);
#29877=ORIENTED_EDGE('',*,*,#20869,.F.);
#29878=ORIENTED_EDGE('',*,*,#20862,.F.);
#29879=ORIENTED_EDGE('',*,*,#20872,.T.);
#29880=ORIENTED_EDGE('',*,*,#20870,.F.);
#29881=ORIENTED_EDGE('',*,*,#20861,.F.);
#29882=ORIENTED_EDGE('',*,*,#20873,.T.);
#29883=ORIENTED_EDGE('',*,*,#20874,.T.);
#29884=ORIENTED_EDGE('',*,*,#20873,.F.);
#29885=ORIENTED_EDGE('',*,*,#20860,.F.);
#29886=ORIENTED_EDGE('',*,*,#20875,.T.);
#29887=ORIENTED_EDGE('',*,*,#20876,.T.);
#29888=ORIENTED_EDGE('',*,*,#20875,.F.);
#29889=ORIENTED_EDGE('',*,*,#20859,.F.);
#29890=ORIENTED_EDGE('',*,*,#20866,.T.);
#29891=ORIENTED_EDGE('',*,*,#20877,.T.);
#29892=ORIENTED_EDGE('',*,*,#20878,.T.);
#29893=ORIENTED_EDGE('',*,*,#20879,.T.);
#29894=ORIENTED_EDGE('',*,*,#20880,.T.);
#29895=ORIENTED_EDGE('',*,*,#20881,.T.);
#29896=ORIENTED_EDGE('',*,*,#20882,.T.);
#29897=ORIENTED_EDGE('',*,*,#20883,.T.);
#29898=ORIENTED_EDGE('',*,*,#20884,.F.);
#29899=ORIENTED_EDGE('',*,*,#20882,.F.);
#29900=ORIENTED_EDGE('',*,*,#20885,.T.);
#29901=ORIENTED_EDGE('',*,*,#20886,.T.);
#29902=ORIENTED_EDGE('',*,*,#20885,.F.);
#29903=ORIENTED_EDGE('',*,*,#20881,.F.);
#29904=ORIENTED_EDGE('',*,*,#20887,.T.);
#29905=ORIENTED_EDGE('',*,*,#20888,.T.);
#29906=ORIENTED_EDGE('',*,*,#20889,.F.);
#29907=ORIENTED_EDGE('',*,*,#20887,.F.);
#29908=ORIENTED_EDGE('',*,*,#20880,.F.);
#29909=ORIENTED_EDGE('',*,*,#20890,.T.);
#29910=ORIENTED_EDGE('',*,*,#20888,.F.);
#29911=ORIENTED_EDGE('',*,*,#20879,.F.);
#29912=ORIENTED_EDGE('',*,*,#20891,.T.);
#29913=ORIENTED_EDGE('',*,*,#20892,.T.);
#29914=ORIENTED_EDGE('',*,*,#20891,.F.);
#29915=ORIENTED_EDGE('',*,*,#20878,.F.);
#29916=ORIENTED_EDGE('',*,*,#20893,.T.);
#29917=ORIENTED_EDGE('',*,*,#20894,.T.);
#29918=ORIENTED_EDGE('',*,*,#20893,.F.);
#29919=ORIENTED_EDGE('',*,*,#20877,.F.);
#29920=ORIENTED_EDGE('',*,*,#20884,.T.);
#29921=ORIENTED_EDGE('',*,*,#20895,.T.);
#29922=ORIENTED_EDGE('',*,*,#20871,.T.);
#29923=ORIENTED_EDGE('',*,*,#20872,.F.);
#29924=ORIENTED_EDGE('',*,*,#20874,.F.);
#29925=ORIENTED_EDGE('',*,*,#20876,.F.);
#29926=ORIENTED_EDGE('',*,*,#20865,.F.);
#29927=ORIENTED_EDGE('',*,*,#20868,.F.);
#29928=ORIENTED_EDGE('',*,*,#20896,.T.);
#29929=ORIENTED_EDGE('',*,*,#20897,.T.);
#29930=ORIENTED_EDGE('',*,*,#20898,.T.);
#29931=ORIENTED_EDGE('',*,*,#20895,.F.);
#29932=ORIENTED_EDGE('',*,*,#20898,.F.);
#29933=ORIENTED_EDGE('',*,*,#20899,.F.);
#29934=ORIENTED_EDGE('',*,*,#20900,.T.);
#29935=ORIENTED_EDGE('',*,*,#20896,.F.);
#29936=ORIENTED_EDGE('',*,*,#20897,.F.);
#29937=ORIENTED_EDGE('',*,*,#20900,.F.);
#29938=ORIENTED_EDGE('',*,*,#20901,.F.);
#29939=ORIENTED_EDGE('',*,*,#20902,.F.);
#29940=ORIENTED_EDGE('',*,*,#20903,.T.);
#29941=ORIENTED_EDGE('',*,*,#20904,.T.);
#29942=ORIENTED_EDGE('',*,*,#20903,.F.);
#29943=ORIENTED_EDGE('',*,*,#20904,.F.);
#29944=ORIENTED_EDGE('',*,*,#20905,.T.);
#29945=ORIENTED_EDGE('',*,*,#20889,.T.);
#29946=ORIENTED_EDGE('',*,*,#20890,.F.);
#29947=ORIENTED_EDGE('',*,*,#20892,.F.);
#29948=ORIENTED_EDGE('',*,*,#20894,.F.);
#29949=ORIENTED_EDGE('',*,*,#20883,.F.);
#29950=ORIENTED_EDGE('',*,*,#20886,.F.);
#29951=ORIENTED_EDGE('',*,*,#20906,.T.);
#29952=ORIENTED_EDGE('',*,*,#20907,.T.);
#29953=ORIENTED_EDGE('',*,*,#20908,.T.);
#29954=ORIENTED_EDGE('',*,*,#20905,.F.);
#29955=ORIENTED_EDGE('',*,*,#20908,.F.);
#29956=ORIENTED_EDGE('',*,*,#20909,.T.);
#29957=ORIENTED_EDGE('',*,*,#20910,.T.);
#29958=ORIENTED_EDGE('',*,*,#20911,.T.);
#29959=ORIENTED_EDGE('',*,*,#20912,.T.);
#29960=ORIENTED_EDGE('',*,*,#20913,.T.);
#29961=ORIENTED_EDGE('',*,*,#20914,.T.);
#29962=ORIENTED_EDGE('',*,*,#20915,.T.);
#29963=ORIENTED_EDGE('',*,*,#20916,.F.);
#29964=ORIENTED_EDGE('',*,*,#20914,.F.);
#29965=ORIENTED_EDGE('',*,*,#20917,.T.);
#29966=ORIENTED_EDGE('',*,*,#20918,.T.);
#29967=ORIENTED_EDGE('',*,*,#20917,.F.);
#29968=ORIENTED_EDGE('',*,*,#20913,.F.);
#29969=ORIENTED_EDGE('',*,*,#20919,.T.);
#29970=ORIENTED_EDGE('',*,*,#20920,.T.);
#29971=ORIENTED_EDGE('',*,*,#20921,.F.);
#29972=ORIENTED_EDGE('',*,*,#20919,.F.);
#29973=ORIENTED_EDGE('',*,*,#20912,.F.);
#29974=ORIENTED_EDGE('',*,*,#20922,.T.);
#29975=ORIENTED_EDGE('',*,*,#20920,.F.);
#29976=ORIENTED_EDGE('',*,*,#20911,.F.);
#29977=ORIENTED_EDGE('',*,*,#20923,.T.);
#29978=ORIENTED_EDGE('',*,*,#20924,.T.);
#29979=ORIENTED_EDGE('',*,*,#20923,.F.);
#29980=ORIENTED_EDGE('',*,*,#20910,.F.);
#29981=ORIENTED_EDGE('',*,*,#20925,.T.);
#29982=ORIENTED_EDGE('',*,*,#20926,.T.);
#29983=ORIENTED_EDGE('',*,*,#20925,.F.);
#29984=ORIENTED_EDGE('',*,*,#20909,.F.);
#29985=ORIENTED_EDGE('',*,*,#20916,.T.);
#29986=ORIENTED_EDGE('',*,*,#20927,.T.);
#29987=ORIENTED_EDGE('',*,*,#20928,.T.);
#29988=ORIENTED_EDGE('',*,*,#20929,.T.);
#29989=ORIENTED_EDGE('',*,*,#20930,.T.);
#29990=ORIENTED_EDGE('',*,*,#20931,.T.);
#29991=ORIENTED_EDGE('',*,*,#20932,.T.);
#29992=ORIENTED_EDGE('',*,*,#20933,.T.);
#29993=ORIENTED_EDGE('',*,*,#20934,.F.);
#29994=ORIENTED_EDGE('',*,*,#20932,.F.);
#29995=ORIENTED_EDGE('',*,*,#20935,.T.);
#29996=ORIENTED_EDGE('',*,*,#20936,.T.);
#29997=ORIENTED_EDGE('',*,*,#20935,.F.);
#29998=ORIENTED_EDGE('',*,*,#20931,.F.);
#29999=ORIENTED_EDGE('',*,*,#20937,.T.);
#30000=ORIENTED_EDGE('',*,*,#20938,.T.);
#30001=ORIENTED_EDGE('',*,*,#20939,.F.);
#30002=ORIENTED_EDGE('',*,*,#20937,.F.);
#30003=ORIENTED_EDGE('',*,*,#20930,.F.);
#30004=ORIENTED_EDGE('',*,*,#20940,.T.);
#30005=ORIENTED_EDGE('',*,*,#20938,.F.);
#30006=ORIENTED_EDGE('',*,*,#20929,.F.);
#30007=ORIENTED_EDGE('',*,*,#20941,.T.);
#30008=ORIENTED_EDGE('',*,*,#20942,.T.);
#30009=ORIENTED_EDGE('',*,*,#20941,.F.);
#30010=ORIENTED_EDGE('',*,*,#20928,.F.);
#30011=ORIENTED_EDGE('',*,*,#20943,.T.);
#30012=ORIENTED_EDGE('',*,*,#20944,.T.);
#30013=ORIENTED_EDGE('',*,*,#20943,.F.);
#30014=ORIENTED_EDGE('',*,*,#20927,.F.);
#30015=ORIENTED_EDGE('',*,*,#20934,.T.);
#30016=ORIENTED_EDGE('',*,*,#20945,.T.);
#30017=ORIENTED_EDGE('',*,*,#20939,.T.);
#30018=ORIENTED_EDGE('',*,*,#20940,.F.);
#30019=ORIENTED_EDGE('',*,*,#20942,.F.);
#30020=ORIENTED_EDGE('',*,*,#20944,.F.);
#30021=ORIENTED_EDGE('',*,*,#20933,.F.);
#30022=ORIENTED_EDGE('',*,*,#20936,.F.);
#30023=ORIENTED_EDGE('',*,*,#20946,.T.);
#30024=ORIENTED_EDGE('',*,*,#20947,.T.);
#30025=ORIENTED_EDGE('',*,*,#20948,.T.);
#30026=ORIENTED_EDGE('',*,*,#20945,.F.);
#30027=ORIENTED_EDGE('',*,*,#20948,.F.);
#30028=ORIENTED_EDGE('',*,*,#20949,.F.);
#30029=ORIENTED_EDGE('',*,*,#20950,.T.);
#30030=ORIENTED_EDGE('',*,*,#20946,.F.);
#30031=ORIENTED_EDGE('',*,*,#20947,.F.);
#30032=ORIENTED_EDGE('',*,*,#20950,.F.);
#30033=ORIENTED_EDGE('',*,*,#20951,.F.);
#30034=ORIENTED_EDGE('',*,*,#20952,.F.);
#30035=ORIENTED_EDGE('',*,*,#20953,.T.);
#30036=ORIENTED_EDGE('',*,*,#20954,.T.);
#30037=ORIENTED_EDGE('',*,*,#20953,.F.);
#30038=ORIENTED_EDGE('',*,*,#20954,.F.);
#30039=ORIENTED_EDGE('',*,*,#20955,.T.);
#30040=ORIENTED_EDGE('',*,*,#20921,.T.);
#30041=ORIENTED_EDGE('',*,*,#20922,.F.);
#30042=ORIENTED_EDGE('',*,*,#20924,.F.);
#30043=ORIENTED_EDGE('',*,*,#20926,.F.);
#30044=ORIENTED_EDGE('',*,*,#20915,.F.);
#30045=ORIENTED_EDGE('',*,*,#20918,.F.);
#30046=ORIENTED_EDGE('',*,*,#20956,.T.);
#30047=ORIENTED_EDGE('',*,*,#20957,.T.);
#30048=ORIENTED_EDGE('',*,*,#20958,.T.);
#30049=ORIENTED_EDGE('',*,*,#20955,.F.);
#30050=ORIENTED_EDGE('',*,*,#20958,.F.);
#30051=ORIENTED_EDGE('',*,*,#20959,.F.);
#30052=ORIENTED_EDGE('',*,*,#20960,.T.);
#30053=ORIENTED_EDGE('',*,*,#20956,.F.);
#30054=ORIENTED_EDGE('',*,*,#20957,.F.);
#30055=ORIENTED_EDGE('',*,*,#20960,.F.);
#30056=ORIENTED_EDGE('',*,*,#20853,.F.);
#30057=ORIENTED_EDGE('',*,*,#20854,.F.);
#30058=ORIENTED_EDGE('',*,*,#20961,.T.);
#30059=ORIENTED_EDGE('',*,*,#20962,.T.);
#30060=ORIENTED_EDGE('',*,*,#20961,.F.);
#30061=ORIENTED_EDGE('',*,*,#20962,.F.);
#30062=ORIENTED_EDGE('',*,*,#20951,.T.);
#30063=ORIENTED_EDGE('',*,*,#20952,.T.);
#30064=ORIENTED_EDGE('',*,*,#20963,.T.);
#30065=ORIENTED_EDGE('',*,*,#20851,.F.);
#30066=ORIENTED_EDGE('',*,*,#20963,.F.);
#30067=ORIENTED_EDGE('',*,*,#20901,.T.);
#30068=ORIENTED_EDGE('',*,*,#20902,.T.);
#30069=ORIENTED_EDGE('',*,*,#20964,.T.);
#30070=ORIENTED_EDGE('',*,*,#20852,.F.);
#30071=ORIENTED_EDGE('',*,*,#20964,.F.);
#30072=ORIENTED_EDGE('',*,*,#20965,.F.);
#30073=ORIENTED_EDGE('',*,*,#20832,.F.);
#30074=ORIENTED_EDGE('',*,*,#20833,.F.);
#30075=ORIENTED_EDGE('',*,*,#20966,.T.);
#30076=ORIENTED_EDGE('',*,*,#20965,.T.);
#30077=ORIENTED_EDGE('',*,*,#20966,.F.);
#30078=ORIENTED_EDGE('',*,*,#20967,.F.);
#30079=ORIENTED_EDGE('',*,*,#20968,.T.);
#30080=ORIENTED_EDGE('',*,*,#20906,.F.);
#30081=ORIENTED_EDGE('',*,*,#20907,.F.);
#30082=ORIENTED_EDGE('',*,*,#20968,.F.);
#30083=ORIENTED_EDGE('',*,*,#20969,.T.);
#30084=ORIENTED_EDGE('',*,*,#20970,.T.);
#30085=ORIENTED_EDGE('',*,*,#20971,.T.);
#30086=ORIENTED_EDGE('',*,*,#20972,.T.);
#30087=ORIENTED_EDGE('',*,*,#20971,.F.);
#30088=ORIENTED_EDGE('',*,*,#20959,.T.);
#30089=ORIENTED_EDGE('',*,*,#20949,.T.);
#30090=ORIENTED_EDGE('',*,*,#20969,.F.);
#30091=ORIENTED_EDGE('',*,*,#20970,.F.);
#30092=ORIENTED_EDGE('',*,*,#20973,.T.);
#30093=ORIENTED_EDGE('',*,*,#20847,.T.);
#30094=ORIENTED_EDGE('',*,*,#20973,.F.);
#30095=ORIENTED_EDGE('',*,*,#20848,.F.);
#30096=ORIENTED_EDGE('',*,*,#20846,.F.);
#30097=ORIENTED_EDGE('',*,*,#20841,.F.);
#30098=ORIENTED_EDGE('',*,*,#20857,.T.);
#30099=ORIENTED_EDGE('',*,*,#20545,.F.);
#30100=ORIENTED_EDGE('',*,*,#20974,.F.);
#30101=ORIENTED_EDGE('',*,*,#20544,.F.);
#30102=ORIENTED_EDGE('',*,*,#20975,.T.);
#30103=ORIENTED_EDGE('',*,*,#20849,.T.);
#30104=ORIENTED_EDGE('',*,*,#20974,.T.);
#30105=ORIENTED_EDGE('',*,*,#20543,.F.);
#30106=ORIENTED_EDGE('',*,*,#20858,.F.);
#30107=ORIENTED_EDGE('',*,*,#20843,.T.);
#30108=ORIENTED_EDGE('',*,*,#20845,.F.);
#30109=ORIENTED_EDGE('',*,*,#20850,.F.);
#30110=ORIENTED_EDGE('',*,*,#20975,.F.);
#30111=ORIENTED_EDGE('',*,*,#20976,.T.);
#30112=ORIENTED_EDGE('',*,*,#20977,.T.);
#30113=ORIENTED_EDGE('',*,*,#20836,.F.);
#30114=ORIENTED_EDGE('',*,*,#20837,.F.);
#30115=ORIENTED_EDGE('',*,*,#20977,.F.);
#30116=ORIENTED_EDGE('',*,*,#20899,.T.);
#30117=ORIENTED_EDGE('',*,*,#20967,.T.);
#30118=ORIENTED_EDGE('',*,*,#20780,.F.);
#30119=ORIENTED_EDGE('',*,*,#20978,.F.);
#30120=ORIENTED_EDGE('',*,*,#20979,.T.);
#30121=ORIENTED_EDGE('',*,*,#20972,.F.);
#30122=ORIENTED_EDGE('',*,*,#20781,.F.);
#30123=ORIENTED_EDGE('',*,*,#20980,.T.);
#30124=ORIENTED_EDGE('',*,*,#20979,.F.);
#30125=ORIENTED_EDGE('',*,*,#20980,.F.);
#30126=ORIENTED_EDGE('',*,*,#20784,.F.);
#30127=ORIENTED_EDGE('',*,*,#20978,.T.);
#30128=ORIENTED_EDGE('',*,*,#20981,.T.);
#30129=ORIENTED_EDGE('',*,*,#20982,.T.);
#30130=ORIENTED_EDGE('',*,*,#20981,.F.);
#30131=ORIENTED_EDGE('',*,*,#20812,.F.);
#30132=ORIENTED_EDGE('',*,*,#20982,.F.);
#30133=ORIENTED_EDGE('',*,*,#20983,.T.);
#30134=ORIENTED_EDGE('',*,*,#20976,.F.);
#30135=ORIENTED_EDGE('',*,*,#20813,.F.);
#30136=ORIENTED_EDGE('',*,*,#20814,.F.);
#30137=ORIENTED_EDGE('',*,*,#20984,.T.);
#30138=ORIENTED_EDGE('',*,*,#20983,.F.);
#30139=ORIENTED_EDGE('',*,*,#20984,.F.);
#30140=ORIENTED_EDGE('',*,*,#20985,.F.);
#30141=ORIENTED_EDGE('',*,*,#20986,.F.);
#30142=ORIENTED_EDGE('',*,*,#20987,.F.);
#30143=ORIENTED_EDGE('',*,*,#20988,.F.);
#30144=ORIENTED_EDGE('',*,*,#20989,.F.);
#30145=ORIENTED_EDGE('',*,*,#20990,.F.);
#30146=ORIENTED_EDGE('',*,*,#20991,.F.);
#30147=ORIENTED_EDGE('',*,*,#20992,.F.);
#30148=ORIENTED_EDGE('',*,*,#20993,.F.);
#30149=ORIENTED_EDGE('',*,*,#20994,.F.);
#30150=ORIENTED_EDGE('',*,*,#20995,.F.);
#30151=ORIENTED_EDGE('',*,*,#20996,.F.);
#30152=ORIENTED_EDGE('',*,*,#20997,.F.);
#30153=ORIENTED_EDGE('',*,*,#20998,.F.);
#30154=ORIENTED_EDGE('',*,*,#20995,.T.);
#30155=ORIENTED_EDGE('',*,*,#20999,.T.);
#30156=ORIENTED_EDGE('',*,*,#20988,.T.);
#30157=ORIENTED_EDGE('',*,*,#21000,.T.);
#30158=ORIENTED_EDGE('',*,*,#21001,.T.);
#30159=ORIENTED_EDGE('',*,*,#20825,.F.);
#30160=ORIENTED_EDGE('',*,*,#21002,.F.);
#30161=ORIENTED_EDGE('',*,*,#21003,.T.);
#30162=ORIENTED_EDGE('',*,*,#20990,.T.);
#30163=ORIENTED_EDGE('',*,*,#21004,.T.);
#30164=ORIENTED_EDGE('',*,*,#21002,.T.);
#30165=ORIENTED_EDGE('',*,*,#20824,.F.);
#30166=ORIENTED_EDGE('',*,*,#21005,.F.);
#30167=ORIENTED_EDGE('',*,*,#21006,.F.);
#30168=ORIENTED_EDGE('',*,*,#20993,.T.);
#30169=ORIENTED_EDGE('',*,*,#21007,.F.);
#30170=ORIENTED_EDGE('',*,*,#21003,.F.);
#30171=ORIENTED_EDGE('',*,*,#21008,.F.);
#30172=ORIENTED_EDGE('',*,*,#20991,.T.);
#30173=ORIENTED_EDGE('',*,*,#20999,.F.);
#30174=ORIENTED_EDGE('',*,*,#21004,.F.);
#30175=ORIENTED_EDGE('',*,*,#20989,.T.);
#30176=ORIENTED_EDGE('',*,*,#21009,.F.);
#30177=ORIENTED_EDGE('',*,*,#20985,.T.);
#30178=ORIENTED_EDGE('',*,*,#21010,.F.);
#30179=ORIENTED_EDGE('',*,*,#21011,.F.);
#30180=ORIENTED_EDGE('',*,*,#21000,.F.);
#30181=ORIENTED_EDGE('',*,*,#20987,.T.);
#30182=ORIENTED_EDGE('',*,*,#21011,.T.);
#30183=ORIENTED_EDGE('',*,*,#20986,.T.);
#30184=ORIENTED_EDGE('',*,*,#21009,.T.);
#30185=ORIENTED_EDGE('',*,*,#21012,.T.);
#30186=ORIENTED_EDGE('',*,*,#20826,.F.);
#30187=ORIENTED_EDGE('',*,*,#21001,.F.);
#30188=ORIENTED_EDGE('',*,*,#21010,.T.);
#30189=ORIENTED_EDGE('',*,*,#20996,.T.);
#30190=ORIENTED_EDGE('',*,*,#20998,.T.);
#30191=ORIENTED_EDGE('',*,*,#21013,.T.);
#30192=ORIENTED_EDGE('',*,*,#20827,.F.);
#30193=ORIENTED_EDGE('',*,*,#21012,.F.);
#30194=ORIENTED_EDGE('',*,*,#20997,.T.);
#30195=ORIENTED_EDGE('',*,*,#20994,.T.);
#30196=ORIENTED_EDGE('',*,*,#21006,.T.);
#30197=ORIENTED_EDGE('',*,*,#21014,.T.);
#30198=ORIENTED_EDGE('',*,*,#20828,.F.);
#30199=ORIENTED_EDGE('',*,*,#21013,.F.);
#30200=ORIENTED_EDGE('',*,*,#21007,.T.);
#30201=ORIENTED_EDGE('',*,*,#20992,.T.);
#30202=ORIENTED_EDGE('',*,*,#21008,.T.);
#30203=ORIENTED_EDGE('',*,*,#21005,.T.);
#30204=ORIENTED_EDGE('',*,*,#20823,.F.);
#30205=ORIENTED_EDGE('',*,*,#21014,.F.);
#30206=ORIENTED_EDGE('',*,*,#21015,.F.);
#30207=ORIENTED_EDGE('',*,*,#21016,.F.);
#30208=ORIENTED_EDGE('',*,*,#21017,.F.);
#30209=ORIENTED_EDGE('',*,*,#21018,.F.);
#30210=ORIENTED_EDGE('',*,*,#21019,.F.);
#30211=ORIENTED_EDGE('',*,*,#21020,.F.);
#30212=ORIENTED_EDGE('',*,*,#21021,.F.);
#30213=ORIENTED_EDGE('',*,*,#21022,.F.);
#30214=ORIENTED_EDGE('',*,*,#21023,.F.);
#30215=ORIENTED_EDGE('',*,*,#21024,.F.);
#30216=ORIENTED_EDGE('',*,*,#21025,.F.);
#30217=ORIENTED_EDGE('',*,*,#21026,.F.);
#30218=ORIENTED_EDGE('',*,*,#21027,.F.);
#30219=ORIENTED_EDGE('',*,*,#21028,.F.);
#30220=ORIENTED_EDGE('',*,*,#21025,.T.);
#30221=ORIENTED_EDGE('',*,*,#21029,.T.);
#30222=ORIENTED_EDGE('',*,*,#21018,.T.);
#30223=ORIENTED_EDGE('',*,*,#21030,.T.);
#30224=ORIENTED_EDGE('',*,*,#21031,.T.);
#30225=ORIENTED_EDGE('',*,*,#20819,.F.);
#30226=ORIENTED_EDGE('',*,*,#21032,.F.);
#30227=ORIENTED_EDGE('',*,*,#21033,.T.);
#30228=ORIENTED_EDGE('',*,*,#21020,.T.);
#30229=ORIENTED_EDGE('',*,*,#21034,.T.);
#30230=ORIENTED_EDGE('',*,*,#21032,.T.);
#30231=ORIENTED_EDGE('',*,*,#20818,.F.);
#30232=ORIENTED_EDGE('',*,*,#21035,.F.);
#30233=ORIENTED_EDGE('',*,*,#21036,.F.);
#30234=ORIENTED_EDGE('',*,*,#21023,.T.);
#30235=ORIENTED_EDGE('',*,*,#21037,.F.);
#30236=ORIENTED_EDGE('',*,*,#21033,.F.);
#30237=ORIENTED_EDGE('',*,*,#21038,.F.);
#30238=ORIENTED_EDGE('',*,*,#21021,.T.);
#30239=ORIENTED_EDGE('',*,*,#21029,.F.);
#30240=ORIENTED_EDGE('',*,*,#21034,.F.);
#30241=ORIENTED_EDGE('',*,*,#21019,.T.);
#30242=ORIENTED_EDGE('',*,*,#21039,.F.);
#30243=ORIENTED_EDGE('',*,*,#21015,.T.);
#30244=ORIENTED_EDGE('',*,*,#21040,.F.);
#30245=ORIENTED_EDGE('',*,*,#21041,.F.);
#30246=ORIENTED_EDGE('',*,*,#21030,.F.);
#30247=ORIENTED_EDGE('',*,*,#21017,.T.);
#30248=ORIENTED_EDGE('',*,*,#21041,.T.);
#30249=ORIENTED_EDGE('',*,*,#21016,.T.);
#30250=ORIENTED_EDGE('',*,*,#21039,.T.);
#30251=ORIENTED_EDGE('',*,*,#21042,.T.);
#30252=ORIENTED_EDGE('',*,*,#20820,.F.);
#30253=ORIENTED_EDGE('',*,*,#21031,.F.);
#30254=ORIENTED_EDGE('',*,*,#21040,.T.);
#30255=ORIENTED_EDGE('',*,*,#21026,.T.);
#30256=ORIENTED_EDGE('',*,*,#21028,.T.);
#30257=ORIENTED_EDGE('',*,*,#21043,.T.);
#30258=ORIENTED_EDGE('',*,*,#20821,.F.);
#30259=ORIENTED_EDGE('',*,*,#21042,.F.);
#30260=ORIENTED_EDGE('',*,*,#21027,.T.);
#30261=ORIENTED_EDGE('',*,*,#21024,.T.);
#30262=ORIENTED_EDGE('',*,*,#21036,.T.);
#30263=ORIENTED_EDGE('',*,*,#21044,.T.);
#30264=ORIENTED_EDGE('',*,*,#20822,.F.);
#30265=ORIENTED_EDGE('',*,*,#21043,.F.);
#30266=ORIENTED_EDGE('',*,*,#21037,.T.);
#30267=ORIENTED_EDGE('',*,*,#21022,.T.);
#30268=ORIENTED_EDGE('',*,*,#21038,.T.);
#30269=ORIENTED_EDGE('',*,*,#21035,.T.);
#30270=ORIENTED_EDGE('',*,*,#20817,.F.);
#30271=ORIENTED_EDGE('',*,*,#21044,.F.);
#30272=ORIENTED_EDGE('',*,*,#21045,.T.);
#30273=ORIENTED_EDGE('',*,*,#20709,.T.);
#30274=ORIENTED_EDGE('',*,*,#21046,.T.);
#30275=ORIENTED_EDGE('',*,*,#20701,.T.);
#30276=ORIENTED_EDGE('',*,*,#21047,.T.);
#30277=ORIENTED_EDGE('',*,*,#20693,.T.);
#30278=ORIENTED_EDGE('',*,*,#21048,.T.);
#30279=ORIENTED_EDGE('',*,*,#21049,.T.);
#30280=ORIENTED_EDGE('',*,*,#21050,.F.);
#30281=ORIENTED_EDGE('',*,*,#21049,.F.);
#30282=ORIENTED_EDGE('',*,*,#21051,.T.);
#30283=ORIENTED_EDGE('',*,*,#21052,.T.);
#30284=ORIENTED_EDGE('',*,*,#21053,.F.);
#30285=ORIENTED_EDGE('',*,*,#21052,.F.);
#30286=ORIENTED_EDGE('',*,*,#21054,.F.);
#30287=ORIENTED_EDGE('',*,*,#21055,.T.);
#30288=ORIENTED_EDGE('',*,*,#20510,.F.);
#30289=ORIENTED_EDGE('',*,*,#21055,.F.);
#30290=ORIENTED_EDGE('',*,*,#21056,.T.);
#30291=ORIENTED_EDGE('',*,*,#21057,.T.);
#30292=ORIENTED_EDGE('',*,*,#21058,.F.);
#30293=ORIENTED_EDGE('',*,*,#21057,.F.);
#30294=ORIENTED_EDGE('',*,*,#21059,.T.);
#30295=ORIENTED_EDGE('',*,*,#21060,.T.);
#30296=ORIENTED_EDGE('',*,*,#21061,.F.);
#30297=ORIENTED_EDGE('',*,*,#21060,.F.);
#30298=ORIENTED_EDGE('',*,*,#21062,.T.);
#30299=ORIENTED_EDGE('',*,*,#21063,.T.);
#30300=ORIENTED_EDGE('',*,*,#21064,.F.);
#30301=ORIENTED_EDGE('',*,*,#21063,.F.);
#30302=ORIENTED_EDGE('',*,*,#21065,.T.);
#30303=ORIENTED_EDGE('',*,*,#21066,.T.);
#30304=ORIENTED_EDGE('',*,*,#21067,.F.);
#30305=ORIENTED_EDGE('',*,*,#21066,.F.);
#30306=ORIENTED_EDGE('',*,*,#21068,.F.);
#30307=ORIENTED_EDGE('',*,*,#21069,.T.);
#30308=ORIENTED_EDGE('',*,*,#21070,.T.);
#30309=ORIENTED_EDGE('',*,*,#21071,.T.);
#30310=ORIENTED_EDGE('',*,*,#21072,.T.);
#30311=ORIENTED_EDGE('',*,*,#21073,.T.);
#30312=ORIENTED_EDGE('',*,*,#21074,.T.);
#30313=ORIENTED_EDGE('',*,*,#21075,.T.);
#30314=ORIENTED_EDGE('',*,*,#21076,.T.);
#30315=ORIENTED_EDGE('',*,*,#21077,.F.);
#30316=ORIENTED_EDGE('',*,*,#21078,.F.);
#30317=ORIENTED_EDGE('',*,*,#21079,.T.);
#30318=ORIENTED_EDGE('',*,*,#21080,.T.);
#30319=ORIENTED_EDGE('',*,*,#21081,.F.);
#30320=ORIENTED_EDGE('',*,*,#21082,.F.);
#30321=ORIENTED_EDGE('',*,*,#21077,.T.);
#30322=ORIENTED_EDGE('',*,*,#21083,.T.);
#30323=ORIENTED_EDGE('',*,*,#21084,.F.);
#30324=ORIENTED_EDGE('',*,*,#21085,.F.);
#30325=ORIENTED_EDGE('',*,*,#21081,.T.);
#30326=ORIENTED_EDGE('',*,*,#21086,.T.);
#30327=ORIENTED_EDGE('',*,*,#21087,.F.);
#30328=ORIENTED_EDGE('',*,*,#21088,.F.);
#30329=ORIENTED_EDGE('',*,*,#21084,.T.);
#30330=ORIENTED_EDGE('',*,*,#21089,.T.);
#30331=ORIENTED_EDGE('',*,*,#21090,.F.);
#30332=ORIENTED_EDGE('',*,*,#21091,.F.);
#30333=ORIENTED_EDGE('',*,*,#21087,.T.);
#30334=ORIENTED_EDGE('',*,*,#21092,.T.);
#30335=ORIENTED_EDGE('',*,*,#21093,.F.);
#30336=ORIENTED_EDGE('',*,*,#21094,.F.);
#30337=ORIENTED_EDGE('',*,*,#21090,.T.);
#30338=ORIENTED_EDGE('',*,*,#21095,.F.);
#30339=ORIENTED_EDGE('',*,*,#21096,.F.);
#30340=ORIENTED_EDGE('',*,*,#21097,.T.);
#30341=ORIENTED_EDGE('',*,*,#21093,.T.);
#30342=ORIENTED_EDGE('',*,*,#21098,.T.);
#30343=ORIENTED_EDGE('',*,*,#21079,.F.);
#30344=ORIENTED_EDGE('',*,*,#21099,.F.);
#30345=ORIENTED_EDGE('',*,*,#21096,.T.);
#30346=ORIENTED_EDGE('',*,*,#21078,.T.);
#30347=ORIENTED_EDGE('',*,*,#21082,.T.);
#30348=ORIENTED_EDGE('',*,*,#21085,.T.);
#30349=ORIENTED_EDGE('',*,*,#21088,.T.);
#30350=ORIENTED_EDGE('',*,*,#21091,.T.);
#30351=ORIENTED_EDGE('',*,*,#21094,.T.);
#30352=ORIENTED_EDGE('',*,*,#21097,.F.);
#30353=ORIENTED_EDGE('',*,*,#21099,.T.);
#30354=ORIENTED_EDGE('',*,*,#21100,.T.);
#30355=ORIENTED_EDGE('',*,*,#21101,.F.);
#30356=ORIENTED_EDGE('',*,*,#21102,.F.);
#30357=ORIENTED_EDGE('',*,*,#21103,.T.);
#30358=ORIENTED_EDGE('',*,*,#21104,.T.);
#30359=ORIENTED_EDGE('',*,*,#21105,.F.);
#30360=ORIENTED_EDGE('',*,*,#21106,.F.);
#30361=ORIENTED_EDGE('',*,*,#21101,.T.);
#30362=ORIENTED_EDGE('',*,*,#21107,.T.);
#30363=ORIENTED_EDGE('',*,*,#21108,.F.);
#30364=ORIENTED_EDGE('',*,*,#21109,.F.);
#30365=ORIENTED_EDGE('',*,*,#21105,.T.);
#30366=ORIENTED_EDGE('',*,*,#21110,.T.);
#30367=ORIENTED_EDGE('',*,*,#21111,.F.);
#30368=ORIENTED_EDGE('',*,*,#21112,.F.);
#30369=ORIENTED_EDGE('',*,*,#21108,.T.);
#30370=ORIENTED_EDGE('',*,*,#21113,.T.);
#30371=ORIENTED_EDGE('',*,*,#21114,.F.);
#30372=ORIENTED_EDGE('',*,*,#21115,.F.);
#30373=ORIENTED_EDGE('',*,*,#21111,.T.);
#30374=ORIENTED_EDGE('',*,*,#21116,.T.);
#30375=ORIENTED_EDGE('',*,*,#21117,.F.);
#30376=ORIENTED_EDGE('',*,*,#21118,.F.);
#30377=ORIENTED_EDGE('',*,*,#21114,.T.);
#30378=ORIENTED_EDGE('',*,*,#21119,.F.);
#30379=ORIENTED_EDGE('',*,*,#21120,.F.);
#30380=ORIENTED_EDGE('',*,*,#21121,.T.);
#30381=ORIENTED_EDGE('',*,*,#21117,.T.);
#30382=ORIENTED_EDGE('',*,*,#21122,.T.);
#30383=ORIENTED_EDGE('',*,*,#21103,.F.);
#30384=ORIENTED_EDGE('',*,*,#21123,.F.);
#30385=ORIENTED_EDGE('',*,*,#21120,.T.);
#30386=ORIENTED_EDGE('',*,*,#21102,.T.);
#30387=ORIENTED_EDGE('',*,*,#21106,.T.);
#30388=ORIENTED_EDGE('',*,*,#21109,.T.);
#30389=ORIENTED_EDGE('',*,*,#21112,.T.);
#30390=ORIENTED_EDGE('',*,*,#21115,.T.);
#30391=ORIENTED_EDGE('',*,*,#21118,.T.);
#30392=ORIENTED_EDGE('',*,*,#21121,.F.);
#30393=ORIENTED_EDGE('',*,*,#21123,.T.);
#30394=ORIENTED_EDGE('',*,*,#21124,.T.);
#30395=ORIENTED_EDGE('',*,*,#21125,.F.);
#30396=ORIENTED_EDGE('',*,*,#21126,.F.);
#30397=ORIENTED_EDGE('',*,*,#21127,.T.);
#30398=ORIENTED_EDGE('',*,*,#21128,.T.);
#30399=ORIENTED_EDGE('',*,*,#21129,.F.);
#30400=ORIENTED_EDGE('',*,*,#21130,.F.);
#30401=ORIENTED_EDGE('',*,*,#21125,.T.);
#30402=ORIENTED_EDGE('',*,*,#21131,.T.);
#30403=ORIENTED_EDGE('',*,*,#21132,.F.);
#30404=ORIENTED_EDGE('',*,*,#21133,.F.);
#30405=ORIENTED_EDGE('',*,*,#21129,.T.);
#30406=ORIENTED_EDGE('',*,*,#21134,.T.);
#30407=ORIENTED_EDGE('',*,*,#21135,.F.);
#30408=ORIENTED_EDGE('',*,*,#21136,.F.);
#30409=ORIENTED_EDGE('',*,*,#21132,.T.);
#30410=ORIENTED_EDGE('',*,*,#21137,.T.);
#30411=ORIENTED_EDGE('',*,*,#21138,.F.);
#30412=ORIENTED_EDGE('',*,*,#21139,.F.);
#30413=ORIENTED_EDGE('',*,*,#21135,.T.);
#30414=ORIENTED_EDGE('',*,*,#21140,.T.);
#30415=ORIENTED_EDGE('',*,*,#21141,.F.);
#30416=ORIENTED_EDGE('',*,*,#21142,.F.);
#30417=ORIENTED_EDGE('',*,*,#21138,.T.);
#30418=ORIENTED_EDGE('',*,*,#21143,.F.);
#30419=ORIENTED_EDGE('',*,*,#21144,.F.);
#30420=ORIENTED_EDGE('',*,*,#21145,.T.);
#30421=ORIENTED_EDGE('',*,*,#21141,.T.);
#30422=ORIENTED_EDGE('',*,*,#21146,.T.);
#30423=ORIENTED_EDGE('',*,*,#21127,.F.);
#30424=ORIENTED_EDGE('',*,*,#21147,.F.);
#30425=ORIENTED_EDGE('',*,*,#21144,.T.);
#30426=ORIENTED_EDGE('',*,*,#21126,.T.);
#30427=ORIENTED_EDGE('',*,*,#21130,.T.);
#30428=ORIENTED_EDGE('',*,*,#21133,.T.);
#30429=ORIENTED_EDGE('',*,*,#21136,.T.);
#30430=ORIENTED_EDGE('',*,*,#21139,.T.);
#30431=ORIENTED_EDGE('',*,*,#21142,.T.);
#30432=ORIENTED_EDGE('',*,*,#21145,.F.);
#30433=ORIENTED_EDGE('',*,*,#21147,.T.);
#30434=ORIENTED_EDGE('',*,*,#21047,.F.);
#30435=ORIENTED_EDGE('',*,*,#21148,.T.);
#30436=ORIENTED_EDGE('',*,*,#21149,.F.);
#30437=ORIENTED_EDGE('',*,*,#21148,.F.);
#30438=ORIENTED_EDGE('',*,*,#21046,.F.);
#30439=ORIENTED_EDGE('',*,*,#21150,.T.);
#30440=ORIENTED_EDGE('',*,*,#21151,.F.);
#30441=ORIENTED_EDGE('',*,*,#21150,.F.);
#30442=ORIENTED_EDGE('',*,*,#21045,.F.);
#30443=ORIENTED_EDGE('',*,*,#21152,.T.);
#30444=ORIENTED_EDGE('',*,*,#21153,.F.);
#30445=ORIENTED_EDGE('',*,*,#21152,.F.);
#30446=ORIENTED_EDGE('',*,*,#21154,.T.);
#30447=ORIENTED_EDGE('',*,*,#21155,.F.);
#30448=ORIENTED_EDGE('',*,*,#21156,.F.);
#30449=ORIENTED_EDGE('',*,*,#21157,.F.);
#30450=ORIENTED_EDGE('',*,*,#21158,.T.);
#30451=ORIENTED_EDGE('',*,*,#21156,.T.);
#30452=ORIENTED_EDGE('',*,*,#21159,.T.);
#30453=ORIENTED_EDGE('',*,*,#21160,.F.);
#30454=ORIENTED_EDGE('',*,*,#21161,.F.);
#30455=ORIENTED_EDGE('',*,*,#21162,.F.);
#30456=ORIENTED_EDGE('',*,*,#21163,.T.);
#30457=ORIENTED_EDGE('',*,*,#21161,.T.);
#30458=ORIENTED_EDGE('',*,*,#21164,.F.);
#30459=ORIENTED_EDGE('',*,*,#21165,.T.);
#30460=ORIENTED_EDGE('',*,*,#21166,.F.);
#30461=ORIENTED_EDGE('',*,*,#21167,.F.);
#30462=ORIENTED_EDGE('',*,*,#21168,.T.);
#30463=ORIENTED_EDGE('',*,*,#21167,.T.);
#30464=ORIENTED_EDGE('',*,*,#21169,.F.);
#30465=ORIENTED_EDGE('',*,*,#21170,.F.);
#30466=ORIENTED_EDGE('',*,*,#21171,.T.);
#30467=ORIENTED_EDGE('',*,*,#21172,.F.);
#30468=ORIENTED_EDGE('',*,*,#21173,.F.);
#30469=ORIENTED_EDGE('',*,*,#21174,.F.);
#30470=ORIENTED_EDGE('',*,*,#21153,.T.);
#30471=ORIENTED_EDGE('',*,*,#21175,.F.);
#30472=ORIENTED_EDGE('',*,*,#21176,.F.);
#30473=ORIENTED_EDGE('',*,*,#21177,.F.);
#30474=ORIENTED_EDGE('',*,*,#21178,.F.);
#30475=ORIENTED_EDGE('',*,*,#21179,.T.);
#30476=ORIENTED_EDGE('',*,*,#21180,.F.);
#30477=ORIENTED_EDGE('',*,*,#21149,.T.);
#30478=ORIENTED_EDGE('',*,*,#21181,.F.);
#30479=ORIENTED_EDGE('',*,*,#21182,.F.);
#30480=ORIENTED_EDGE('',*,*,#21183,.F.);
#30481=ORIENTED_EDGE('',*,*,#21184,.F.);
#30482=ORIENTED_EDGE('',*,*,#21185,.T.);
#30483=ORIENTED_EDGE('',*,*,#21186,.F.);
#30484=ORIENTED_EDGE('',*,*,#21187,.T.);
#30485=ORIENTED_EDGE('',*,*,#21188,.F.);
#30486=ORIENTED_EDGE('',*,*,#21189,.T.);
#30487=ORIENTED_EDGE('',*,*,#21190,.T.);
#30488=ORIENTED_EDGE('',*,*,#21191,.T.);
#30489=ORIENTED_EDGE('',*,*,#21189,.F.);
#30490=ORIENTED_EDGE('',*,*,#21192,.T.);
#30491=ORIENTED_EDGE('',*,*,#20776,.F.);
#30492=ORIENTED_EDGE('',*,*,#21193,.T.);
#30493=ORIENTED_EDGE('',*,*,#21194,.T.);
#30494=ORIENTED_EDGE('',*,*,#21195,.T.);
#30495=ORIENTED_EDGE('',*,*,#21196,.T.);
#30496=ORIENTED_EDGE('',*,*,#21197,.T.);
#30497=ORIENTED_EDGE('',*,*,#20770,.F.);
#30498=ORIENTED_EDGE('',*,*,#21198,.T.);
#30499=ORIENTED_EDGE('',*,*,#20774,.F.);
#30500=ORIENTED_EDGE('',*,*,#21199,.T.);
#30501=ORIENTED_EDGE('',*,*,#21200,.T.);
#30502=ORIENTED_EDGE('',*,*,#21201,.T.);
#30503=ORIENTED_EDGE('',*,*,#20772,.F.);
#30504=ORIENTED_EDGE('',*,*,#21202,.T.);
#30505=ORIENTED_EDGE('',*,*,#21203,.T.);
#30506=ORIENTED_EDGE('',*,*,#21204,.T.);
#30507=ORIENTED_EDGE('',*,*,#21164,.T.);
#30508=ORIENTED_EDGE('',*,*,#21168,.F.);
#30509=ORIENTED_EDGE('',*,*,#21166,.T.);
#30510=ORIENTED_EDGE('',*,*,#21205,.T.);
#30511=ORIENTED_EDGE('',*,*,#21206,.F.);
#30512=ORIENTED_EDGE('',*,*,#21173,.T.);
#30513=ORIENTED_EDGE('',*,*,#21207,.T.);
#30514=ORIENTED_EDGE('',*,*,#21208,.F.);
#30515=ORIENTED_EDGE('',*,*,#21209,.T.);
#30516=ORIENTED_EDGE('',*,*,#21177,.T.);
#30517=ORIENTED_EDGE('',*,*,#21210,.T.);
#30518=ORIENTED_EDGE('',*,*,#21210,.F.);
#30519=ORIENTED_EDGE('',*,*,#21176,.T.);
#30520=ORIENTED_EDGE('',*,*,#21211,.T.);
#30521=ORIENTED_EDGE('',*,*,#21212,.T.);
#30522=ORIENTED_EDGE('',*,*,#21213,.T.);
#30523=ORIENTED_EDGE('',*,*,#21162,.T.);
#30524=ORIENTED_EDGE('',*,*,#21163,.F.);
#30525=ORIENTED_EDGE('',*,*,#21160,.T.);
#30526=ORIENTED_EDGE('',*,*,#21214,.T.);
#30527=ORIENTED_EDGE('',*,*,#21211,.F.);
#30528=ORIENTED_EDGE('',*,*,#21175,.T.);
#30529=ORIENTED_EDGE('',*,*,#21215,.T.);
#30530=ORIENTED_EDGE('',*,*,#21216,.F.);
#30531=ORIENTED_EDGE('',*,*,#21217,.T.);
#30532=ORIENTED_EDGE('',*,*,#21183,.T.);
#30533=ORIENTED_EDGE('',*,*,#21218,.T.);
#30534=ORIENTED_EDGE('',*,*,#21218,.F.);
#30535=ORIENTED_EDGE('',*,*,#21182,.T.);
#30536=ORIENTED_EDGE('',*,*,#21219,.T.);
#30537=ORIENTED_EDGE('',*,*,#21220,.T.);
#30538=ORIENTED_EDGE('',*,*,#21221,.T.);
#30539=ORIENTED_EDGE('',*,*,#21157,.T.);
#30540=ORIENTED_EDGE('',*,*,#21158,.F.);
#30541=ORIENTED_EDGE('',*,*,#21155,.T.);
#30542=ORIENTED_EDGE('',*,*,#21222,.T.);
#30543=ORIENTED_EDGE('',*,*,#21219,.F.);
#30544=ORIENTED_EDGE('',*,*,#21181,.T.);
#30545=ORIENTED_EDGE('',*,*,#21223,.T.);
#30546=ORIENTED_EDGE('',*,*,#21224,.F.);
#30547=ORIENTED_EDGE('',*,*,#21225,.T.);
#30548=ORIENTED_EDGE('',*,*,#21226,.T.);
#30549=ORIENTED_EDGE('',*,*,#21227,.T.);
#30550=ORIENTED_EDGE('',*,*,#21227,.F.);
#30551=ORIENTED_EDGE('',*,*,#21228,.T.);
#30552=ORIENTED_EDGE('',*,*,#21229,.T.);
#30553=ORIENTED_EDGE('',*,*,#21230,.T.);
#30554=ORIENTED_EDGE('',*,*,#21231,.T.);
#30555=ORIENTED_EDGE('',*,*,#21232,.T.);
#30556=ORIENTED_EDGE('',*,*,#21233,.F.);
#30557=ORIENTED_EDGE('',*,*,#21234,.T.);
#30558=ORIENTED_EDGE('',*,*,#21235,.T.);
#30559=ORIENTED_EDGE('',*,*,#21229,.F.);
#30560=ORIENTED_EDGE('',*,*,#21236,.T.);
#30561=ORIENTED_EDGE('',*,*,#21237,.T.);
#30562=ORIENTED_EDGE('',*,*,#21238,.F.);
#30563=ORIENTED_EDGE('',*,*,#21239,.T.);
#30564=ORIENTED_EDGE('',*,*,#21169,.T.);
#30565=ORIENTED_EDGE('',*,*,#21240,.T.);
#30566=ORIENTED_EDGE('',*,*,#21240,.F.);
#30567=ORIENTED_EDGE('',*,*,#21174,.T.);
#30568=ORIENTED_EDGE('',*,*,#21206,.T.);
#30569=ORIENTED_EDGE('',*,*,#21241,.T.);
#30570=ORIENTED_EDGE('',*,*,#21242,.T.);
#30571=ORIENTED_EDGE('',*,*,#21238,.T.);
#30572=ORIENTED_EDGE('',*,*,#21243,.F.);
#30573=ORIENTED_EDGE('',*,*,#21244,.F.);
#30574=ORIENTED_EDGE('',*,*,#21245,.T.);
#30575=ORIENTED_EDGE('',*,*,#21224,.T.);
#30576=ORIENTED_EDGE('',*,*,#21246,.F.);
#30577=ORIENTED_EDGE('',*,*,#21247,.F.);
#30578=ORIENTED_EDGE('',*,*,#21248,.T.);
#30579=ORIENTED_EDGE('',*,*,#21216,.T.);
#30580=ORIENTED_EDGE('',*,*,#21249,.F.);
#30581=ORIENTED_EDGE('',*,*,#21250,.F.);
#30582=ORIENTED_EDGE('',*,*,#21251,.T.);
#30583=ORIENTED_EDGE('',*,*,#21208,.T.);
#30584=ORIENTED_EDGE('',*,*,#21252,.F.);
#30585=ORIENTED_EDGE('',*,*,#21253,.F.);
#30586=ORIENTED_EDGE('',*,*,#21054,.T.);
#30587=ORIENTED_EDGE('',*,*,#21237,.F.);
#30588=ORIENTED_EDGE('',*,*,#21254,.T.);
#30589=ORIENTED_EDGE('',*,*,#21255,.T.);
#30590=ORIENTED_EDGE('',*,*,#21243,.T.);
#30591=ORIENTED_EDGE('',*,*,#21244,.T.);
#30592=ORIENTED_EDGE('',*,*,#21255,.F.);
#30593=ORIENTED_EDGE('',*,*,#21256,.F.);
#30594=ORIENTED_EDGE('',*,*,#21257,.T.);
#30595=ORIENTED_EDGE('',*,*,#21225,.F.);
#30596=ORIENTED_EDGE('',*,*,#21245,.F.);
#30597=ORIENTED_EDGE('',*,*,#21257,.F.);
#30598=ORIENTED_EDGE('',*,*,#21258,.T.);
#30599=ORIENTED_EDGE('',*,*,#21223,.F.);
#30600=ORIENTED_EDGE('',*,*,#21186,.T.);
#30601=ORIENTED_EDGE('',*,*,#21259,.T.);
#30602=ORIENTED_EDGE('',*,*,#21246,.T.);
#30603=ORIENTED_EDGE('',*,*,#21247,.T.);
#30604=ORIENTED_EDGE('',*,*,#21259,.F.);
#30605=ORIENTED_EDGE('',*,*,#21185,.F.);
#30606=ORIENTED_EDGE('',*,*,#21260,.T.);
#30607=ORIENTED_EDGE('',*,*,#21217,.F.);
#30608=ORIENTED_EDGE('',*,*,#21248,.F.);
#30609=ORIENTED_EDGE('',*,*,#21260,.F.);
#30610=ORIENTED_EDGE('',*,*,#21184,.T.);
#30611=ORIENTED_EDGE('',*,*,#21215,.F.);
#30612=ORIENTED_EDGE('',*,*,#21180,.T.);
#30613=ORIENTED_EDGE('',*,*,#21261,.T.);
#30614=ORIENTED_EDGE('',*,*,#21249,.T.);
#30615=ORIENTED_EDGE('',*,*,#21250,.T.);
#30616=ORIENTED_EDGE('',*,*,#21261,.F.);
#30617=ORIENTED_EDGE('',*,*,#21179,.F.);
#30618=ORIENTED_EDGE('',*,*,#21262,.T.);
#30619=ORIENTED_EDGE('',*,*,#21209,.F.);
#30620=ORIENTED_EDGE('',*,*,#21251,.F.);
#30621=ORIENTED_EDGE('',*,*,#21262,.F.);
#30622=ORIENTED_EDGE('',*,*,#21178,.T.);
#30623=ORIENTED_EDGE('',*,*,#21207,.F.);
#30624=ORIENTED_EDGE('',*,*,#21172,.T.);
#30625=ORIENTED_EDGE('',*,*,#21263,.T.);
#30626=ORIENTED_EDGE('',*,*,#21252,.T.);
#30627=ORIENTED_EDGE('',*,*,#21253,.T.);
#30628=ORIENTED_EDGE('',*,*,#21263,.F.);
#30629=ORIENTED_EDGE('',*,*,#21171,.F.);
#30630=ORIENTED_EDGE('',*,*,#21264,.T.);
#30631=ORIENTED_EDGE('',*,*,#21239,.F.);
#30632=ORIENTED_EDGE('',*,*,#21242,.F.);
#30633=ORIENTED_EDGE('',*,*,#21264,.F.);
#30634=ORIENTED_EDGE('',*,*,#21170,.T.);
#30635=ORIENTED_EDGE('',*,*,#21236,.F.);
#30636=ORIENTED_EDGE('',*,*,#21228,.F.);
#30637=ORIENTED_EDGE('',*,*,#21226,.F.);
#30638=ORIENTED_EDGE('',*,*,#21258,.F.);
#30639=ORIENTED_EDGE('',*,*,#21256,.T.);
#30640=ORIENTED_EDGE('',*,*,#21254,.F.);
#30641=ORIENTED_EDGE('',*,*,#21151,.T.);
#30642=ORIENTED_EDGE('',*,*,#21265,.T.);
#30643=ORIENTED_EDGE('',*,*,#21234,.F.);
#30644=ORIENTED_EDGE('',*,*,#21266,.F.);
#30645=ORIENTED_EDGE('',*,*,#21232,.F.);
#30646=ORIENTED_EDGE('',*,*,#21233,.T.);
#30647=ORIENTED_EDGE('',*,*,#21266,.T.);
#30648=ORIENTED_EDGE('',*,*,#21267,.T.);
#30649=ORIENTED_EDGE('',*,*,#21268,.F.);
#30650=ORIENTED_EDGE('',*,*,#21269,.F.);
#30651=ORIENTED_EDGE('',*,*,#21270,.T.);
#30652=ORIENTED_EDGE('',*,*,#21271,.T.);
#30653=ORIENTED_EDGE('',*,*,#21272,.F.);
#30654=ORIENTED_EDGE('',*,*,#21273,.F.);
#30655=ORIENTED_EDGE('',*,*,#21268,.T.);
#30656=ORIENTED_EDGE('',*,*,#21274,.T.);
#30657=ORIENTED_EDGE('',*,*,#21275,.F.);
#30658=ORIENTED_EDGE('',*,*,#21276,.F.);
#30659=ORIENTED_EDGE('',*,*,#21272,.T.);
#30660=ORIENTED_EDGE('',*,*,#21277,.F.);
#30661=ORIENTED_EDGE('',*,*,#21278,.F.);
#30662=ORIENTED_EDGE('',*,*,#21279,.T.);
#30663=ORIENTED_EDGE('',*,*,#21275,.T.);
#30664=ORIENTED_EDGE('',*,*,#21280,.T.);
#30665=ORIENTED_EDGE('',*,*,#21281,.F.);
#30666=ORIENTED_EDGE('',*,*,#21282,.F.);
#30667=ORIENTED_EDGE('',*,*,#21278,.T.);
#30668=ORIENTED_EDGE('',*,*,#21283,.T.);
#30669=ORIENTED_EDGE('',*,*,#21284,.F.);
#30670=ORIENTED_EDGE('',*,*,#21285,.F.);
#30671=ORIENTED_EDGE('',*,*,#21281,.T.);
#30672=ORIENTED_EDGE('',*,*,#21286,.T.);
#30673=ORIENTED_EDGE('',*,*,#21287,.F.);
#30674=ORIENTED_EDGE('',*,*,#21288,.F.);
#30675=ORIENTED_EDGE('',*,*,#21284,.T.);
#30676=ORIENTED_EDGE('',*,*,#21289,.T.);
#30677=ORIENTED_EDGE('',*,*,#21270,.F.);
#30678=ORIENTED_EDGE('',*,*,#21290,.F.);
#30679=ORIENTED_EDGE('',*,*,#21287,.T.);
#30680=ORIENTED_EDGE('',*,*,#21269,.T.);
#30681=ORIENTED_EDGE('',*,*,#21273,.T.);
#30682=ORIENTED_EDGE('',*,*,#21276,.T.);
#30683=ORIENTED_EDGE('',*,*,#21279,.F.);
#30684=ORIENTED_EDGE('',*,*,#21282,.T.);
#30685=ORIENTED_EDGE('',*,*,#21285,.T.);
#30686=ORIENTED_EDGE('',*,*,#21288,.T.);
#30687=ORIENTED_EDGE('',*,*,#21290,.T.);
#30688=ORIENTED_EDGE('',*,*,#21291,.T.);
#30689=ORIENTED_EDGE('',*,*,#21292,.F.);
#30690=ORIENTED_EDGE('',*,*,#21293,.F.);
#30691=ORIENTED_EDGE('',*,*,#21294,.T.);
#30692=ORIENTED_EDGE('',*,*,#21295,.T.);
#30693=ORIENTED_EDGE('',*,*,#21296,.F.);
#30694=ORIENTED_EDGE('',*,*,#21297,.F.);
#30695=ORIENTED_EDGE('',*,*,#21292,.T.);
#30696=ORIENTED_EDGE('',*,*,#21298,.F.);
#30697=ORIENTED_EDGE('',*,*,#21299,.F.);
#30698=ORIENTED_EDGE('',*,*,#21300,.T.);
#30699=ORIENTED_EDGE('',*,*,#21296,.T.);
#30700=ORIENTED_EDGE('',*,*,#21301,.T.);
#30701=ORIENTED_EDGE('',*,*,#21302,.F.);
#30702=ORIENTED_EDGE('',*,*,#21303,.F.);
#30703=ORIENTED_EDGE('',*,*,#21299,.T.);
#30704=ORIENTED_EDGE('',*,*,#21304,.T.);
#30705=ORIENTED_EDGE('',*,*,#21305,.F.);
#30706=ORIENTED_EDGE('',*,*,#21306,.F.);
#30707=ORIENTED_EDGE('',*,*,#21302,.T.);
#30708=ORIENTED_EDGE('',*,*,#21307,.T.);
#30709=ORIENTED_EDGE('',*,*,#21308,.F.);
#30710=ORIENTED_EDGE('',*,*,#21309,.F.);
#30711=ORIENTED_EDGE('',*,*,#21305,.T.);
#30712=ORIENTED_EDGE('',*,*,#21310,.T.);
#30713=ORIENTED_EDGE('',*,*,#21311,.F.);
#30714=ORIENTED_EDGE('',*,*,#21312,.F.);
#30715=ORIENTED_EDGE('',*,*,#21308,.T.);
#30716=ORIENTED_EDGE('',*,*,#21313,.T.);
#30717=ORIENTED_EDGE('',*,*,#21294,.F.);
#30718=ORIENTED_EDGE('',*,*,#21314,.F.);
#30719=ORIENTED_EDGE('',*,*,#21311,.T.);
#30720=ORIENTED_EDGE('',*,*,#21293,.T.);
#30721=ORIENTED_EDGE('',*,*,#21297,.T.);
#30722=ORIENTED_EDGE('',*,*,#21300,.F.);
#30723=ORIENTED_EDGE('',*,*,#21303,.T.);
#30724=ORIENTED_EDGE('',*,*,#21306,.T.);
#30725=ORIENTED_EDGE('',*,*,#21309,.T.);
#30726=ORIENTED_EDGE('',*,*,#21312,.T.);
#30727=ORIENTED_EDGE('',*,*,#21314,.T.);
#30728=ORIENTED_EDGE('',*,*,#21315,.T.);
#30729=ORIENTED_EDGE('',*,*,#21316,.F.);
#30730=ORIENTED_EDGE('',*,*,#21317,.F.);
#30731=ORIENTED_EDGE('',*,*,#21318,.T.);
#30732=ORIENTED_EDGE('',*,*,#21319,.T.);
#30733=ORIENTED_EDGE('',*,*,#21320,.F.);
#30734=ORIENTED_EDGE('',*,*,#21321,.F.);
#30735=ORIENTED_EDGE('',*,*,#21316,.T.);
#30736=ORIENTED_EDGE('',*,*,#21322,.T.);
#30737=ORIENTED_EDGE('',*,*,#21323,.F.);
#30738=ORIENTED_EDGE('',*,*,#21324,.F.);
#30739=ORIENTED_EDGE('',*,*,#21320,.T.);
#30740=ORIENTED_EDGE('',*,*,#21325,.T.);
#30741=ORIENTED_EDGE('',*,*,#21326,.F.);
#30742=ORIENTED_EDGE('',*,*,#21327,.F.);
#30743=ORIENTED_EDGE('',*,*,#21323,.T.);
#30744=ORIENTED_EDGE('',*,*,#21328,.F.);
#30745=ORIENTED_EDGE('',*,*,#21329,.F.);
#30746=ORIENTED_EDGE('',*,*,#21330,.T.);
#30747=ORIENTED_EDGE('',*,*,#21326,.T.);
#30748=ORIENTED_EDGE('',*,*,#21331,.T.);
#30749=ORIENTED_EDGE('',*,*,#21332,.F.);
#30750=ORIENTED_EDGE('',*,*,#21333,.F.);
#30751=ORIENTED_EDGE('',*,*,#21329,.T.);
#30752=ORIENTED_EDGE('',*,*,#21334,.T.);
#30753=ORIENTED_EDGE('',*,*,#21335,.F.);
#30754=ORIENTED_EDGE('',*,*,#21336,.F.);
#30755=ORIENTED_EDGE('',*,*,#21332,.T.);
#30756=ORIENTED_EDGE('',*,*,#21337,.T.);
#30757=ORIENTED_EDGE('',*,*,#21318,.F.);
#30758=ORIENTED_EDGE('',*,*,#21338,.F.);
#30759=ORIENTED_EDGE('',*,*,#21335,.T.);
#30760=ORIENTED_EDGE('',*,*,#21317,.T.);
#30761=ORIENTED_EDGE('',*,*,#21321,.T.);
#30762=ORIENTED_EDGE('',*,*,#21324,.T.);
#30763=ORIENTED_EDGE('',*,*,#21327,.T.);
#30764=ORIENTED_EDGE('',*,*,#21330,.F.);
#30765=ORIENTED_EDGE('',*,*,#21333,.T.);
#30766=ORIENTED_EDGE('',*,*,#21336,.T.);
#30767=ORIENTED_EDGE('',*,*,#21338,.T.);
#30768=ORIENTED_EDGE('',*,*,#21339,.T.);
#30769=ORIENTED_EDGE('',*,*,#21340,.F.);
#30770=ORIENTED_EDGE('',*,*,#21341,.F.);
#30771=ORIENTED_EDGE('',*,*,#21342,.T.);
#30772=ORIENTED_EDGE('',*,*,#21343,.T.);
#30773=ORIENTED_EDGE('',*,*,#21344,.F.);
#30774=ORIENTED_EDGE('',*,*,#21345,.F.);
#30775=ORIENTED_EDGE('',*,*,#21340,.T.);
#30776=ORIENTED_EDGE('',*,*,#21346,.T.);
#30777=ORIENTED_EDGE('',*,*,#21347,.F.);
#30778=ORIENTED_EDGE('',*,*,#21348,.F.);
#30779=ORIENTED_EDGE('',*,*,#21344,.T.);
#30780=ORIENTED_EDGE('',*,*,#21349,.T.);
#30781=ORIENTED_EDGE('',*,*,#21350,.F.);
#30782=ORIENTED_EDGE('',*,*,#21351,.F.);
#30783=ORIENTED_EDGE('',*,*,#21347,.T.);
#30784=ORIENTED_EDGE('',*,*,#21352,.F.);
#30785=ORIENTED_EDGE('',*,*,#21353,.F.);
#30786=ORIENTED_EDGE('',*,*,#21354,.T.);
#30787=ORIENTED_EDGE('',*,*,#21350,.T.);
#30788=ORIENTED_EDGE('',*,*,#21355,.T.);
#30789=ORIENTED_EDGE('',*,*,#21356,.F.);
#30790=ORIENTED_EDGE('',*,*,#21357,.F.);
#30791=ORIENTED_EDGE('',*,*,#21353,.T.);
#30792=ORIENTED_EDGE('',*,*,#21358,.T.);
#30793=ORIENTED_EDGE('',*,*,#21359,.F.);
#30794=ORIENTED_EDGE('',*,*,#21360,.F.);
#30795=ORIENTED_EDGE('',*,*,#21356,.T.);
#30796=ORIENTED_EDGE('',*,*,#21361,.T.);
#30797=ORIENTED_EDGE('',*,*,#21342,.F.);
#30798=ORIENTED_EDGE('',*,*,#21362,.F.);
#30799=ORIENTED_EDGE('',*,*,#21359,.T.);
#30800=ORIENTED_EDGE('',*,*,#21341,.T.);
#30801=ORIENTED_EDGE('',*,*,#21345,.T.);
#30802=ORIENTED_EDGE('',*,*,#21348,.T.);
#30803=ORIENTED_EDGE('',*,*,#21351,.T.);
#30804=ORIENTED_EDGE('',*,*,#21354,.F.);
#30805=ORIENTED_EDGE('',*,*,#21357,.T.);
#30806=ORIENTED_EDGE('',*,*,#21360,.T.);
#30807=ORIENTED_EDGE('',*,*,#21362,.T.);
#30808=ORIENTED_EDGE('',*,*,#21363,.F.);
#30809=ORIENTED_EDGE('',*,*,#21364,.F.);
#30810=ORIENTED_EDGE('',*,*,#21068,.T.);
#30811=ORIENTED_EDGE('',*,*,#21365,.T.);
#30812=ORIENTED_EDGE('',*,*,#21366,.T.);
#30813=ORIENTED_EDGE('',*,*,#21365,.F.);
#30814=ORIENTED_EDGE('',*,*,#21075,.F.);
#30815=ORIENTED_EDGE('',*,*,#21367,.T.);
#30816=ORIENTED_EDGE('',*,*,#21368,.T.);
#30817=ORIENTED_EDGE('',*,*,#21367,.F.);
#30818=ORIENTED_EDGE('',*,*,#21074,.F.);
#30819=ORIENTED_EDGE('',*,*,#21369,.T.);
#30820=ORIENTED_EDGE('',*,*,#21370,.T.);
#30821=ORIENTED_EDGE('',*,*,#21369,.F.);
#30822=ORIENTED_EDGE('',*,*,#21073,.F.);
#30823=ORIENTED_EDGE('',*,*,#21371,.T.);
#30824=ORIENTED_EDGE('',*,*,#21372,.T.);
#30825=ORIENTED_EDGE('',*,*,#21371,.F.);
#30826=ORIENTED_EDGE('',*,*,#21072,.F.);
#30827=ORIENTED_EDGE('',*,*,#21373,.T.);
#30828=ORIENTED_EDGE('',*,*,#21374,.T.);
#30829=ORIENTED_EDGE('',*,*,#21373,.F.);
#30830=ORIENTED_EDGE('',*,*,#21071,.F.);
#30831=ORIENTED_EDGE('',*,*,#21375,.T.);
#30832=ORIENTED_EDGE('',*,*,#21376,.T.);
#30833=ORIENTED_EDGE('',*,*,#21377,.F.);
#30834=ORIENTED_EDGE('',*,*,#21069,.F.);
#30835=ORIENTED_EDGE('',*,*,#21364,.T.);
#30836=ORIENTED_EDGE('',*,*,#21378,.T.);
#30837=ORIENTED_EDGE('',*,*,#21375,.F.);
#30838=ORIENTED_EDGE('',*,*,#21070,.F.);
#30839=ORIENTED_EDGE('',*,*,#21377,.T.);
#30840=ORIENTED_EDGE('',*,*,#21191,.F.);
#30841=ORIENTED_EDGE('',*,*,#21379,.T.);
#30842=ORIENTED_EDGE('',*,*,#21380,.T.);
#30843=ORIENTED_EDGE('',*,*,#21379,.F.);
#30844=ORIENTED_EDGE('',*,*,#21190,.F.);
#30845=ORIENTED_EDGE('',*,*,#21380,.F.);
#30846=ORIENTED_EDGE('',*,*,#21050,.T.);
#30847=ORIENTED_EDGE('',*,*,#21053,.T.);
#30848=ORIENTED_EDGE('',*,*,#21058,.T.);
#30849=ORIENTED_EDGE('',*,*,#21061,.T.);
#30850=ORIENTED_EDGE('',*,*,#21064,.T.);
#30851=ORIENTED_EDGE('',*,*,#21067,.T.);
#30852=ORIENTED_EDGE('',*,*,#21381,.T.);
#30853=ORIENTED_EDGE('',*,*,#21382,.T.);
#30854=ORIENTED_EDGE('',*,*,#21383,.T.);
#30855=ORIENTED_EDGE('',*,*,#21384,.T.);
#30856=ORIENTED_EDGE('',*,*,#21385,.T.);
#30857=ORIENTED_EDGE('',*,*,#21386,.T.);
#30858=ORIENTED_EDGE('',*,*,#21387,.T.);
#30859=ORIENTED_EDGE('',*,*,#21388,.T.);
#30860=ORIENTED_EDGE('',*,*,#21194,.F.);
#30861=ORIENTED_EDGE('',*,*,#21389,.F.);
#30862=ORIENTED_EDGE('',*,*,#21388,.F.);
#30863=ORIENTED_EDGE('',*,*,#21390,.T.);
#30864=ORIENTED_EDGE('',*,*,#21196,.F.);
#30865=ORIENTED_EDGE('',*,*,#21391,.F.);
#30866=ORIENTED_EDGE('',*,*,#21386,.F.);
#30867=ORIENTED_EDGE('',*,*,#21392,.T.);
#30868=ORIENTED_EDGE('',*,*,#21195,.F.);
#30869=ORIENTED_EDGE('',*,*,#20769,.F.);
#30870=ORIENTED_EDGE('',*,*,#21192,.F.);
#30871=ORIENTED_EDGE('',*,*,#21390,.F.);
#30872=ORIENTED_EDGE('',*,*,#21387,.F.);
#30873=ORIENTED_EDGE('',*,*,#21391,.T.);
#30874=ORIENTED_EDGE('',*,*,#21201,.F.);
#30875=ORIENTED_EDGE('',*,*,#21393,.F.);
#30876=ORIENTED_EDGE('',*,*,#21383,.F.);
#30877=ORIENTED_EDGE('',*,*,#21394,.T.);
#30878=ORIENTED_EDGE('',*,*,#21199,.F.);
#30879=ORIENTED_EDGE('',*,*,#20773,.F.);
#30880=ORIENTED_EDGE('',*,*,#21200,.F.);
#30881=ORIENTED_EDGE('',*,*,#21394,.F.);
#30882=ORIENTED_EDGE('',*,*,#21382,.F.);
#30883=ORIENTED_EDGE('',*,*,#21395,.T.);
#30884=ORIENTED_EDGE('',*,*,#21188,.T.);
#30885=ORIENTED_EDGE('',*,*,#21376,.F.);
#30886=ORIENTED_EDGE('',*,*,#21363,.T.);
#30887=ORIENTED_EDGE('',*,*,#21366,.F.);
#30888=ORIENTED_EDGE('',*,*,#21368,.F.);
#30889=ORIENTED_EDGE('',*,*,#21370,.F.);
#30890=ORIENTED_EDGE('',*,*,#21372,.F.);
#30891=ORIENTED_EDGE('',*,*,#21374,.F.);
#30892=ORIENTED_EDGE('',*,*,#21378,.F.);
#30893=ORIENTED_EDGE('',*,*,#21165,.F.);
#30894=ORIENTED_EDGE('',*,*,#21204,.F.);
#30895=ORIENTED_EDGE('',*,*,#21212,.F.);
#30896=ORIENTED_EDGE('',*,*,#21214,.F.);
#30897=ORIENTED_EDGE('',*,*,#21159,.F.);
#30898=ORIENTED_EDGE('',*,*,#21213,.F.);
#30899=ORIENTED_EDGE('',*,*,#21220,.F.);
#30900=ORIENTED_EDGE('',*,*,#21222,.F.);
#30901=ORIENTED_EDGE('',*,*,#21154,.F.);
#30902=ORIENTED_EDGE('',*,*,#21221,.F.);
#30903=ORIENTED_EDGE('',*,*,#21230,.F.);
#30904=ORIENTED_EDGE('',*,*,#21235,.F.);
#30905=ORIENTED_EDGE('',*,*,#21265,.F.);
#30906=ORIENTED_EDGE('',*,*,#21231,.F.);
#30907=ORIENTED_EDGE('',*,*,#21241,.F.);
#30908=ORIENTED_EDGE('',*,*,#21205,.F.);
#30909=ORIENTED_EDGE('',*,*,#21048,.F.);
#30910=ORIENTED_EDGE('',*,*,#21051,.F.);
#30911=ORIENTED_EDGE('',*,*,#21056,.F.);
#30912=ORIENTED_EDGE('',*,*,#21059,.F.);
#30913=ORIENTED_EDGE('',*,*,#21062,.F.);
#30914=ORIENTED_EDGE('',*,*,#21065,.F.);
#30915=ORIENTED_EDGE('',*,*,#21124,.F.);
#30916=ORIENTED_EDGE('',*,*,#21146,.F.);
#30917=ORIENTED_EDGE('',*,*,#21143,.T.);
#30918=ORIENTED_EDGE('',*,*,#21140,.F.);
#30919=ORIENTED_EDGE('',*,*,#21137,.F.);
#30920=ORIENTED_EDGE('',*,*,#21134,.F.);
#30921=ORIENTED_EDGE('',*,*,#21131,.F.);
#30922=ORIENTED_EDGE('',*,*,#21128,.F.);
#30923=ORIENTED_EDGE('',*,*,#21100,.F.);
#30924=ORIENTED_EDGE('',*,*,#21122,.F.);
#30925=ORIENTED_EDGE('',*,*,#21119,.T.);
#30926=ORIENTED_EDGE('',*,*,#21116,.F.);
#30927=ORIENTED_EDGE('',*,*,#21113,.F.);
#30928=ORIENTED_EDGE('',*,*,#21110,.F.);
#30929=ORIENTED_EDGE('',*,*,#21107,.F.);
#30930=ORIENTED_EDGE('',*,*,#21104,.F.);
#30931=ORIENTED_EDGE('',*,*,#21076,.F.);
#30932=ORIENTED_EDGE('',*,*,#21098,.F.);
#30933=ORIENTED_EDGE('',*,*,#21095,.T.);
#30934=ORIENTED_EDGE('',*,*,#21092,.F.);
#30935=ORIENTED_EDGE('',*,*,#21089,.F.);
#30936=ORIENTED_EDGE('',*,*,#21086,.F.);
#30937=ORIENTED_EDGE('',*,*,#21083,.F.);
#30938=ORIENTED_EDGE('',*,*,#21080,.F.);
#30939=ORIENTED_EDGE('',*,*,#21339,.F.);
#30940=ORIENTED_EDGE('',*,*,#21361,.F.);
#30941=ORIENTED_EDGE('',*,*,#21358,.F.);
#30942=ORIENTED_EDGE('',*,*,#21355,.F.);
#30943=ORIENTED_EDGE('',*,*,#21352,.T.);
#30944=ORIENTED_EDGE('',*,*,#21349,.F.);
#30945=ORIENTED_EDGE('',*,*,#21346,.F.);
#30946=ORIENTED_EDGE('',*,*,#21343,.F.);
#30947=ORIENTED_EDGE('',*,*,#21315,.F.);
#30948=ORIENTED_EDGE('',*,*,#21337,.F.);
#30949=ORIENTED_EDGE('',*,*,#21334,.F.);
#30950=ORIENTED_EDGE('',*,*,#21331,.F.);
#30951=ORIENTED_EDGE('',*,*,#21328,.T.);
#30952=ORIENTED_EDGE('',*,*,#21325,.F.);
#30953=ORIENTED_EDGE('',*,*,#21322,.F.);
#30954=ORIENTED_EDGE('',*,*,#21319,.F.);
#30955=ORIENTED_EDGE('',*,*,#21291,.F.);
#30956=ORIENTED_EDGE('',*,*,#21313,.F.);
#30957=ORIENTED_EDGE('',*,*,#21310,.F.);
#30958=ORIENTED_EDGE('',*,*,#21307,.F.);
#30959=ORIENTED_EDGE('',*,*,#21304,.F.);
#30960=ORIENTED_EDGE('',*,*,#21301,.F.);
#30961=ORIENTED_EDGE('',*,*,#21298,.T.);
#30962=ORIENTED_EDGE('',*,*,#21295,.F.);
#30963=ORIENTED_EDGE('',*,*,#21267,.F.);
#30964=ORIENTED_EDGE('',*,*,#21289,.F.);
#30965=ORIENTED_EDGE('',*,*,#21286,.F.);
#30966=ORIENTED_EDGE('',*,*,#21283,.F.);
#30967=ORIENTED_EDGE('',*,*,#21280,.F.);
#30968=ORIENTED_EDGE('',*,*,#21277,.T.);
#30969=ORIENTED_EDGE('',*,*,#21274,.F.);
#30970=ORIENTED_EDGE('',*,*,#21271,.F.);
#30971=ORIENTED_EDGE('',*,*,#21202,.F.);
#30972=ORIENTED_EDGE('',*,*,#20771,.F.);
#30973=ORIENTED_EDGE('',*,*,#21197,.F.);
#30974=ORIENTED_EDGE('',*,*,#21392,.F.);
#30975=ORIENTED_EDGE('',*,*,#21385,.F.);
#30976=ORIENTED_EDGE('',*,*,#21396,.T.);
#30977=ORIENTED_EDGE('',*,*,#21198,.F.);
#30978=ORIENTED_EDGE('',*,*,#21395,.F.);
#30979=ORIENTED_EDGE('',*,*,#21381,.F.);
#30980=ORIENTED_EDGE('',*,*,#21389,.T.);
#30981=ORIENTED_EDGE('',*,*,#21193,.F.);
#30982=ORIENTED_EDGE('',*,*,#20775,.F.);
#30983=ORIENTED_EDGE('',*,*,#21203,.F.);
#30984=ORIENTED_EDGE('',*,*,#21396,.F.);
#30985=ORIENTED_EDGE('',*,*,#21384,.F.);
#30986=ORIENTED_EDGE('',*,*,#21393,.T.);
#30987=ORIENTED_EDGE('',*,*,#20807,.T.);
#30988=ORIENTED_EDGE('',*,*,#20486,.F.);
#30989=ORIENTED_EDGE('',*,*,#21397,.F.);
#30990=ORIENTED_EDGE('',*,*,#21398,.F.);
#30991=ORIENTED_EDGE('',*,*,#21399,.T.);
#30992=ORIENTED_EDGE('',*,*,#21400,.T.);
#30993=ORIENTED_EDGE('',*,*,#21399,.F.);
#30994=ORIENTED_EDGE('',*,*,#21397,.T.);
#30995=ORIENTED_EDGE('',*,*,#21398,.T.);
#30996=ORIENTED_EDGE('',*,*,#21401,.T.);
#30997=ORIENTED_EDGE('',*,*,#21402,.F.);
#30998=ORIENTED_EDGE('',*,*,#21403,.F.);
#30999=ORIENTED_EDGE('',*,*,#21401,.F.);
#31000=ORIENTED_EDGE('',*,*,#21403,.T.);
#31001=ORIENTED_EDGE('',*,*,#21404,.T.);
#31002=ORIENTED_EDGE('',*,*,#21187,.F.);
#31003=ORIENTED_EDGE('',*,*,#21404,.F.);
#31004=ORIENTED_EDGE('',*,*,#21402,.T.);
#31005=ORIENTED_EDGE('',*,*,#21405,.T.);
#31006=ORIENTED_EDGE('',*,*,#21406,.F.);
#31007=ORIENTED_EDGE('',*,*,#21407,.F.);
#31008=ORIENTED_EDGE('',*,*,#21408,.T.);
#31009=ORIENTED_EDGE('',*,*,#21409,.T.);
#31010=ORIENTED_EDGE('',*,*,#21410,.F.);
#31011=ORIENTED_EDGE('',*,*,#21411,.F.);
#31012=ORIENTED_EDGE('',*,*,#21406,.T.);
#31013=ORIENTED_EDGE('',*,*,#21412,.T.);
#31014=ORIENTED_EDGE('',*,*,#21413,.F.);
#31015=ORIENTED_EDGE('',*,*,#21414,.F.);
#31016=ORIENTED_EDGE('',*,*,#21410,.T.);
#31017=ORIENTED_EDGE('',*,*,#21413,.T.);
#31018=ORIENTED_EDGE('',*,*,#21415,.F.);
#31019=ORIENTED_EDGE('',*,*,#21416,.F.);
#31020=ORIENTED_EDGE('',*,*,#21417,.F.);
#31021=ORIENTED_EDGE('',*,*,#21418,.T.);
#31022=ORIENTED_EDGE('',*,*,#21419,.F.);
#31023=ORIENTED_EDGE('',*,*,#21420,.F.);
#31024=ORIENTED_EDGE('',*,*,#21416,.T.);
#31025=ORIENTED_EDGE('',*,*,#21407,.T.);
#31026=ORIENTED_EDGE('',*,*,#21411,.T.);
#31027=ORIENTED_EDGE('',*,*,#21414,.T.);
#31028=ORIENTED_EDGE('',*,*,#21417,.T.);
#31029=ORIENTED_EDGE('',*,*,#21420,.T.);
#31030=ORIENTED_EDGE('',*,*,#21421,.T.);
#31031=ORIENTED_EDGE('',*,*,#21422,.T.);
#31032=ORIENTED_EDGE('',*,*,#21408,.F.);
#31033=ORIENTED_EDGE('',*,*,#21421,.F.);
#31034=ORIENTED_EDGE('',*,*,#21419,.T.);
#31035=ORIENTED_EDGE('',*,*,#21400,.F.);
#31036=ORIENTED_EDGE('',*,*,#21412,.F.);
#31037=ORIENTED_EDGE('',*,*,#21409,.F.);
#31038=ORIENTED_EDGE('',*,*,#21405,.F.);
#31039=ORIENTED_EDGE('',*,*,#21422,.F.);
#31040=ORIENTED_EDGE('',*,*,#21418,.F.);
#31041=ORIENTED_EDGE('',*,*,#21415,.T.);
#31669=PLANE('',#37252);
#31670=PLANE('',#37260);
#31671=PLANE('',#37262);
#31672=PLANE('',#37269);
#31673=PLANE('',#37277);
#31674=PLANE('',#37279);
#31675=PLANE('',#37286);
#31676=PLANE('',#37294);
#31677=PLANE('',#37298);
#31678=PLANE('',#37302);
#31679=PLANE('',#37306);
#31680=PLANE('',#37311);
#31681=PLANE('',#37319);
#31682=PLANE('',#37323);
#31683=PLANE('',#37328);
#31684=PLANE('',#37333);
#31685=PLANE('',#37337);
#31686=PLANE('',#37341);
#31687=PLANE('',#37342);
#31688=PLANE('',#37343);
#31689=PLANE('',#37345);
#31690=PLANE('',#37347);
#31691=PLANE('',#37348);
#31692=PLANE('',#37358);
#31693=PLANE('',#37360);
#31694=PLANE('',#37367);
#31695=PLANE('',#37369);
#31696=PLANE('',#37375);
#31697=PLANE('',#37376);
#31698=PLANE('',#37380);
#31699=PLANE('',#37383);
#31700=PLANE('',#37398);
#31701=PLANE('',#37399);
#31702=PLANE('',#37400);
#31703=PLANE('',#37401);
#31704=PLANE('',#37402);
#31705=PLANE('',#37403);
#31706=PLANE('',#37406);
#31707=PLANE('',#37424);
#31708=PLANE('',#37425);
#31709=PLANE('',#37426);
#31710=PLANE('',#37427);
#31711=PLANE('',#37430);
#31712=PLANE('',#37435);
#31713=PLANE('',#37436);
#31714=PLANE('',#37437);
#31715=PLANE('',#37438);
#31716=PLANE('',#37439);
#31717=PLANE('',#37450);
#31718=PLANE('',#37451);
#31719=PLANE('',#37454);
#31720=PLANE('',#37455);
#31721=PLANE('',#37456);
#31722=PLANE('',#37457);
#31723=PLANE('',#37458);
#31724=PLANE('',#37469);
#31725=PLANE('',#37470);
#31726=PLANE('',#37473);
#31727=PLANE('',#37474);
#31728=PLANE('',#37475);
#31729=PLANE('',#37476);
#31730=PLANE('',#37477);
#31731=PLANE('',#37478);
#31732=PLANE('',#37479);
#31733=PLANE('',#37480);
#31734=PLANE('',#37481);
#31735=PLANE('',#37483);
#31736=PLANE('',#37490);
#31737=PLANE('',#37491);
#31738=PLANE('',#37492);
#31739=PLANE('',#37493);
#31740=PLANE('',#37494);
#31741=PLANE('',#37495);
#31742=PLANE('',#37496);
#31743=PLANE('',#37499);
#31744=PLANE('',#37500);
#31745=PLANE('',#37501);
#31746=PLANE('',#37502);
#31747=PLANE('',#37503);
#31748=PLANE('',#37504);
#31749=PLANE('',#37505);
#31750=PLANE('',#37506);
#31751=PLANE('',#37509);
#31752=PLANE('',#37510);
#31753=PLANE('',#37511);
#31754=PLANE('',#37512);
#31755=PLANE('',#37513);
#31756=PLANE('',#37580);
#31757=PLANE('',#37581);
#31758=PLANE('',#37582);
#31759=PLANE('',#37583);
#31760=PLANE('',#37584);
#31761=PLANE('',#37585);
#31762=PLANE('',#37586);
#31763=PLANE('',#37587);
#31764=PLANE('',#37588);
#31765=PLANE('',#37589);
#31766=PLANE('',#37598);
#31767=PLANE('',#37599);
#31768=PLANE('',#37600);
#31769=PLANE('',#37601);
#31770=PLANE('',#37602);
#31771=PLANE('',#37603);
#31772=PLANE('',#37604);
#31773=PLANE('',#37605);
#31774=PLANE('',#37606);
#31775=PLANE('',#37607);
#31776=PLANE('',#37608);
#31777=PLANE('',#37627);
#31778=PLANE('',#37628);
#31779=PLANE('',#37632);
#31780=PLANE('',#37641);
#31781=PLANE('',#37645);
#31782=PLANE('',#37653);
#31783=PLANE('',#37654);
#31784=PLANE('',#37655);
#31785=PLANE('',#37656);
#31786=PLANE('',#37657);
#31787=PLANE('',#37658);
#31788=PLANE('',#37659);
#31789=PLANE('',#37660);
#31790=PLANE('',#37661);
#31791=PLANE('',#37662);
#31792=PLANE('',#37663);
#31793=PLANE('',#37664);
#31794=PLANE('',#37665);
#31795=PLANE('',#37666);
#31796=PLANE('',#37667);
#31797=PLANE('',#37668);
#31798=PLANE('',#37678);
#31799=PLANE('',#37679);
#31800=PLANE('',#37684);
#31801=PLANE('',#37685);
#31802=PLANE('',#37686);
#31803=PLANE('',#37687);
#31804=PLANE('',#37688);
#31805=PLANE('',#37689);
#31806=PLANE('',#37690);
#31807=PLANE('',#37691);
#31808=PLANE('',#37692);
#31809=PLANE('',#37693);
#31810=PLANE('',#37694);
#31811=PLANE('',#37695);
#31812=PLANE('',#37696);
#31813=PLANE('',#37697);
#31814=PLANE('',#37698);
#31815=PLANE('',#37708);
#31816=PLANE('',#37709);
#31817=PLANE('',#37717);
#31818=PLANE('',#37720);
#31819=PLANE('',#37729);
#31820=PLANE('',#37731);
#31821=PLANE('',#37734);
#31822=PLANE('',#37736);
#31823=PLANE('',#37741);
#31824=PLANE('',#37742);
#31825=PLANE('',#37745);
#31826=PLANE('',#37753);
#31827=PLANE('',#37754);
#31828=PLANE('',#37760);
#31829=PLANE('',#37761);
#31830=PLANE('',#37762);
#31831=PLANE('',#37763);
#31832=PLANE('',#37764);
#31833=PLANE('',#37772);
#31834=PLANE('',#37773);
#31835=PLANE('',#37779);
#31836=PLANE('',#37780);
#31837=PLANE('',#37781);
#31838=PLANE('',#37782);
#31839=PLANE('',#37783);
#31840=PLANE('',#37785);
#31841=PLANE('',#37787);
#31842=PLANE('',#37809);
#31843=PLANE('',#37816);
#31844=PLANE('',#37826);
#31845=PLANE('',#37836);
#31846=PLANE('',#37837);
#31847=PLANE('',#37847);
#31848=PLANE('',#37857);
#31849=PLANE('',#37858);
#31850=PLANE('',#37868);
#31851=PLANE('',#37878);
#31852=PLANE('',#37890);
#31853=PLANE('',#37896);
#31854=PLANE('',#37902);
#31855=PLANE('',#37903);
#31856=PLANE('',#37906);
#31857=PLANE('',#37909);
#31858=PLANE('',#37917);
#31859=PLANE('',#37918);
#31860=PLANE('',#37919);
#31861=PLANE('',#37920);
#31862=PLANE('',#37921);
#31863=PLANE('',#37924);
#31864=PLANE('',#37927);
#31865=PLANE('',#37931);
#31866=PLANE('',#37936);
#31867=PLANE('',#37941);
#31868=PLANE('',#37944);
#31869=PLANE('',#37945);
#31870=PLANE('',#37947);
#31871=PLANE('',#37948);
#31872=PLANE('',#37950);
#31873=PLANE('',#37951);
#31874=PLANE('',#37953);
#31875=PLANE('',#37954);
#31876=PLANE('',#37958);
#31877=PLANE('',#37962);
#31878=PLANE('',#37972);
#31879=PLANE('',#37979);
#31880=PLANE('',#37980);
#31881=PLANE('',#37990);
#31882=PLANE('',#38000);
#31883=PLANE('',#38007);
#31884=PLANE('',#38017);
#31885=PLANE('',#38021);
#31886=PLANE('',#38028);
#31887=PLANE('',#38038);
#31888=PLANE('',#38042);
#31889=PLANE('',#38047);
#31890=PLANE('',#38056);
#31891=PLANE('',#38060);
#31892=PLANE('',#38061);
#31893=PLANE('',#38062);
#31894=PLANE('',#38063);
#31895=PLANE('',#38064);
#31896=PLANE('',#38065);
#31897=PLANE('',#38066);
#31898=PLANE('',#38067);
#31899=PLANE('',#38068);
#31900=PLANE('',#38069);
#31901=PLANE('',#38070);
#31902=PLANE('',#38079);
#31903=PLANE('',#38080);
#31904=PLANE('',#38081);
#31905=PLANE('',#38082);
#31906=PLANE('',#38083);
#31907=PLANE('',#38084);
#31908=PLANE('',#38085);
#31909=PLANE('',#38086);
#33325=ADVANCED_FACE('',(#5644),#616,.T.);
#33326=ADVANCED_FACE('',(#5645),#31669,.T.);
#33327=ADVANCED_FACE('',(#5646),#617,.F.);
#33328=ADVANCED_FACE('',(#5647),#1751,.F.);
#33329=ADVANCED_FACE('',(#5648),#1752,.T.);
#33330=ADVANCED_FACE('',(#5649,#2137),#31670,.T.);
#33331=ADVANCED_FACE('',(#5650,#2138),#31671,.T.);
#33332=ADVANCED_FACE('',(#5651),#1753,.F.);
#33333=ADVANCED_FACE('',(#5652),#618,.T.);
#33334=ADVANCED_FACE('',(#5653),#31672,.T.);
#33335=ADVANCED_FACE('',(#5654),#619,.F.);
#33336=ADVANCED_FACE('',(#5655),#1754,.F.);
#33337=ADVANCED_FACE('',(#5656),#1755,.T.);
#33338=ADVANCED_FACE('',(#5657,#2139),#31673,.T.);
#33339=ADVANCED_FACE('',(#5658,#2140),#31674,.T.);
#33340=ADVANCED_FACE('',(#5659),#1756,.F.);
#33341=ADVANCED_FACE('',(#5660),#620,.T.);
#33342=ADVANCED_FACE('',(#5661),#31675,.T.);
#33343=ADVANCED_FACE('',(#5662),#1757,.F.);
#33344=ADVANCED_FACE('',(#5663),#621,.F.);
#33345=ADVANCED_FACE('',(#5664),#1758,.T.);
#33346=ADVANCED_FACE('',(#5665,#2141),#31676,.T.);
#33347=ADVANCED_FACE('',(#5666),#1759,.F.);
#33348=ADVANCED_FACE('',(#5667,#2142),#31677,.T.);
#33349=ADVANCED_FACE('',(#5668),#1760,.T.);
#33350=ADVANCED_FACE('',(#5669,#2143),#31678,.T.);
#33351=ADVANCED_FACE('',(#5670),#1761,.F.);
#33352=ADVANCED_FACE('',(#5671,#2144),#31679,.T.);
#33353=ADVANCED_FACE('',(#5672),#622,.T.);
#33354=ADVANCED_FACE('',(#5673),#31680,.T.);
#33355=ADVANCED_FACE('',(#5674),#1762,.F.);
#33356=ADVANCED_FACE('',(#5675),#623,.F.);
#33357=ADVANCED_FACE('',(#5676),#1763,.T.);
#33358=ADVANCED_FACE('',(#5677,#2145),#31681,.T.);
#33359=ADVANCED_FACE('',(#5678),#1764,.F.);
#33360=ADVANCED_FACE('',(#5679,#2146),#31682,.T.);
#33361=ADVANCED_FACE('',(#5680),#624,.T.);
#33362=ADVANCED_FACE('',(#5681),#31683,.T.);
#33363=ADVANCED_FACE('',(#5682),#1765,.F.);
#33364=ADVANCED_FACE('',(#5683),#625,.F.);
#33365=ADVANCED_FACE('',(#5684),#31684,.T.);
#33366=ADVANCED_FACE('',(#5685),#626,.T.);
#33367=ADVANCED_FACE('',(#5686),#31685,.T.);
#33368=ADVANCED_FACE('',(#5687),#627,.T.);
#33369=ADVANCED_FACE('',(#5688),#31686,.T.);
#33370=ADVANCED_FACE('',(#5689),#31687,.T.);
#33371=ADVANCED_FACE('',(#5690),#31688,.T.);
#33372=ADVANCED_FACE('',(#5691),#31689,.T.);
#33373=ADVANCED_FACE('',(#5692),#31690,.T.);
#33374=ADVANCED_FACE('',(#5693,#2147),#31691,.T.);
#33375=ADVANCED_FACE('',(#5694),#1766,.F.);
#33376=ADVANCED_FACE('',(#5695),#31692,.T.);
#33377=ADVANCED_FACE('',(#5696,#2148,#2149,#2150,#2151),#31693,.T.);
#33378=ADVANCED_FACE('',(#5697),#1767,.F.);
#33379=ADVANCED_FACE('',(#5698),#31694,.T.);
#33380=ADVANCED_FACE('',(#5699),#31695,.T.);
#33381=ADVANCED_FACE('',(#5700),#1768,.F.);
#33382=ADVANCED_FACE('',(#5701),#31696,.T.);
#33383=ADVANCED_FACE('',(#5702),#31697,.T.);
#33384=ADVANCED_FACE('',(#5703),#1769,.F.);
#33385=ADVANCED_FACE('',(#5704),#31698,.T.);
#33386=ADVANCED_FACE('',(#5705),#31699,.T.);
#33387=ADVANCED_FACE('',(#5706),#1770,.F.);
#33388=ADVANCED_FACE('',(#5707),#1771,.T.);
#33389=ADVANCED_FACE('',(#5708),#31700,.T.);
#33390=ADVANCED_FACE('',(#5709),#31701,.T.);
#33391=ADVANCED_FACE('',(#5710),#31702,.T.);
#33392=ADVANCED_FACE('',(#5711),#31703,.T.);
#33393=ADVANCED_FACE('',(#5712),#31704,.T.);
#33394=ADVANCED_FACE('',(#5713),#31705,.T.);
#33395=ADVANCED_FACE('',(#5714),#628,.T.);
#33396=ADVANCED_FACE('',(#5715,#2152),#31706,.T.);
#33397=ADVANCED_FACE('',(#5716),#1772,.F.);
#33398=ADVANCED_FACE('',(#5717),#1773,.F.);
#33399=ADVANCED_FACE('',(#5718),#1774,.F.);
#33400=ADVANCED_FACE('',(#5719),#1775,.F.);
#33401=ADVANCED_FACE('',(#5720),#31707,.T.);
#33402=ADVANCED_FACE('',(#5721),#31708,.T.);
#33403=ADVANCED_FACE('',(#5722),#31709,.T.);
#33404=ADVANCED_FACE('',(#5723,#2153),#31710,.T.);
#33405=ADVANCED_FACE('',(#5724),#31711,.T.);
#33406=ADVANCED_FACE('',(#5725),#1776,.T.);
#33407=ADVANCED_FACE('',(#5726),#31712,.T.);
#33408=ADVANCED_FACE('',(#5727),#31713,.T.);
#33409=ADVANCED_FACE('',(#5728),#31714,.T.);
#33410=ADVANCED_FACE('',(#5729),#31715,.T.);
#33411=ADVANCED_FACE('',(#5730),#31716,.T.);
#33412=ADVANCED_FACE('',(#5731),#629,.T.);
#33413=ADVANCED_FACE('',(#5732),#630,.T.);
#33414=ADVANCED_FACE('',(#5733),#631,.T.);
#33415=ADVANCED_FACE('',(#5734),#632,.T.);
#33416=ADVANCED_FACE('',(#5735),#633,.T.);
#33417=ADVANCED_FACE('',(#5736),#31717,.T.);
#33418=ADVANCED_FACE('',(#5737),#31718,.T.);
#33419=ADVANCED_FACE('',(#5738),#634,.T.);
#33420=ADVANCED_FACE('',(#5739),#31719,.T.);
#33421=ADVANCED_FACE('',(#5740),#31720,.T.);
#33422=ADVANCED_FACE('',(#5741),#31721,.T.);
#33423=ADVANCED_FACE('',(#5742),#31722,.T.);
#33424=ADVANCED_FACE('',(#5743),#31723,.T.);
#33425=ADVANCED_FACE('',(#5744),#635,.T.);
#33426=ADVANCED_FACE('',(#5745),#636,.T.);
#33427=ADVANCED_FACE('',(#5746),#637,.T.);
#33428=ADVANCED_FACE('',(#5747),#638,.T.);
#33429=ADVANCED_FACE('',(#5748),#639,.T.);
#33430=ADVANCED_FACE('',(#5749),#31724,.T.);
#33431=ADVANCED_FACE('',(#5750),#31725,.T.);
#33432=ADVANCED_FACE('',(#5751),#640,.T.);
#33433=ADVANCED_FACE('',(#5752),#31726,.T.);
#33434=ADVANCED_FACE('',(#5753),#31727,.T.);
#33435=ADVANCED_FACE('',(#5754),#31728,.T.);
#33436=ADVANCED_FACE('',(#5755),#31729,.T.);
#33437=ADVANCED_FACE('',(#5756),#31730,.T.);
#33438=ADVANCED_FACE('',(#5757),#31731,.T.);
#33439=ADVANCED_FACE('',(#5758),#31732,.T.);
#33440=ADVANCED_FACE('',(#5759),#31733,.T.);
#33441=ADVANCED_FACE('',(#5760),#31734,.T.);
#33442=ADVANCED_FACE('',(#5761),#31735,.T.);
#33443=ADVANCED_FACE('',(#5762),#641,.T.);
#33444=ADVANCED_FACE('',(#5763),#642,.T.);
#33445=ADVANCED_FACE('',(#5764),#643,.T.);
#33446=ADVANCED_FACE('',(#5765),#31736,.T.);
#33447=ADVANCED_FACE('',(#5766),#31737,.T.);
#33448=ADVANCED_FACE('',(#5767),#31738,.T.);
#33449=ADVANCED_FACE('',(#5768),#31739,.T.);
#33450=ADVANCED_FACE('',(#5769),#31740,.T.);
#33451=ADVANCED_FACE('',(#5770),#31741,.T.);
#33452=ADVANCED_FACE('',(#5771),#31742,.T.);
#33453=ADVANCED_FACE('',(#5772),#644,.T.);
#33454=ADVANCED_FACE('',(#5773,#2154),#31743,.T.);
#33455=ADVANCED_FACE('',(#5774),#31744,.T.);
#33456=ADVANCED_FACE('',(#5775),#31745,.T.);
#33457=ADVANCED_FACE('',(#5776),#31746,.T.);
#33458=ADVANCED_FACE('',(#5777),#31747,.T.);
#33459=ADVANCED_FACE('',(#5778),#31748,.T.);
#33460=ADVANCED_FACE('',(#5779),#31749,.T.);
#33461=ADVANCED_FACE('',(#5780),#31750,.T.);
#33462=ADVANCED_FACE('',(#5781),#645,.T.);
#33463=ADVANCED_FACE('',(#5782,#2155),#31751,.T.);
#33464=ADVANCED_FACE('',(#5783),#31752,.T.);
#33465=ADVANCED_FACE('',(#5784),#31753,.T.);
#33466=ADVANCED_FACE('',(#5785),#31754,.T.);
#33467=ADVANCED_FACE('',(#5786,#2156),#31755,.T.);
#33468=ADVANCED_FACE('',(#5787),#646,.T.);
#33469=ADVANCED_FACE('',(#5788),#647,.F.);
#33470=ADVANCED_FACE('',(#5789),#1777,.F.);
#33471=ADVANCED_FACE('',(#5790),#648,.F.);
#33472=ADVANCED_FACE('',(#5791),#649,.F.);
#33473=ADVANCED_FACE('',(#5792),#1778,.F.);
#33474=ADVANCED_FACE('',(#5793),#650,.F.);
#33475=ADVANCED_FACE('',(#5794),#651,.F.);
#33476=ADVANCED_FACE('',(#5795),#1779,.F.);
#33477=ADVANCED_FACE('',(#5796),#652,.F.);
#33478=ADVANCED_FACE('',(#5797),#653,.F.);
#33479=ADVANCED_FACE('',(#5798),#1780,.F.);
#33480=ADVANCED_FACE('',(#5799),#654,.F.);
#33481=ADVANCED_FACE('',(#5800),#655,.F.);
#33482=ADVANCED_FACE('',(#5801),#1781,.F.);
#33483=ADVANCED_FACE('',(#5802),#656,.F.);
#33484=ADVANCED_FACE('',(#5803),#657,.F.);
#33485=ADVANCED_FACE('',(#5804),#1782,.F.);
#33486=ADVANCED_FACE('',(#5805),#658,.F.);
#33487=ADVANCED_FACE('',(#5806),#659,.F.);
#33488=ADVANCED_FACE('',(#5807),#1783,.F.);
#33489=ADVANCED_FACE('',(#5808),#660,.F.);
#33490=ADVANCED_FACE('',(#5809),#661,.F.);
#33491=ADVANCED_FACE('',(#5810),#662,.F.);
#33492=ADVANCED_FACE('',(#5811),#663,.F.);
#33493=ADVANCED_FACE('',(#5812),#664,.F.);
#33494=ADVANCED_FACE('',(#5813),#665,.F.);
#33495=ADVANCED_FACE('',(#5814),#666,.F.);
#33496=ADVANCED_FACE('',(#5815),#667,.F.);
#33497=ADVANCED_FACE('',(#5816),#668,.F.);
#33498=ADVANCED_FACE('',(#5817),#31756,.T.);
#33499=ADVANCED_FACE('',(#5818),#31757,.T.);
#33500=ADVANCED_FACE('',(#5819),#31758,.T.);
#33501=ADVANCED_FACE('',(#5820),#31759,.T.);
#33502=ADVANCED_FACE('',(#5821),#31760,.T.);
#33503=ADVANCED_FACE('',(#5822),#31761,.T.);
#33504=ADVANCED_FACE('',(#5823),#31762,.T.);
#33505=ADVANCED_FACE('',(#5824),#31763,.T.);
#33506=ADVANCED_FACE('',(#5825,#2157),#31764,.T.);
#33507=ADVANCED_FACE('',(#5826,#2158),#31765,.T.);
#33508=ADVANCED_FACE('',(#5827),#1784,.F.);
#33509=ADVANCED_FACE('',(#5828),#669,.F.);
#33510=ADVANCED_FACE('',(#5829,#2159,#2160,#2161,#2162),#31766,.T.);
#33511=ADVANCED_FACE('',(#5830),#31767,.T.);
#33512=ADVANCED_FACE('',(#5831),#31768,.T.);
#33513=ADVANCED_FACE('',(#5832),#31769,.T.);
#33514=ADVANCED_FACE('',(#5833),#31770,.T.);
#33515=ADVANCED_FACE('',(#5834),#31771,.T.);
#33516=ADVANCED_FACE('',(#5835),#31772,.T.);
#33517=ADVANCED_FACE('',(#5836),#31773,.T.);
#33518=ADVANCED_FACE('',(#5837,#2163,#2164,#2165,#2166,#2167),#31774,.T.);
#33519=ADVANCED_FACE('',(#5838),#31775,.T.);
#33520=ADVANCED_FACE('',(#5839),#31776,.T.);
#33521=ADVANCED_FACE('',(#5840),#670,.T.);
#33522=ADVANCED_FACE('',(#5841),#671,.F.);
#33523=ADVANCED_FACE('',(#5842),#1785,.F.);
#33524=ADVANCED_FACE('',(#5843),#672,.F.);
#33525=ADVANCED_FACE('',(#5844),#1786,.F.);
#33526=ADVANCED_FACE('',(#5845),#673,.T.);
#33527=ADVANCED_FACE('',(#5846),#674,.T.);
#33528=ADVANCED_FACE('',(#5847),#1787,.F.);
#33529=ADVANCED_FACE('',(#5848),#675,.F.);
#33530=ADVANCED_FACE('',(#5849,#2168,#2169,#2170,#2171,#2172),#31777,.T.);
#33531=ADVANCED_FACE('',(#5850,#2173),#31778,.T.);
#33532=ADVANCED_FACE('',(#5851),#1788,.T.);
#33533=ADVANCED_FACE('',(#5852,#2174),#31779,.T.);
#33534=ADVANCED_FACE('',(#5853),#1789,.F.);
#33535=ADVANCED_FACE('',(#5854),#676,.T.);
#33536=ADVANCED_FACE('',(#5855,#2175),#31780,.T.);
#33537=ADVANCED_FACE('',(#5856),#677,.F.);
#33538=ADVANCED_FACE('',(#5857,#2176),#31781,.T.);
#33539=ADVANCED_FACE('',(#5858,#2177,#2178),#1790,.F.);
#33540=ADVANCED_FACE('',(#5859),#1791,.F.);
#33541=ADVANCED_FACE('',(#5860,#2179,#2180),#31782,.T.);
#33542=ADVANCED_FACE('',(#5861),#31783,.T.);
#33543=ADVANCED_FACE('',(#5862),#31784,.T.);
#33544=ADVANCED_FACE('',(#5863),#31785,.T.);
#33545=ADVANCED_FACE('',(#5864),#31786,.T.);
#33546=ADVANCED_FACE('',(#5865),#31787,.T.);
#33547=ADVANCED_FACE('',(#5866),#31788,.T.);
#33548=ADVANCED_FACE('',(#5867),#31789,.T.);
#33549=ADVANCED_FACE('',(#5868),#31790,.T.);
#33550=ADVANCED_FACE('',(#5869),#31791,.T.);
#33551=ADVANCED_FACE('',(#5870),#31792,.T.);
#33552=ADVANCED_FACE('',(#5871),#31793,.T.);
#33553=ADVANCED_FACE('',(#5872),#31794,.T.);
#33554=ADVANCED_FACE('',(#5873),#31795,.T.);
#33555=ADVANCED_FACE('',(#5874),#31796,.T.);
#33556=ADVANCED_FACE('',(#5875,#2181),#31797,.T.);
#33557=ADVANCED_FACE('',(#5876),#678,.T.);
#33558=ADVANCED_FACE('',(#5877),#1792,.T.);
#33559=ADVANCED_FACE('',(#5878),#679,.T.);
#33560=ADVANCED_FACE('',(#5879),#31798,.T.);
#33561=ADVANCED_FACE('',(#5880,#2182),#31799,.T.);
#33562=ADVANCED_FACE('',(#5881),#680,.T.);
#33563=ADVANCED_FACE('',(#5882),#31800,.T.);
#33564=ADVANCED_FACE('',(#5883),#31801,.T.);
#33565=ADVANCED_FACE('',(#5884),#31802,.T.);
#33566=ADVANCED_FACE('',(#5885),#31803,.T.);
#33567=ADVANCED_FACE('',(#5886),#31804,.T.);
#33568=ADVANCED_FACE('',(#5887),#31805,.T.);
#33569=ADVANCED_FACE('',(#5888),#31806,.T.);
#33570=ADVANCED_FACE('',(#5889),#31807,.T.);
#33571=ADVANCED_FACE('',(#5890),#31808,.T.);
#33572=ADVANCED_FACE('',(#5891),#31809,.T.);
#33573=ADVANCED_FACE('',(#5892),#31810,.T.);
#33574=ADVANCED_FACE('',(#5893),#31811,.T.);
#33575=ADVANCED_FACE('',(#5894),#31812,.T.);
#33576=ADVANCED_FACE('',(#5895),#31813,.T.);
#33577=ADVANCED_FACE('',(#5896,#2183),#31814,.T.);
#33578=ADVANCED_FACE('',(#5897),#681,.T.);
#33579=ADVANCED_FACE('',(#5898),#1793,.T.);
#33580=ADVANCED_FACE('',(#5899),#682,.T.);
#33581=ADVANCED_FACE('',(#5900),#31815,.T.);
#33582=ADVANCED_FACE('',(#5901,#2184),#31816,.T.);
#33583=ADVANCED_FACE('',(#5902),#683,.T.);
#33584=ADVANCED_FACE('',(#5903),#1794,.T.);
#33585=ADVANCED_FACE('',(#5904),#684,.T.);
#33586=ADVANCED_FACE('',(#5905),#31817,.T.);
#33587=ADVANCED_FACE('',(#5906),#1795,.F.);
#33588=ADVANCED_FACE('',(#5907),#1796,.F.);
#33589=ADVANCED_FACE('',(#5908),#31818,.T.);
#33590=ADVANCED_FACE('',(#5909),#685,.T.);
#33591=ADVANCED_FACE('',(#5910),#1797,.T.);
#33592=ADVANCED_FACE('',(#5911,#2185,#2186),#1798,.T.);
#33593=ADVANCED_FACE('',(#5912),#686,.T.);
#33594=ADVANCED_FACE('',(#5913),#31819,.T.);
#33595=ADVANCED_FACE('',(#5914),#687,.F.);
#33596=ADVANCED_FACE('',(#5915),#31820,.T.);
#33597=ADVANCED_FACE('',(#5916,#2187,#2188),#1799,.T.);
#33598=ADVANCED_FACE('',(#5917,#2189),#31821,.T.);
#33599=ADVANCED_FACE('',(#5918,#2190),#31822,.T.);
#33600=ADVANCED_FACE('',(#5919),#1800,.T.);
#33601=ADVANCED_FACE('',(#5920),#1801,.T.);
#33602=ADVANCED_FACE('',(#5921,#2191),#31823,.T.);
#33603=ADVANCED_FACE('',(#5922,#2192),#31824,.T.);
#33604=ADVANCED_FACE('',(#5923),#1802,.T.);
#33605=ADVANCED_FACE('',(#5924),#31825,.T.);
#33606=ADVANCED_FACE('',(#5925),#688,.T.);
#33607=ADVANCED_FACE('',(#5926),#31826,.T.);
#33608=ADVANCED_FACE('',(#5927),#31827,.T.);
#33609=ADVANCED_FACE('',(#5928),#689,.T.);
#33610=ADVANCED_FACE('',(#5929),#690,.T.);
#33611=ADVANCED_FACE('',(#5930),#691,.T.);
#33612=ADVANCED_FACE('',(#5931),#692,.T.);
#33613=ADVANCED_FACE('',(#5932),#693,.T.);
#33614=ADVANCED_FACE('',(#5933),#31828,.T.);
#33615=ADVANCED_FACE('',(#5934),#31829,.T.);
#33616=ADVANCED_FACE('',(#5935),#31830,.T.);
#33617=ADVANCED_FACE('',(#5936),#31831,.T.);
#33618=ADVANCED_FACE('',(#5937),#31832,.T.);
#33619=ADVANCED_FACE('',(#5938),#694,.T.);
#33620=ADVANCED_FACE('',(#5939),#31833,.T.);
#33621=ADVANCED_FACE('',(#5940),#31834,.T.);
#33622=ADVANCED_FACE('',(#5941),#695,.T.);
#33623=ADVANCED_FACE('',(#5942),#696,.T.);
#33624=ADVANCED_FACE('',(#5943),#697,.T.);
#33625=ADVANCED_FACE('',(#5944),#698,.T.);
#33626=ADVANCED_FACE('',(#5945),#699,.T.);
#33627=ADVANCED_FACE('',(#5946),#31835,.T.);
#33628=ADVANCED_FACE('',(#5947),#31836,.T.);
#33629=ADVANCED_FACE('',(#5948),#31837,.T.);
#33630=ADVANCED_FACE('',(#5949),#31838,.T.);
#33631=ADVANCED_FACE('',(#5950,#2193),#31839,.T.);
#33632=ADVANCED_FACE('',(#5951,#2194),#31840,.T.);
#33633=ADVANCED_FACE('',(#5952,#2195),#31841,.T.);
#33634=ADVANCED_FACE('',(#5953),#1803,.F.);
#33635=ADVANCED_FACE('',(#5954),#1804,.F.);
#33636=ADVANCED_FACE('',(#5955),#1805,.F.);
#33637=ADVANCED_FACE('',(#5956),#1806,.F.);
#33638=ADVANCED_FACE('',(#5957),#1807,.F.);
#33639=ADVANCED_FACE('',(#5958),#1808,.F.);
#33640=ADVANCED_FACE('',(#5959),#1809,.F.);
#33641=ADVANCED_FACE('',(#5960),#31842,.T.);
#33642=ADVANCED_FACE('',(#5961),#31843,.T.);
#33643=ADVANCED_FACE('',(#5962),#1810,.F.);
#33644=ADVANCED_FACE('',(#5963),#1811,.F.);
#33645=ADVANCED_FACE('',(#5964),#1812,.F.);
#33646=ADVANCED_FACE('',(#5965),#31844,.T.);
#33647=ADVANCED_FACE('',(#5966),#1813,.F.);
#33648=ADVANCED_FACE('',(#5967),#1814,.T.);
#33649=ADVANCED_FACE('',(#5968),#1815,.F.);
#33650=ADVANCED_FACE('',(#5969),#31845,.T.);
#33651=ADVANCED_FACE('',(#5970),#31846,.T.);
#33652=ADVANCED_FACE('',(#5971),#1816,.F.);
#33653=ADVANCED_FACE('',(#5972),#1817,.F.);
#33654=ADVANCED_FACE('',(#5973),#1818,.F.);
#33655=ADVANCED_FACE('',(#5974),#31847,.T.);
#33656=ADVANCED_FACE('',(#5975),#1819,.F.);
#33657=ADVANCED_FACE('',(#5976),#1820,.T.);
#33658=ADVANCED_FACE('',(#5977),#1821,.F.);
#33659=ADVANCED_FACE('',(#5978),#31848,.T.);
#33660=ADVANCED_FACE('',(#5979),#31849,.T.);
#33661=ADVANCED_FACE('',(#5980),#1822,.F.);
#33662=ADVANCED_FACE('',(#5981),#1823,.F.);
#33663=ADVANCED_FACE('',(#5982),#1824,.F.);
#33664=ADVANCED_FACE('',(#5983),#31850,.T.);
#33665=ADVANCED_FACE('',(#5984),#1825,.F.);
#33666=ADVANCED_FACE('',(#5985),#1826,.T.);
#33667=ADVANCED_FACE('',(#5986),#1827,.F.);
#33668=ADVANCED_FACE('',(#5987),#31851,.T.);
#33669=ADVANCED_FACE('',(#5988),#1828,.F.);
#33670=ADVANCED_FACE('',(#5989),#1829,.F.);
#33671=ADVANCED_FACE('',(#5990),#1830,.F.);
#33672=ADVANCED_FACE('',(#5991),#1831,.F.);
#33673=ADVANCED_FACE('',(#5992),#31852,.T.);
#33674=ADVANCED_FACE('',(#5993),#1832,.F.);
#33675=ADVANCED_FACE('',(#5994),#31853,.T.);
#33676=ADVANCED_FACE('',(#5995),#1833,.F.);
#33677=ADVANCED_FACE('',(#5996),#31854,.T.);
#33678=ADVANCED_FACE('',(#5997,#2196),#31855,.T.);
#33679=ADVANCED_FACE('',(#5998,#2197),#31856,.T.);
#33680=ADVANCED_FACE('',(#5999,#2198),#31857,.T.);
#33681=ADVANCED_FACE('',(#6000),#700,.T.);
#33682=ADVANCED_FACE('',(#6001),#31858,.T.);
#33683=ADVANCED_FACE('',(#6002),#31859,.T.);
#33684=ADVANCED_FACE('',(#6003),#31860,.T.);
#33685=ADVANCED_FACE('',(#6004),#31861,.T.);
#33686=ADVANCED_FACE('',(#6005),#31862,.T.);
#33687=ADVANCED_FACE('',(#6006),#701,.F.);
#33688=ADVANCED_FACE('',(#6007),#31863,.T.);
#33689=ADVANCED_FACE('',(#6008),#702,.F.);
#33690=ADVANCED_FACE('',(#6009),#31864,.T.);
#33691=ADVANCED_FACE('',(#6010),#703,.F.);
#33692=ADVANCED_FACE('',(#6011),#31865,.T.);
#33693=ADVANCED_FACE('',(#6012),#704,.F.);
#33694=ADVANCED_FACE('',(#6013,#2199),#31866,.T.);
#33695=ADVANCED_FACE('',(#6014),#31867,.T.);
#33696=ADVANCED_FACE('',(#6015),#1834,.T.);
#33697=ADVANCED_FACE('',(#6016),#31868,.T.);
#33698=ADVANCED_FACE('',(#6017),#31869,.T.);
#33699=ADVANCED_FACE('',(#6018),#1835,.T.);
#33700=ADVANCED_FACE('',(#6019),#31870,.T.);
#33701=ADVANCED_FACE('',(#6020),#31871,.T.);
#33702=ADVANCED_FACE('',(#6021),#1836,.T.);
#33703=ADVANCED_FACE('',(#6022),#31872,.T.);
#33704=ADVANCED_FACE('',(#6023),#31873,.T.);
#33705=ADVANCED_FACE('',(#6024),#1837,.T.);
#33706=ADVANCED_FACE('',(#6025),#31874,.T.);
#33707=ADVANCED_FACE('',(#6026,#2200),#31875,.T.);
#33708=ADVANCED_FACE('',(#6027),#1838,.F.);
#33709=ADVANCED_FACE('',(#6028),#31876,.T.);
#33710=ADVANCED_FACE('',(#6029),#1839,.F.);
#33711=ADVANCED_FACE('',(#6030),#31877,.T.);
#33712=ADVANCED_FACE('',(#6031),#1840,.F.);
#33713=ADVANCED_FACE('',(#6032),#1841,.T.);
#33714=ADVANCED_FACE('',(#6033),#1842,.F.);
#33715=ADVANCED_FACE('',(#6034),#31878,.T.);
#33716=ADVANCED_FACE('',(#6035),#1843,.F.);
#33717=ADVANCED_FACE('',(#6036),#1844,.F.);
#33718=ADVANCED_FACE('',(#6037),#31879,.T.);
#33719=ADVANCED_FACE('',(#6038),#31880,.T.);
#33720=ADVANCED_FACE('',(#6039),#1845,.F.);
#33721=ADVANCED_FACE('',(#6040),#1846,.T.);
#33722=ADVANCED_FACE('',(#6041),#1847,.F.);
#33723=ADVANCED_FACE('',(#6042),#31881,.T.);
#33724=ADVANCED_FACE('',(#6043),#1848,.F.);
#33725=ADVANCED_FACE('',(#6044),#1849,.F.);
#33726=ADVANCED_FACE('',(#6045),#1850,.F.);
#33727=ADVANCED_FACE('',(#6046),#31882,.T.);
#33728=ADVANCED_FACE('',(#6047),#1851,.F.);
#33729=ADVANCED_FACE('',(#6048),#1852,.F.);
#33730=ADVANCED_FACE('',(#6049),#31883,.T.);
#33731=ADVANCED_FACE('',(#6050),#1853,.F.);
#33732=ADVANCED_FACE('',(#6051),#1854,.T.);
#33733=ADVANCED_FACE('',(#6052),#1855,.F.);
#33734=ADVANCED_FACE('',(#6053),#31884,.T.);
#33735=ADVANCED_FACE('',(#6054),#1856,.F.);
#33736=ADVANCED_FACE('',(#6055),#31885,.T.);
#33737=ADVANCED_FACE('',(#6056),#1857,.F.);
#33738=ADVANCED_FACE('',(#6057),#1858,.F.);
#33739=ADVANCED_FACE('',(#6058),#31886,.T.);
#33740=ADVANCED_FACE('',(#6059),#1859,.F.);
#33741=ADVANCED_FACE('',(#6060),#1860,.T.);
#33742=ADVANCED_FACE('',(#6061),#1861,.F.);
#33743=ADVANCED_FACE('',(#6062),#31887,.T.);
#33744=ADVANCED_FACE('',(#6063),#1862,.F.);
#33745=ADVANCED_FACE('',(#6064),#31888,.T.);
#33746=ADVANCED_FACE('',(#6065),#1863,.T.);
#33747=ADVANCED_FACE('',(#6066),#1864,.F.);
#33748=ADVANCED_FACE('',(#6067),#31889,.T.);
#33749=ADVANCED_FACE('',(#6068),#1865,.F.);
#33750=ADVANCED_FACE('',(#6069),#1866,.F.);
#33751=ADVANCED_FACE('',(#6070),#1867,.F.);
#33752=ADVANCED_FACE('',(#6071),#1868,.F.);
#33753=ADVANCED_FACE('',(#6072),#31890,.T.);
#33754=ADVANCED_FACE('',(#6073),#910,.T.);
#33755=ADVANCED_FACE('',(#6074,#2201,#2202,#2203,#2204,#2205,#2206,#2207),
#31891,.T.);
#33756=ADVANCED_FACE('',(#6075),#31892,.T.);
#33757=ADVANCED_FACE('',(#6076),#31893,.T.);
#33758=ADVANCED_FACE('',(#6077),#31894,.T.);
#33759=ADVANCED_FACE('',(#6078),#31895,.T.);
#33760=ADVANCED_FACE('',(#6079),#31896,.T.);
#33761=ADVANCED_FACE('',(#6080,#2208,#2209,#2210,#2211,#2212,#2213,#2214,
#2215,#2216,#2217,#2218,#2219,#2220,#2221,#2222),#31897,.T.);
#33762=ADVANCED_FACE('',(#6081),#31898,.T.);
#33763=ADVANCED_FACE('',(#6082),#31899,.T.);
#33764=ADVANCED_FACE('',(#6083),#31900,.T.);
#33765=ADVANCED_FACE('',(#6084,#2223),#31901,.T.);
#33766=ADVANCED_FACE('',(#6085),#705,.T.);
#33767=ADVANCED_FACE('',(#6086),#1869,.T.);
#33768=ADVANCED_FACE('',(#6087),#706,.T.);
#33769=ADVANCED_FACE('',(#6088),#31902,.T.);
#33770=ADVANCED_FACE('',(#6089),#31903,.T.);
#33771=ADVANCED_FACE('',(#6090),#31904,.T.);
#33772=ADVANCED_FACE('',(#6091),#31905,.T.);
#33773=ADVANCED_FACE('',(#6092),#31906,.T.);
#33774=ADVANCED_FACE('',(#6093),#31907,.T.);
#33775=ADVANCED_FACE('',(#6094),#31908,.T.);
#33776=ADVANCED_FACE('',(#6095,#2224),#31909,.T.);
#33828=CLOSED_SHELL('',(#33325,#33326,#33327,#33328));
#33829=CLOSED_SHELL('',(#33329,#33330,#33331,#33332));
#33830=CLOSED_SHELL('',(#33333,#33334,#33335,#33336));
#33831=CLOSED_SHELL('',(#33337,#33338,#33339,#33340));
#33832=CLOSED_SHELL('',(#33341,#33342,#33343,#33344));
#33833=CLOSED_SHELL('',(#33345,#33346,#33347,#33348));
#33834=CLOSED_SHELL('',(#33349,#33350,#33351,#33352));
#33835=CLOSED_SHELL('',(#33353,#33354,#33355,#33356));
#33836=CLOSED_SHELL('',(#33357,#33358,#33359,#33360));
#33837=CLOSED_SHELL('',(#33361,#33362,#33363,#33364));
#33838=CLOSED_SHELL('',(#33365,#33366,#33367,#33368,#33369,#33370,#33371,
#33372,#33373,#33374,#33375,#33376,#33377,#33378,#33379,#33380,#33381,#33382,
#33383,#33384,#33385,#33386,#33387,#33388,#33389,#33390,#33391,#33392,#33393,
#33394,#33395,#33396,#33397,#33398,#33399,#33400,#33401,#33402,#33403,#33404,
#33405,#33406,#33407,#33408,#33409,#33410,#33411,#33412,#33413,#33414,#33415,
#33416,#33417,#33418,#33419,#33420,#33421,#33422,#33423,#33424,#33425,#33426,
#33427,#33428,#33429,#33430,#33431,#33432,#33433,#33434,#33435,#33436,#33437,
#33438,#33439,#33440,#33441,#33442,#33443,#33444,#33445,#33446,#33447,#33448,
#33449,#33450,#33451,#33452,#33453,#33454,#33455,#33456,#33457,#33458,#33459,
#33460,#33461,#33462,#33463,#33464,#33465,#33466,#33467,#33468,#33469,#33470,
#33471,#33472,#33473,#33474,#33475,#33476,#33477,#33478,#33479,#33480,#33481,
#33482,#33483,#33484,#33485,#33486,#33487,#33488,#33489,#33490,#33491,#33492,
#33493,#33494,#33495,#33496,#33497,#33498,#33499,#33500,#33501,#33502,#33503,
#33504,#33505,#33506,#33507,#33508,#33509,#33510,#33511,#33512,#33513,#33514,
#33515,#33516,#33517,#33518,#33519,#33520,#33521,#33522,#33523,#33524,#33525,
#33526,#33527,#33528,#33529,#33530,#33531,#33532,#33533,#33534,#33535,#33536,
#33537,#33538,#33539,#33540,#33541,#33542,#33543,#33544,#33545,#33546,#33547,
#33548,#33549,#33550,#33551,#33552,#33553,#33554,#33555,#33556,#33557,#33558,
#33559,#33560,#33561,#33562,#33563,#33564,#33565,#33566,#33567,#33568,#33569,
#33570,#33571,#33572,#33573,#33574,#33575,#33576,#33577,#33578,#33579,#33580,
#33581,#33582,#33583,#33584,#33585,#33586,#33587,#33588,#33589,#33590,#33591,
#33592,#33593,#33594,#33595,#33596,#33597,#33598,#33599,#33600,#33601,#33602,
#33603,#33604,#33605,#33606,#33607,#33608,#33609,#33610,#33611,#33612,#33613,
#33614,#33615,#33616,#33617,#33618,#33619,#33620,#33621,#33622,#33623,#33624,
#33625,#33626,#33627,#33628,#33629,#33630,#33631,#33632,#33633,#33634,#33635,
#33636,#33637,#33638,#33639,#33640,#33641,#33642,#33643,#33644,#33645,#33646,
#33647,#33648,#33649,#33650,#33651,#33652,#33653,#33654,#33655,#33656,#33657,
#33658,#33659,#33660,#33661,#33662,#33663,#33664,#33665,#33666,#33667,#33668,
#33669,#33670,#33671,#33672,#33673,#33674,#33675,#33676,#33677,#33678,#33679,
#33680,#33681,#33682,#33683,#33684,#33685,#33686,#33687,#33688,#33689,#33690,
#33691,#33692,#33693,#33694,#33695,#33696,#33697,#33698,#33699,#33700,#33701,
#33702,#33703,#33704,#33705,#33706,#33707,#33708,#33709,#33710,#33711,#33712,
#33713,#33714,#33715,#33716,#33717,#33718,#33719,#33720,#33721,#33722,#33723,
#33724,#33725,#33726,#33727,#33728,#33729,#33730,#33731,#33732,#33733,#33734,
#33735,#33736,#33737,#33738,#33739,#33740,#33741,#33742,#33743,#33744,#33745,
#33746,#33747,#33748,#33749,#33750,#33751,#33752,#33753,#33754,#33755,#33756,
#33757,#33758,#33759,#33760,#33761,#33762,#33763,#33764,#33765,#33766,#33767,
#33768,#33769,#33770,#33771,#33772,#33773,#33774,#33775,#33776));
#37247=AXIS2_PLACEMENT_3D('',#58607,#46290,#46291);
#37248=AXIS2_PLACEMENT_3D('',#58608,#46292,#46293);
#37249=AXIS2_PLACEMENT_3D('',#58611,#46294,#46295);
#37250=AXIS2_PLACEMENT_3D('',#58612,#46296,#46297);
#37251=AXIS2_PLACEMENT_3D('',#58615,#46299,#46300);
#37252=AXIS2_PLACEMENT_3D('',#58616,#46301,#46302);
#37253=AXIS2_PLACEMENT_3D('',#58617,#46303,#46304);
#37254=AXIS2_PLACEMENT_3D('',#58622,#46306,#46307);
#37255=AXIS2_PLACEMENT_3D('',#58623,#46308,#46309);
#37256=AXIS2_PLACEMENT_3D('',#58624,#46310,#46311);
#37257=AXIS2_PLACEMENT_3D('',#58626,#46313,#46314);
#37258=AXIS2_PLACEMENT_3D('',#58628,#46315,#46316);
#37259=AXIS2_PLACEMENT_3D('',#58631,#46318,#46319);
#37260=AXIS2_PLACEMENT_3D('',#58632,#46320,#46321);
#37261=AXIS2_PLACEMENT_3D('',#58634,#46322,#46323);
#37262=AXIS2_PLACEMENT_3D('',#58635,#46324,#46325);
#37263=AXIS2_PLACEMENT_3D('',#58637,#46326,#46327);
#37264=AXIS2_PLACEMENT_3D('',#58638,#46328,#46329);
#37265=AXIS2_PLACEMENT_3D('',#58640,#46331,#46332);
#37266=AXIS2_PLACEMENT_3D('',#58643,#46333,#46334);
#37267=AXIS2_PLACEMENT_3D('',#58644,#46335,#46336);
#37268=AXIS2_PLACEMENT_3D('',#58647,#46338,#46339);
#37269=AXIS2_PLACEMENT_3D('',#58648,#46340,#46341);
#37270=AXIS2_PLACEMENT_3D('',#58649,#46342,#46343);
#37271=AXIS2_PLACEMENT_3D('',#58654,#46345,#46346);
#37272=AXIS2_PLACEMENT_3D('',#58655,#46347,#46348);
#37273=AXIS2_PLACEMENT_3D('',#58656,#46349,#46350);
#37274=AXIS2_PLACEMENT_3D('',#58658,#46352,#46353);
#37275=AXIS2_PLACEMENT_3D('',#58660,#46354,#46355);
#37276=AXIS2_PLACEMENT_3D('',#58663,#46357,#46358);
#37277=AXIS2_PLACEMENT_3D('',#58664,#46359,#46360);
#37278=AXIS2_PLACEMENT_3D('',#58666,#46361,#46362);
#37279=AXIS2_PLACEMENT_3D('',#58667,#46363,#46364);
#37280=AXIS2_PLACEMENT_3D('',#58669,#46365,#46366);
#37281=AXIS2_PLACEMENT_3D('',#58670,#46367,#46368);
#37282=AXIS2_PLACEMENT_3D('',#58672,#46370,#46371);
#37283=AXIS2_PLACEMENT_3D('',#58675,#46372,#46373);
#37284=AXIS2_PLACEMENT_3D('',#58678,#46375,#46376);
#37285=AXIS2_PLACEMENT_3D('',#58679,#46377,#46378);
#37286=AXIS2_PLACEMENT_3D('',#58680,#46379,#46380);
#37287=AXIS2_PLACEMENT_3D('',#58681,#46381,#46382);
#37288=AXIS2_PLACEMENT_3D('',#58684,#46383,#46384);
#37289=AXIS2_PLACEMENT_3D('',#58685,#46385,#46386);
#37290=AXIS2_PLACEMENT_3D('',#58687,#46388,#46389);
#37291=AXIS2_PLACEMENT_3D('',#58690,#46391,#46392);
#37292=AXIS2_PLACEMENT_3D('',#58692,#46393,#46394);
#37293=AXIS2_PLACEMENT_3D('',#58695,#46396,#46397);
#37294=AXIS2_PLACEMENT_3D('',#58696,#46398,#46399);
#37295=AXIS2_PLACEMENT_3D('',#58698,#46400,#46401);
#37296=AXIS2_PLACEMENT_3D('',#58699,#46402,#46403);
#37297=AXIS2_PLACEMENT_3D('',#58701,#46404,#46405);
#37298=AXIS2_PLACEMENT_3D('',#58703,#46407,#46408);
#37299=AXIS2_PLACEMENT_3D('',#58704,#46409,#46410);
#37300=AXIS2_PLACEMENT_3D('',#58706,#46411,#46412);
#37301=AXIS2_PLACEMENT_3D('',#58709,#46414,#46415);
#37302=AXIS2_PLACEMENT_3D('',#58710,#46416,#46417);
#37303=AXIS2_PLACEMENT_3D('',#58712,#46418,#46419);
#37304=AXIS2_PLACEMENT_3D('',#58713,#46420,#46421);
#37305=AXIS2_PLACEMENT_3D('',#58716,#46423,#46424);
#37306=AXIS2_PLACEMENT_3D('',#58717,#46425,#46426);
#37307=AXIS2_PLACEMENT_3D('',#58718,#46427,#46428);
#37308=AXIS2_PLACEMENT_3D('',#58721,#46429,#46430);
#37309=AXIS2_PLACEMENT_3D('',#58722,#46431,#46432);
#37310=AXIS2_PLACEMENT_3D('',#58725,#46434,#46435);
#37311=AXIS2_PLACEMENT_3D('',#58726,#46436,#46437);
#37312=AXIS2_PLACEMENT_3D('',#58727,#46438,#46439);
#37313=AXIS2_PLACEMENT_3D('',#58730,#46440,#46441);
#37314=AXIS2_PLACEMENT_3D('',#58731,#46442,#46443);
#37315=AXIS2_PLACEMENT_3D('',#58733,#46445,#46446);
#37316=AXIS2_PLACEMENT_3D('',#58736,#46448,#46449);
#37317=AXIS2_PLACEMENT_3D('',#58738,#46450,#46451);
#37318=AXIS2_PLACEMENT_3D('',#58741,#46453,#46454);
#37319=AXIS2_PLACEMENT_3D('',#58742,#46455,#46456);
#37320=AXIS2_PLACEMENT_3D('',#58744,#46457,#46458);
#37321=AXIS2_PLACEMENT_3D('',#58745,#46459,#46460);
#37322=AXIS2_PLACEMENT_3D('',#58748,#46462,#46463);
#37323=AXIS2_PLACEMENT_3D('',#58749,#46464,#46465);
#37324=AXIS2_PLACEMENT_3D('',#58750,#46466,#46467);
#37325=AXIS2_PLACEMENT_3D('',#58753,#46468,#46469);
#37326=AXIS2_PLACEMENT_3D('',#58754,#46470,#46471);
#37327=AXIS2_PLACEMENT_3D('',#58757,#46473,#46474);
#37328=AXIS2_PLACEMENT_3D('',#58758,#46475,#46476);
#37329=AXIS2_PLACEMENT_3D('',#58759,#46477,#46478);
#37330=AXIS2_PLACEMENT_3D('',#58762,#46479,#46480);
#37331=AXIS2_PLACEMENT_3D('',#58763,#46481,#46482);
#37332=AXIS2_PLACEMENT_3D('',#58765,#46484,#46485);
#37333=AXIS2_PLACEMENT_3D('',#58768,#46487,#46488);
#37334=AXIS2_PLACEMENT_3D('',#58805,#46503,#46504);
#37335=AXIS2_PLACEMENT_3D('',#58808,#46505,#46506);
#37336=AXIS2_PLACEMENT_3D('',#58812,#46508,#46509);
#37337=AXIS2_PLACEMENT_3D('',#58814,#46511,#46512);
#37338=AXIS2_PLACEMENT_3D('',#58820,#46516,#46517);
#37339=AXIS2_PLACEMENT_3D('',#58823,#46518,#46519);
#37340=AXIS2_PLACEMENT_3D('',#58827,#46521,#46522);
#37341=AXIS2_PLACEMENT_3D('',#58829,#46524,#46525);
#37342=AXIS2_PLACEMENT_3D('',#58839,#46531,#46532);
#37343=AXIS2_PLACEMENT_3D('',#58846,#46537,#46538);
#37344=AXIS2_PLACEMENT_3D('',#58852,#46542,#46543);
#37345=AXIS2_PLACEMENT_3D('',#58853,#46544,#46545);
#37346=AXIS2_PLACEMENT_3D('',#58857,#46547,#46548);
#37347=AXIS2_PLACEMENT_3D('',#58865,#46553,#46554);
#37348=AXIS2_PLACEMENT_3D('',#58869,#46557,#46558);
#37349=AXIS2_PLACEMENT_3D('',#58871,#46559,#46560);
#37350=AXIS2_PLACEMENT_3D('',#58878,#46564,#46565);
#37351=AXIS2_PLACEMENT_3D('',#58880,#46566,#46567);
#37352=AXIS2_PLACEMENT_3D('',#58887,#46571,#46572);
#37353=AXIS2_PLACEMENT_3D('',#58889,#46573,#46574);
#37354=AXIS2_PLACEMENT_3D('',#58890,#46575,#46576);
#37355=AXIS2_PLACEMENT_3D('',#58892,#46577,#46578);
#37356=AXIS2_PLACEMENT_3D('',#58896,#46580,#46581);
#37357=AXIS2_PLACEMENT_3D('',#58897,#46582,#46583);
#37358=AXIS2_PLACEMENT_3D('',#58898,#46584,#46585);
#37359=AXIS2_PLACEMENT_3D('',#58899,#46586,#46587);
#37360=AXIS2_PLACEMENT_3D('',#58901,#46589,#46590);
#37361=AXIS2_PLACEMENT_3D('',#58914,#46597,#46598);
#37362=AXIS2_PLACEMENT_3D('',#58916,#46599,#46600);
#37363=AXIS2_PLACEMENT_3D('',#58918,#46601,#46602);
#37364=AXIS2_PLACEMENT_3D('',#58919,#46603,#46604);
#37365=AXIS2_PLACEMENT_3D('',#58923,#46606,#46607);
#37366=AXIS2_PLACEMENT_3D('',#58924,#46608,#46609);
#37367=AXIS2_PLACEMENT_3D('',#58925,#46610,#46611);
#37368=AXIS2_PLACEMENT_3D('',#58928,#46613,#46614);
#37369=AXIS2_PLACEMENT_3D('',#58929,#46615,#46616);
#37370=AXIS2_PLACEMENT_3D('',#58935,#46619,#46620);
#37371=AXIS2_PLACEMENT_3D('',#58939,#46622,#46623);
#37372=AXIS2_PLACEMENT_3D('',#58949,#46629,#46630);
#37373=AXIS2_PLACEMENT_3D('',#58953,#46632,#46633);
#37374=AXIS2_PLACEMENT_3D('',#58954,#46634,#46635);
#37375=AXIS2_PLACEMENT_3D('',#58955,#46636,#46637);
#37376=AXIS2_PLACEMENT_3D('',#58959,#46640,#46641);
#37377=AXIS2_PLACEMENT_3D('',#58963,#46644,#46645);
#37378=AXIS2_PLACEMENT_3D('',#58967,#46647,#46648);
#37379=AXIS2_PLACEMENT_3D('',#58968,#46649,#46650);
#37380=AXIS2_PLACEMENT_3D('',#58969,#46651,#46652);
#37381=AXIS2_PLACEMENT_3D('',#58977,#46657,#46658);
#37382=AXIS2_PLACEMENT_3D('',#58978,#46659,#46660);
#37383=AXIS2_PLACEMENT_3D('',#58979,#46661,#46662);
#37384=AXIS2_PLACEMENT_3D('',#58983,#46664,#46665);
#37385=AXIS2_PLACEMENT_3D('',#59007,#46675,#46676);
#37386=AXIS2_PLACEMENT_3D('',#59010,#46677,#46678);
#37387=AXIS2_PLACEMENT_3D('',#59014,#46680,#46681);
#37388=AXIS2_PLACEMENT_3D('',#59015,#46682,#46683);
#37389=AXIS2_PLACEMENT_3D('',#59017,#46684,#46685);
#37390=AXIS2_PLACEMENT_3D('',#59021,#46687,#46688);
#37391=AXIS2_PLACEMENT_3D('',#59023,#46689,#46690);
#37392=AXIS2_PLACEMENT_3D('',#59025,#46692,#46693);
#37393=AXIS2_PLACEMENT_3D('',#59028,#46694,#46695);
#37394=AXIS2_PLACEMENT_3D('',#59031,#46697,#46698);
#37395=AXIS2_PLACEMENT_3D('',#59033,#46699,#46700);
#37396=AXIS2_PLACEMENT_3D('',#59037,#46702,#46703);
#37397=AXIS2_PLACEMENT_3D('',#59039,#46704,#46705);
#37398=AXIS2_PLACEMENT_3D('',#59041,#46707,#46708);
#37399=AXIS2_PLACEMENT_3D('',#59045,#46711,#46712);
#37400=AXIS2_PLACEMENT_3D('',#59047,#46714,#46715);
#37401=AXIS2_PLACEMENT_3D('',#59056,#46720,#46721);
#37402=AXIS2_PLACEMENT_3D('',#59062,#46725,#46726);
#37403=AXIS2_PLACEMENT_3D('',#59068,#46730,#46731);
#37404=AXIS2_PLACEMENT_3D('',#59070,#46733,#46734);
#37405=AXIS2_PLACEMENT_3D('',#59076,#46735,#46736);
#37406=AXIS2_PLACEMENT_3D('',#59080,#46737,#46738);
#37407=AXIS2_PLACEMENT_3D('',#59083,#46740,#46741);
#37408=AXIS2_PLACEMENT_3D('',#59084,#46742,#46743);
#37409=AXIS2_PLACEMENT_3D('',#59087,#46744,#46745);
#37410=AXIS2_PLACEMENT_3D('',#59088,#46746,#46747);
#37411=AXIS2_PLACEMENT_3D('',#59091,#46749,#46750);
#37412=AXIS2_PLACEMENT_3D('',#59092,#46751,#46752);
#37413=AXIS2_PLACEMENT_3D('',#59095,#46753,#46754);
#37414=AXIS2_PLACEMENT_3D('',#59096,#46755,#46756);
#37415=AXIS2_PLACEMENT_3D('',#59099,#46758,#46759);
#37416=AXIS2_PLACEMENT_3D('',#59100,#46760,#46761);
#37417=AXIS2_PLACEMENT_3D('',#59103,#46762,#46763);
#37418=AXIS2_PLACEMENT_3D('',#59104,#46764,#46765);
#37419=AXIS2_PLACEMENT_3D('',#59107,#46767,#46768);
#37420=AXIS2_PLACEMENT_3D('',#59108,#46769,#46770);
#37421=AXIS2_PLACEMENT_3D('',#59111,#46771,#46772);
#37422=AXIS2_PLACEMENT_3D('',#59112,#46773,#46774);
#37423=AXIS2_PLACEMENT_3D('',#59115,#46776,#46777);
#37424=AXIS2_PLACEMENT_3D('',#59116,#46778,#46779);
#37425=AXIS2_PLACEMENT_3D('',#59117,#46780,#46781);
#37426=AXIS2_PLACEMENT_3D('',#59126,#46787,#46788);
#37427=AXIS2_PLACEMENT_3D('',#59133,#46793,#46794);
#37428=AXIS2_PLACEMENT_3D('',#59136,#46796,#46797);
#37429=AXIS2_PLACEMENT_3D('',#59137,#46798,#46799);
#37430=AXIS2_PLACEMENT_3D('',#59143,#46803,#46804);
#37431=AXIS2_PLACEMENT_3D('',#59150,#46807,#46808);
#37432=AXIS2_PLACEMENT_3D('',#59152,#46810,#46811);
#37433=AXIS2_PLACEMENT_3D('',#59154,#46812,#46813);
#37434=AXIS2_PLACEMENT_3D('',#59157,#46815,#46816);
#37435=AXIS2_PLACEMENT_3D('',#59158,#46817,#46818);
#37436=AXIS2_PLACEMENT_3D('',#59159,#46819,#46820);
#37437=AXIS2_PLACEMENT_3D('',#59176,#46825,#46826);
#37438=AXIS2_PLACEMENT_3D('',#59190,#46830,#46831);
#37439=AXIS2_PLACEMENT_3D('',#59204,#46835,#46836);
#37440=AXIS2_PLACEMENT_3D('',#59218,#46840,#46841);
#37441=AXIS2_PLACEMENT_3D('',#59223,#46842,#46843);
#37442=AXIS2_PLACEMENT_3D('',#59224,#46844,#46845);
#37443=AXIS2_PLACEMENT_3D('',#59225,#46846,#46847);
#37444=AXIS2_PLACEMENT_3D('',#59226,#46848,#46849);
#37445=AXIS2_PLACEMENT_3D('',#59236,#46850,#46851);
#37446=AXIS2_PLACEMENT_3D('',#59237,#46852,#46853);
#37447=AXIS2_PLACEMENT_3D('',#59242,#46854,#46855);
#37448=AXIS2_PLACEMENT_3D('',#59243,#46856,#46857);
#37449=AXIS2_PLACEMENT_3D('',#59244,#46858,#46859);
#37450=AXIS2_PLACEMENT_3D('',#59245,#46860,#46861);
#37451=AXIS2_PLACEMENT_3D('',#59250,#46865,#46866);
#37452=AXIS2_PLACEMENT_3D('',#59253,#46869,#46870);
#37453=AXIS2_PLACEMENT_3D('',#59254,#46871,#46872);
#37454=AXIS2_PLACEMENT_3D('',#59255,#46873,#46874);
#37455=AXIS2_PLACEMENT_3D('',#59256,#46875,#46876);
#37456=AXIS2_PLACEMENT_3D('',#59273,#46881,#46882);
#37457=AXIS2_PLACEMENT_3D('',#59287,#46886,#46887);
#37458=AXIS2_PLACEMENT_3D('',#59301,#46891,#46892);
#37459=AXIS2_PLACEMENT_3D('',#59315,#46896,#46897);
#37460=AXIS2_PLACEMENT_3D('',#59320,#46898,#46899);
#37461=AXIS2_PLACEMENT_3D('',#59321,#46900,#46901);
#37462=AXIS2_PLACEMENT_3D('',#59322,#46902,#46903);
#37463=AXIS2_PLACEMENT_3D('',#59323,#46904,#46905);
#37464=AXIS2_PLACEMENT_3D('',#59333,#46906,#46907);
#37465=AXIS2_PLACEMENT_3D('',#59334,#46908,#46909);
#37466=AXIS2_PLACEMENT_3D('',#59339,#46910,#46911);
#37467=AXIS2_PLACEMENT_3D('',#59340,#46912,#46913);
#37468=AXIS2_PLACEMENT_3D('',#59341,#46914,#46915);
#37469=AXIS2_PLACEMENT_3D('',#59342,#46916,#46917);
#37470=AXIS2_PLACEMENT_3D('',#59347,#46921,#46922);
#37471=AXIS2_PLACEMENT_3D('',#59350,#46925,#46926);
#37472=AXIS2_PLACEMENT_3D('',#59351,#46927,#46928);
#37473=AXIS2_PLACEMENT_3D('',#59352,#46929,#46930);
#37474=AXIS2_PLACEMENT_3D('',#59353,#46931,#46932);
#37475=AXIS2_PLACEMENT_3D('',#59357,#46935,#46936);
#37476=AXIS2_PLACEMENT_3D('',#59363,#46940,#46941);
#37477=AXIS2_PLACEMENT_3D('',#59367,#46944,#46945);
#37478=AXIS2_PLACEMENT_3D('',#59371,#46948,#46949);
#37479=AXIS2_PLACEMENT_3D('',#59375,#46952,#46953);
#37480=AXIS2_PLACEMENT_3D('',#59379,#46956,#46957);
#37481=AXIS2_PLACEMENT_3D('',#59381,#46959,#46960);
#37482=AXIS2_PLACEMENT_3D('',#59382,#46961,#46962);
#37483=AXIS2_PLACEMENT_3D('',#59384,#46964,#46965);
#37484=AXIS2_PLACEMENT_3D('',#59386,#46967,#46968);
#37485=AXIS2_PLACEMENT_3D('',#59387,#46969,#46970);
#37486=AXIS2_PLACEMENT_3D('',#59388,#46971,#46972);
#37487=AXIS2_PLACEMENT_3D('',#59389,#46973,#46974);
#37488=AXIS2_PLACEMENT_3D('',#59390,#46975,#46976);
#37489=AXIS2_PLACEMENT_3D('',#59391,#46977,#46978);
#37490=AXIS2_PLACEMENT_3D('',#59392,#46979,#46980);
#37491=AXIS2_PLACEMENT_3D('',#59405,#46987,#46988);
#37492=AXIS2_PLACEMENT_3D('',#59411,#46992,#46993);
#37493=AXIS2_PLACEMENT_3D('',#59415,#46996,#46997);
#37494=AXIS2_PLACEMENT_3D('',#59419,#47000,#47001);
#37495=AXIS2_PLACEMENT_3D('',#59423,#47004,#47005);
#37496=AXIS2_PLACEMENT_3D('',#59427,#47008,#47009);
#37497=AXIS2_PLACEMENT_3D('',#59429,#47011,#47012);
#37498=AXIS2_PLACEMENT_3D('',#59430,#47013,#47014);
#37499=AXIS2_PLACEMENT_3D('',#59431,#47015,#47016);
#37500=AXIS2_PLACEMENT_3D('',#59432,#47017,#47018);
#37501=AXIS2_PLACEMENT_3D('',#59445,#47025,#47026);
#37502=AXIS2_PLACEMENT_3D('',#59451,#47030,#47031);
#37503=AXIS2_PLACEMENT_3D('',#59455,#47034,#47035);
#37504=AXIS2_PLACEMENT_3D('',#59459,#47038,#47039);
#37505=AXIS2_PLACEMENT_3D('',#59463,#47042,#47043);
#37506=AXIS2_PLACEMENT_3D('',#59467,#47046,#47047);
#37507=AXIS2_PLACEMENT_3D('',#59469,#47049,#47050);
#37508=AXIS2_PLACEMENT_3D('',#59470,#47051,#47052);
#37509=AXIS2_PLACEMENT_3D('',#59471,#47053,#47054);
#37510=AXIS2_PLACEMENT_3D('',#59472,#47055,#47056);
#37511=AXIS2_PLACEMENT_3D('',#59476,#47059,#47060);
#37512=AXIS2_PLACEMENT_3D('',#59480,#47063,#47064);
#37513=AXIS2_PLACEMENT_3D('',#59482,#47066,#47067);
#37514=AXIS2_PLACEMENT_3D('',#59484,#47068,#47069);
#37515=AXIS2_PLACEMENT_3D('',#59485,#47070,#47071);
#37516=AXIS2_PLACEMENT_3D('',#59487,#47073,#47074);
#37517=AXIS2_PLACEMENT_3D('',#59492,#47076,#47077);
#37518=AXIS2_PLACEMENT_3D('',#59493,#47078,#47079);
#37519=AXIS2_PLACEMENT_3D('',#59494,#47080,#47081);
#37520=AXIS2_PLACEMENT_3D('',#59498,#47083,#47084);
#37521=AXIS2_PLACEMENT_3D('',#59499,#47085,#47086);
#37522=AXIS2_PLACEMENT_3D('',#59500,#47087,#47088);
#37523=AXIS2_PLACEMENT_3D('',#59503,#47090,#47091);
#37524=AXIS2_PLACEMENT_3D('',#59504,#47092,#47093);
#37525=AXIS2_PLACEMENT_3D('',#59509,#47095,#47096);
#37526=AXIS2_PLACEMENT_3D('',#59510,#47097,#47098);
#37527=AXIS2_PLACEMENT_3D('',#59511,#47099,#47100);
#37528=AXIS2_PLACEMENT_3D('',#59515,#47102,#47103);
#37529=AXIS2_PLACEMENT_3D('',#59516,#47104,#47105);
#37530=AXIS2_PLACEMENT_3D('',#59517,#47106,#47107);
#37531=AXIS2_PLACEMENT_3D('',#59520,#47109,#47110);
#37532=AXIS2_PLACEMENT_3D('',#59521,#47111,#47112);
#37533=AXIS2_PLACEMENT_3D('',#59526,#47114,#47115);
#37534=AXIS2_PLACEMENT_3D('',#59527,#47116,#47117);
#37535=AXIS2_PLACEMENT_3D('',#59528,#47118,#47119);
#37536=AXIS2_PLACEMENT_3D('',#59532,#47121,#47122);
#37537=AXIS2_PLACEMENT_3D('',#59533,#47123,#47124);
#37538=AXIS2_PLACEMENT_3D('',#59534,#47125,#47126);
#37539=AXIS2_PLACEMENT_3D('',#59537,#47128,#47129);
#37540=AXIS2_PLACEMENT_3D('',#59538,#47130,#47131);
#37541=AXIS2_PLACEMENT_3D('',#59541,#47132,#47133);
#37542=AXIS2_PLACEMENT_3D('',#59542,#47134,#47135);
#37543=AXIS2_PLACEMENT_3D('',#59545,#47137,#47138);
#37544=AXIS2_PLACEMENT_3D('',#59546,#47139,#47140);
#37545=AXIS2_PLACEMENT_3D('',#59550,#47142,#47143);
#37546=AXIS2_PLACEMENT_3D('',#59551,#47144,#47145);
#37547=AXIS2_PLACEMENT_3D('',#59552,#47146,#47147);
#37548=AXIS2_PLACEMENT_3D('',#59555,#47149,#47150);
#37549=AXIS2_PLACEMENT_3D('',#59558,#47151,#47152);
#37550=AXIS2_PLACEMENT_3D('',#59559,#47153,#47154);
#37551=AXIS2_PLACEMENT_3D('',#59562,#47156,#47157);
#37552=AXIS2_PLACEMENT_3D('',#59563,#47158,#47159);
#37553=AXIS2_PLACEMENT_3D('',#59567,#47161,#47162);
#37554=AXIS2_PLACEMENT_3D('',#59568,#47163,#47164);
#37555=AXIS2_PLACEMENT_3D('',#59569,#47165,#47166);
#37556=AXIS2_PLACEMENT_3D('',#59572,#47168,#47169);
#37557=AXIS2_PLACEMENT_3D('',#59575,#47170,#47171);
#37558=AXIS2_PLACEMENT_3D('',#59576,#47172,#47173);
#37559=AXIS2_PLACEMENT_3D('',#59579,#47175,#47176);
#37560=AXIS2_PLACEMENT_3D('',#59580,#47177,#47178);
#37561=AXIS2_PLACEMENT_3D('',#59584,#47180,#47181);
#37562=AXIS2_PLACEMENT_3D('',#59585,#47182,#47183);
#37563=AXIS2_PLACEMENT_3D('',#59586,#47184,#47185);
#37564=AXIS2_PLACEMENT_3D('',#59589,#47187,#47188);
#37565=AXIS2_PLACEMENT_3D('',#59592,#47189,#47190);
#37566=AXIS2_PLACEMENT_3D('',#59593,#47191,#47192);
#37567=AXIS2_PLACEMENT_3D('',#59596,#47194,#47195);
#37568=AXIS2_PLACEMENT_3D('',#59597,#47196,#47197);
#37569=AXIS2_PLACEMENT_3D('',#59601,#47199,#47200);
#37570=AXIS2_PLACEMENT_3D('',#59602,#47201,#47202);
#37571=AXIS2_PLACEMENT_3D('',#59603,#47203,#47204);
#37572=AXIS2_PLACEMENT_3D('',#59606,#47206,#47207);
#37573=AXIS2_PLACEMENT_3D('',#59609,#47209,#47210);
#37574=AXIS2_PLACEMENT_3D('',#59612,#47212,#47213);
#37575=AXIS2_PLACEMENT_3D('',#59615,#47215,#47216);
#37576=AXIS2_PLACEMENT_3D('',#59618,#47218,#47219);
#37577=AXIS2_PLACEMENT_3D('',#59621,#47221,#47222);
#37578=AXIS2_PLACEMENT_3D('',#59624,#47224,#47225);
#37579=AXIS2_PLACEMENT_3D('',#59627,#47227,#47228);
#37580=AXIS2_PLACEMENT_3D('',#59630,#47230,#47231);
#37581=AXIS2_PLACEMENT_3D('',#59636,#47235,#47236);
#37582=AXIS2_PLACEMENT_3D('',#59640,#47239,#47240);
#37583=AXIS2_PLACEMENT_3D('',#59646,#47244,#47245);
#37584=AXIS2_PLACEMENT_3D('',#59650,#47248,#47249);
#37585=AXIS2_PLACEMENT_3D('',#59654,#47252,#47253);
#37586=AXIS2_PLACEMENT_3D('',#59658,#47256,#47257);
#37587=AXIS2_PLACEMENT_3D('',#59662,#47260,#47261);
#37588=AXIS2_PLACEMENT_3D('',#59664,#47263,#47264);
#37589=AXIS2_PLACEMENT_3D('',#59684,#47275,#47276);
#37590=AXIS2_PLACEMENT_3D('',#59686,#47277,#47278);
#37591=AXIS2_PLACEMENT_3D('',#59688,#47279,#47280);
#37592=AXIS2_PLACEMENT_3D('',#59689,#47281,#47282);
#37593=AXIS2_PLACEMENT_3D('',#59692,#47284,#47285);
#37594=AXIS2_PLACEMENT_3D('',#59693,#47286,#47287);
#37595=AXIS2_PLACEMENT_3D('',#59696,#47288,#47289);
#37596=AXIS2_PLACEMENT_3D('',#59699,#47291,#47292);
#37597=AXIS2_PLACEMENT_3D('',#59700,#47293,#47294);
#37598=AXIS2_PLACEMENT_3D('',#59701,#47295,#47296);
#37599=AXIS2_PLACEMENT_3D('',#59702,#47297,#47298);
#37600=AXIS2_PLACEMENT_3D('',#59704,#47300,#47301);
#37601=AXIS2_PLACEMENT_3D('',#59708,#47304,#47305);
#37602=AXIS2_PLACEMENT_3D('',#59712,#47308,#47309);
#37603=AXIS2_PLACEMENT_3D('',#59716,#47312,#47313);
#37604=AXIS2_PLACEMENT_3D('',#59720,#47316,#47317);
#37605=AXIS2_PLACEMENT_3D('',#59724,#47320,#47321);
#37606=AXIS2_PLACEMENT_3D('',#59726,#47323,#47324);
#37607=AXIS2_PLACEMENT_3D('',#59727,#47325,#47326);
#37608=AXIS2_PLACEMENT_3D('',#59729,#47328,#47329);
#37609=AXIS2_PLACEMENT_3D('',#59730,#47330,#47331);
#37610=AXIS2_PLACEMENT_3D('',#59731,#47332,#47333);
#37611=AXIS2_PLACEMENT_3D('',#59734,#47334,#47335);
#37612=AXIS2_PLACEMENT_3D('',#59735,#47336,#47337);
#37613=AXIS2_PLACEMENT_3D('',#59738,#47339,#47340);
#37614=AXIS2_PLACEMENT_3D('',#59739,#47341,#47342);
#37615=AXIS2_PLACEMENT_3D('',#59819,#47344,#47345);
#37616=AXIS2_PLACEMENT_3D('',#59822,#47347,#47348);
#37617=AXIS2_PLACEMENT_3D('',#59823,#47349,#47350);
#37618=AXIS2_PLACEMENT_3D('',#59826,#47353,#47354);
#37619=AXIS2_PLACEMENT_3D('',#59827,#47355,#47356);
#37620=AXIS2_PLACEMENT_3D('',#59828,#47357,#47358);
#37621=AXIS2_PLACEMENT_3D('',#59830,#47359,#47360);
#37622=AXIS2_PLACEMENT_3D('',#59833,#47362,#47363);
#37623=AXIS2_PLACEMENT_3D('',#59834,#47364,#47365);
#37624=AXIS2_PLACEMENT_3D('',#59837,#47366,#47367);
#37625=AXIS2_PLACEMENT_3D('',#59838,#47368,#47369);
#37626=AXIS2_PLACEMENT_3D('',#59841,#47371,#47372);
#37627=AXIS2_PLACEMENT_3D('',#59842,#47373,#47374);
#37628=AXIS2_PLACEMENT_3D('',#59867,#47387,#47388);
#37629=AXIS2_PLACEMENT_3D('',#59869,#47389,#47390);
#37630=AXIS2_PLACEMENT_3D('',#59870,#47391,#47392);
#37631=AXIS2_PLACEMENT_3D('',#59872,#47393,#47394);
#37632=AXIS2_PLACEMENT_3D('',#59874,#47396,#47397);
#37633=AXIS2_PLACEMENT_3D('',#59875,#47398,#47399);
#37634=AXIS2_PLACEMENT_3D('',#59878,#47400,#47401);
#37635=AXIS2_PLACEMENT_3D('',#59879,#47402,#47403);
#37636=AXIS2_PLACEMENT_3D('',#59882,#47405,#47406);
#37637=AXIS2_PLACEMENT_3D('',#59883,#47407,#47408);
#37638=AXIS2_PLACEMENT_3D('',#59886,#47409,#47410);
#37639=AXIS2_PLACEMENT_3D('',#59887,#47411,#47412);
#37640=AXIS2_PLACEMENT_3D('',#59890,#47414,#47415);
#37641=AXIS2_PLACEMENT_3D('',#59891,#47416,#47417);
#37642=AXIS2_PLACEMENT_3D('',#59898,#47420,#47421);
#37643=AXIS2_PLACEMENT_3D('',#59900,#47423,#47424);
#37644=AXIS2_PLACEMENT_3D('',#59903,#47425,#47426);
#37645=AXIS2_PLACEMENT_3D('',#59912,#47427,#47428);
#37646=AXIS2_PLACEMENT_3D('',#59914,#47429,#47430);
#37647=AXIS2_PLACEMENT_3D('',#59915,#47431,#47432);
#37648=AXIS2_PLACEMENT_3D('',#59919,#47434,#47435);
#37649=AXIS2_PLACEMENT_3D('',#59991,#47437,#47438);
#37650=AXIS2_PLACEMENT_3D('',#59994,#47439,#47440);
#37651=AXIS2_PLACEMENT_3D('',#59995,#47441,#47442);
#37652=AXIS2_PLACEMENT_3D('',#59998,#47444,#47445);
#37653=AXIS2_PLACEMENT_3D('',#59999,#47446,#47447);
#37654=AXIS2_PLACEMENT_3D('',#60002,#47450,#47451);
#37655=AXIS2_PLACEMENT_3D('',#60015,#47458,#47459);
#37656=AXIS2_PLACEMENT_3D('',#60021,#47463,#47464);
#37657=AXIS2_PLACEMENT_3D('',#60025,#47467,#47468);
#37658=AXIS2_PLACEMENT_3D('',#60029,#47471,#47472);
#37659=AXIS2_PLACEMENT_3D('',#60033,#47475,#47476);
#37660=AXIS2_PLACEMENT_3D('',#60037,#47479,#47480);
#37661=AXIS2_PLACEMENT_3D('',#60039,#47482,#47483);
#37662=AXIS2_PLACEMENT_3D('',#60052,#47490,#47491);
#37663=AXIS2_PLACEMENT_3D('',#60058,#47495,#47496);
#37664=AXIS2_PLACEMENT_3D('',#60062,#47499,#47500);
#37665=AXIS2_PLACEMENT_3D('',#60066,#47503,#47504);
#37666=AXIS2_PLACEMENT_3D('',#60070,#47507,#47508);
#37667=AXIS2_PLACEMENT_3D('',#60074,#47511,#47512);
#37668=AXIS2_PLACEMENT_3D('',#60076,#47514,#47515);
#37669=AXIS2_PLACEMENT_3D('',#60078,#47516,#47517);
#37670=AXIS2_PLACEMENT_3D('',#60079,#47518,#47519);
#37671=AXIS2_PLACEMENT_3D('',#60082,#47520,#47521);
#37672=AXIS2_PLACEMENT_3D('',#60083,#47522,#47523);
#37673=AXIS2_PLACEMENT_3D('',#60085,#47525,#47526);
#37674=AXIS2_PLACEMENT_3D('',#60122,#47528,#47529);
#37675=AXIS2_PLACEMENT_3D('',#60125,#47530,#47531);
#37676=AXIS2_PLACEMENT_3D('',#60126,#47532,#47533);
#37677=AXIS2_PLACEMENT_3D('',#60129,#47535,#47536);
#37678=AXIS2_PLACEMENT_3D('',#60130,#47537,#47538);
#37679=AXIS2_PLACEMENT_3D('',#60131,#47539,#47540);
#37680=AXIS2_PLACEMENT_3D('',#60133,#47541,#47542);
#37681=AXIS2_PLACEMENT_3D('',#60134,#47543,#47544);
#37682=AXIS2_PLACEMENT_3D('',#60137,#47545,#47546);
#37683=AXIS2_PLACEMENT_3D('',#60138,#47547,#47548);
#37684=AXIS2_PLACEMENT_3D('',#60140,#47550,#47551);
#37685=AXIS2_PLACEMENT_3D('',#60153,#47558,#47559);
#37686=AXIS2_PLACEMENT_3D('',#60159,#47563,#47564);
#37687=AXIS2_PLACEMENT_3D('',#60163,#47567,#47568);
#37688=AXIS2_PLACEMENT_3D('',#60167,#47571,#47572);
#37689=AXIS2_PLACEMENT_3D('',#60171,#47575,#47576);
#37690=AXIS2_PLACEMENT_3D('',#60175,#47579,#47580);
#37691=AXIS2_PLACEMENT_3D('',#60177,#47582,#47583);
#37692=AXIS2_PLACEMENT_3D('',#60190,#47590,#47591);
#37693=AXIS2_PLACEMENT_3D('',#60196,#47595,#47596);
#37694=AXIS2_PLACEMENT_3D('',#60200,#47599,#47600);
#37695=AXIS2_PLACEMENT_3D('',#60204,#47603,#47604);
#37696=AXIS2_PLACEMENT_3D('',#60208,#47607,#47608);
#37697=AXIS2_PLACEMENT_3D('',#60212,#47611,#47612);
#37698=AXIS2_PLACEMENT_3D('',#60214,#47614,#47615);
#37699=AXIS2_PLACEMENT_3D('',#60216,#47616,#47617);
#37700=AXIS2_PLACEMENT_3D('',#60217,#47618,#47619);
#37701=AXIS2_PLACEMENT_3D('',#60220,#47620,#47621);
#37702=AXIS2_PLACEMENT_3D('',#60221,#47622,#47623);
#37703=AXIS2_PLACEMENT_3D('',#60223,#47625,#47626);
#37704=AXIS2_PLACEMENT_3D('',#60260,#47628,#47629);
#37705=AXIS2_PLACEMENT_3D('',#60263,#47630,#47631);
#37706=AXIS2_PLACEMENT_3D('',#60264,#47632,#47633);
#37707=AXIS2_PLACEMENT_3D('',#60267,#47635,#47636);
#37708=AXIS2_PLACEMENT_3D('',#60268,#47637,#47638);
#37709=AXIS2_PLACEMENT_3D('',#60269,#47639,#47640);
#37710=AXIS2_PLACEMENT_3D('',#60271,#47641,#47642);
#37711=AXIS2_PLACEMENT_3D('',#60272,#47643,#47644);
#37712=AXIS2_PLACEMENT_3D('',#60275,#47645,#47646);
#37713=AXIS2_PLACEMENT_3D('',#60276,#47647,#47648);
#37714=AXIS2_PLACEMENT_3D('',#60278,#47650,#47651);
#37715=AXIS2_PLACEMENT_3D('',#60315,#47653,#47654);
#37716=AXIS2_PLACEMENT_3D('',#60318,#47656,#47657);
#37717=AXIS2_PLACEMENT_3D('',#60319,#47658,#47659);
#37718=AXIS2_PLACEMENT_3D('',#60320,#47660,#47661);
#37719=AXIS2_PLACEMENT_3D('',#60322,#47663,#47664);
#37720=AXIS2_PLACEMENT_3D('',#60324,#47666,#47667);
#37721=AXIS2_PLACEMENT_3D('',#60326,#47668,#47669);
#37722=AXIS2_PLACEMENT_3D('',#60327,#47670,#47671);
#37723=AXIS2_PLACEMENT_3D('',#60329,#47673,#47674);
#37724=AXIS2_PLACEMENT_3D('',#60366,#47676,#47677);
#37725=AXIS2_PLACEMENT_3D('',#60369,#47678,#47679);
#37726=AXIS2_PLACEMENT_3D('',#60370,#47680,#47681);
#37727=AXIS2_PLACEMENT_3D('',#60373,#47683,#47684);
#37728=AXIS2_PLACEMENT_3D('',#60374,#47685,#47686);
#37729=AXIS2_PLACEMENT_3D('',#60376,#47688,#47689);
#37730=AXIS2_PLACEMENT_3D('',#60381,#47690,#47691);
#37731=AXIS2_PLACEMENT_3D('',#60386,#47692,#47693);
#37732=AXIS2_PLACEMENT_3D('',#60387,#47694,#47695);
#37733=AXIS2_PLACEMENT_3D('',#60389,#47696,#47697);
#37734=AXIS2_PLACEMENT_3D('',#60391,#47699,#47700);
#37735=AXIS2_PLACEMENT_3D('',#60393,#47701,#47702);
#37736=AXIS2_PLACEMENT_3D('',#60394,#47703,#47704);
#37737=AXIS2_PLACEMENT_3D('',#60396,#47705,#47706);
#37738=AXIS2_PLACEMENT_3D('',#60397,#47707,#47708);
#37739=AXIS2_PLACEMENT_3D('',#60399,#47710,#47711);
#37740=AXIS2_PLACEMENT_3D('',#60402,#47713,#47714);
#37741=AXIS2_PLACEMENT_3D('',#60403,#47715,#47716);
#37742=AXIS2_PLACEMENT_3D('',#60404,#47717,#47718);
#37743=AXIS2_PLACEMENT_3D('',#60406,#47719,#47720);
#37744=AXIS2_PLACEMENT_3D('',#60407,#47721,#47722);
#37745=AXIS2_PLACEMENT_3D('',#60409,#47724,#47725);
#37746=AXIS2_PLACEMENT_3D('',#60412,#47726,#47727);
#37747=AXIS2_PLACEMENT_3D('',#60416,#47729,#47730);
#37748=AXIS2_PLACEMENT_3D('',#60420,#47732,#47733);
#37749=AXIS2_PLACEMENT_3D('',#60424,#47735,#47736);
#37750=AXIS2_PLACEMENT_3D('',#60428,#47738,#47739);
#37751=AXIS2_PLACEMENT_3D('',#60432,#47741,#47742);
#37752=AXIS2_PLACEMENT_3D('',#60434,#47744,#47745);
#37753=AXIS2_PLACEMENT_3D('',#60442,#47746,#47747);
#37754=AXIS2_PLACEMENT_3D('',#60453,#47750,#47751);
#37755=AXIS2_PLACEMENT_3D('',#60462,#47753,#47754);
#37756=AXIS2_PLACEMENT_3D('',#60470,#47755,#47756);
#37757=AXIS2_PLACEMENT_3D('',#60474,#47757,#47758);
#37758=AXIS2_PLACEMENT_3D('',#60475,#47759,#47760);
#37759=AXIS2_PLACEMENT_3D('',#60483,#47761,#47762);
#37760=AXIS2_PLACEMENT_3D('',#60487,#47763,#47764);
#37761=AXIS2_PLACEMENT_3D('',#60489,#47766,#47767);
#37762=AXIS2_PLACEMENT_3D('',#60491,#47769,#47770);
#37763=AXIS2_PLACEMENT_3D('',#60493,#47772,#47773);
#37764=AXIS2_PLACEMENT_3D('',#60494,#47774,#47775);
#37765=AXIS2_PLACEMENT_3D('',#60497,#47776,#47777);
#37766=AXIS2_PLACEMENT_3D('',#60501,#47779,#47780);
#37767=AXIS2_PLACEMENT_3D('',#60505,#47782,#47783);
#37768=AXIS2_PLACEMENT_3D('',#60509,#47785,#47786);
#37769=AXIS2_PLACEMENT_3D('',#60513,#47788,#47789);
#37770=AXIS2_PLACEMENT_3D('',#60517,#47791,#47792);
#37771=AXIS2_PLACEMENT_3D('',#60519,#47794,#47795);
#37772=AXIS2_PLACEMENT_3D('',#60527,#47796,#47797);
#37773=AXIS2_PLACEMENT_3D('',#60538,#47800,#47801);
#37774=AXIS2_PLACEMENT_3D('',#60547,#47803,#47804);
#37775=AXIS2_PLACEMENT_3D('',#60555,#47805,#47806);
#37776=AXIS2_PLACEMENT_3D('',#60559,#47807,#47808);
#37777=AXIS2_PLACEMENT_3D('',#60560,#47809,#47810);
#37778=AXIS2_PLACEMENT_3D('',#60568,#47811,#47812);
#37779=AXIS2_PLACEMENT_3D('',#60572,#47813,#47814);
#37780=AXIS2_PLACEMENT_3D('',#60574,#47816,#47817);
#37781=AXIS2_PLACEMENT_3D('',#60576,#47819,#47820);
#37782=AXIS2_PLACEMENT_3D('',#60578,#47822,#47823);
#37783=AXIS2_PLACEMENT_3D('',#60579,#47824,#47825);
#37784=AXIS2_PLACEMENT_3D('',#60581,#47826,#47827);
#37785=AXIS2_PLACEMENT_3D('',#60582,#47828,#47829);
#37786=AXIS2_PLACEMENT_3D('',#60584,#47830,#47831);
#37787=AXIS2_PLACEMENT_3D('',#60585,#47832,#47833);
#37788=AXIS2_PLACEMENT_3D('',#60587,#47834,#47835);
#37789=AXIS2_PLACEMENT_3D('',#60588,#47836,#47837);
#37790=AXIS2_PLACEMENT_3D('',#60590,#47838,#47839);
#37791=AXIS2_PLACEMENT_3D('',#60593,#47841,#47842);
#37792=AXIS2_PLACEMENT_3D('',#60594,#47843,#47844);
#37793=AXIS2_PLACEMENT_3D('',#60596,#47845,#47846);
#37794=AXIS2_PLACEMENT_3D('',#60599,#47848,#47849);
#37795=AXIS2_PLACEMENT_3D('',#60600,#47850,#47851);
#37796=AXIS2_PLACEMENT_3D('',#60602,#47852,#47853);
#37797=AXIS2_PLACEMENT_3D('',#60604,#47855,#47856);
#37798=AXIS2_PLACEMENT_3D('',#60606,#47857,#47858);
#37799=AXIS2_PLACEMENT_3D('',#60609,#47860,#47861);
#37800=AXIS2_PLACEMENT_3D('',#60610,#47862,#47863);
#37801=AXIS2_PLACEMENT_3D('',#60612,#47864,#47865);
#37802=AXIS2_PLACEMENT_3D('',#60615,#47867,#47868);
#37803=AXIS2_PLACEMENT_3D('',#60616,#47869,#47870);
#37804=AXIS2_PLACEMENT_3D('',#60618,#47871,#47872);
#37805=AXIS2_PLACEMENT_3D('',#60621,#47874,#47875);
#37806=AXIS2_PLACEMENT_3D('',#60622,#47876,#47877);
#37807=AXIS2_PLACEMENT_3D('',#60624,#47878,#47879);
#37808=AXIS2_PLACEMENT_3D('',#60627,#47881,#47882);
#37809=AXIS2_PLACEMENT_3D('',#60628,#47883,#47884);
#37810=AXIS2_PLACEMENT_3D('',#60631,#47885,#47886);
#37811=AXIS2_PLACEMENT_3D('',#60633,#47887,#47888);
#37812=AXIS2_PLACEMENT_3D('',#60637,#47890,#47891);
#37813=AXIS2_PLACEMENT_3D('',#60639,#47892,#47893);
#37814=AXIS2_PLACEMENT_3D('',#60641,#47894,#47895);
#37815=AXIS2_PLACEMENT_3D('',#60644,#47897,#47898);
#37816=AXIS2_PLACEMENT_3D('',#60645,#47899,#47900);
#37817=AXIS2_PLACEMENT_3D('',#60654,#47905,#47906);
#37818=AXIS2_PLACEMENT_3D('',#60656,#47907,#47908);
#37819=AXIS2_PLACEMENT_3D('',#60659,#47910,#47911);
#37820=AXIS2_PLACEMENT_3D('',#60660,#47912,#47913);
#37821=AXIS2_PLACEMENT_3D('',#60662,#47914,#47915);
#37822=AXIS2_PLACEMENT_3D('',#60665,#47917,#47918);
#37823=AXIS2_PLACEMENT_3D('',#60666,#47919,#47920);
#37824=AXIS2_PLACEMENT_3D('',#60668,#47921,#47922);
#37825=AXIS2_PLACEMENT_3D('',#60671,#47924,#47925);
#37826=AXIS2_PLACEMENT_3D('',#60672,#47926,#47927);
#37827=AXIS2_PLACEMENT_3D('',#60678,#47931,#47932);
#37828=AXIS2_PLACEMENT_3D('',#60680,#47933,#47934);
#37829=AXIS2_PLACEMENT_3D('',#60683,#47936,#47937);
#37830=AXIS2_PLACEMENT_3D('',#60684,#47938,#47939);
#37831=AXIS2_PLACEMENT_3D('',#60686,#47940,#47941);
#37832=AXIS2_PLACEMENT_3D('',#60689,#47943,#47944);
#37833=AXIS2_PLACEMENT_3D('',#60690,#47945,#47946);
#37834=AXIS2_PLACEMENT_3D('',#60691,#47947,#47948);
#37835=AXIS2_PLACEMENT_3D('',#60692,#47949,#47950);
#37836=AXIS2_PLACEMENT_3D('',#60693,#47951,#47952);
#37837=AXIS2_PLACEMENT_3D('',#60694,#47953,#47954);
#37838=AXIS2_PLACEMENT_3D('',#60703,#47959,#47960);
#37839=AXIS2_PLACEMENT_3D('',#60705,#47961,#47962);
#37840=AXIS2_PLACEMENT_3D('',#60708,#47964,#47965);
#37841=AXIS2_PLACEMENT_3D('',#60709,#47966,#47967);
#37842=AXIS2_PLACEMENT_3D('',#60711,#47968,#47969);
#37843=AXIS2_PLACEMENT_3D('',#60714,#47971,#47972);
#37844=AXIS2_PLACEMENT_3D('',#60715,#47973,#47974);
#37845=AXIS2_PLACEMENT_3D('',#60717,#47975,#47976);
#37846=AXIS2_PLACEMENT_3D('',#60720,#47978,#47979);
#37847=AXIS2_PLACEMENT_3D('',#60721,#47980,#47981);
#37848=AXIS2_PLACEMENT_3D('',#60727,#47985,#47986);
#37849=AXIS2_PLACEMENT_3D('',#60729,#47987,#47988);
#37850=AXIS2_PLACEMENT_3D('',#60732,#47990,#47991);
#37851=AXIS2_PLACEMENT_3D('',#60733,#47992,#47993);
#37852=AXIS2_PLACEMENT_3D('',#60735,#47994,#47995);
#37853=AXIS2_PLACEMENT_3D('',#60738,#47997,#47998);
#37854=AXIS2_PLACEMENT_3D('',#60739,#47999,#48000);
#37855=AXIS2_PLACEMENT_3D('',#60740,#48001,#48002);
#37856=AXIS2_PLACEMENT_3D('',#60741,#48003,#48004);
#37857=AXIS2_PLACEMENT_3D('',#60742,#48005,#48006);
#37858=AXIS2_PLACEMENT_3D('',#60743,#48007,#48008);
#37859=AXIS2_PLACEMENT_3D('',#60752,#48013,#48014);
#37860=AXIS2_PLACEMENT_3D('',#60754,#48015,#48016);
#37861=AXIS2_PLACEMENT_3D('',#60757,#48018,#48019);
#37862=AXIS2_PLACEMENT_3D('',#60758,#48020,#48021);
#37863=AXIS2_PLACEMENT_3D('',#60760,#48022,#48023);
#37864=AXIS2_PLACEMENT_3D('',#60763,#48025,#48026);
#37865=AXIS2_PLACEMENT_3D('',#60764,#48027,#48028);
#37866=AXIS2_PLACEMENT_3D('',#60766,#48029,#48030);
#37867=AXIS2_PLACEMENT_3D('',#60769,#48032,#48033);
#37868=AXIS2_PLACEMENT_3D('',#60770,#48034,#48035);
#37869=AXIS2_PLACEMENT_3D('',#60776,#48039,#48040);
#37870=AXIS2_PLACEMENT_3D('',#60778,#48041,#48042);
#37871=AXIS2_PLACEMENT_3D('',#60781,#48044,#48045);
#37872=AXIS2_PLACEMENT_3D('',#60782,#48046,#48047);
#37873=AXIS2_PLACEMENT_3D('',#60784,#48048,#48049);
#37874=AXIS2_PLACEMENT_3D('',#60787,#48051,#48052);
#37875=AXIS2_PLACEMENT_3D('',#60788,#48053,#48054);
#37876=AXIS2_PLACEMENT_3D('',#60789,#48055,#48056);
#37877=AXIS2_PLACEMENT_3D('',#60790,#48057,#48058);
#37878=AXIS2_PLACEMENT_3D('',#60791,#48059,#48060);
#37879=AXIS2_PLACEMENT_3D('',#60792,#48061,#48062);
#37880=AXIS2_PLACEMENT_3D('',#60795,#48064,#48065);
#37881=AXIS2_PLACEMENT_3D('',#60796,#48066,#48067);
#37882=AXIS2_PLACEMENT_3D('',#60799,#48069,#48070);
#37883=AXIS2_PLACEMENT_3D('',#60800,#48071,#48072);
#37884=AXIS2_PLACEMENT_3D('',#60803,#48074,#48075);
#37885=AXIS2_PLACEMENT_3D('',#60804,#48076,#48077);
#37886=AXIS2_PLACEMENT_3D('',#60807,#48078,#48079);
#37887=AXIS2_PLACEMENT_3D('',#60809,#48080,#48081);
#37888=AXIS2_PLACEMENT_3D('',#60811,#48082,#48083);
#37889=AXIS2_PLACEMENT_3D('',#60812,#48084,#48085);
#37890=AXIS2_PLACEMENT_3D('',#60813,#48086,#48087);
#37891=AXIS2_PLACEMENT_3D('',#60815,#48089,#48090);
#37892=AXIS2_PLACEMENT_3D('',#60818,#48091,#48092);
#37893=AXIS2_PLACEMENT_3D('',#60820,#48093,#48094);
#37894=AXIS2_PLACEMENT_3D('',#60822,#48095,#48096);
#37895=AXIS2_PLACEMENT_3D('',#60823,#48097,#48098);
#37896=AXIS2_PLACEMENT_3D('',#60824,#48099,#48100);
#37897=AXIS2_PLACEMENT_3D('',#60826,#48102,#48103);
#37898=AXIS2_PLACEMENT_3D('',#60829,#48104,#48105);
#37899=AXIS2_PLACEMENT_3D('',#60831,#48106,#48107);
#37900=AXIS2_PLACEMENT_3D('',#60833,#48108,#48109);
#37901=AXIS2_PLACEMENT_3D('',#60834,#48110,#48111);
#37902=AXIS2_PLACEMENT_3D('',#60835,#48112,#48113);
#37903=AXIS2_PLACEMENT_3D('',#60837,#48115,#48116);
#37904=AXIS2_PLACEMENT_3D('',#60844,#48119,#48120);
#37905=AXIS2_PLACEMENT_3D('',#60849,#48123,#48124);
#37906=AXIS2_PLACEMENT_3D('',#60850,#48125,#48126);
#37907=AXIS2_PLACEMENT_3D('',#60855,#48128,#48129);
#37908=AXIS2_PLACEMENT_3D('',#60861,#48132,#48133);
#37909=AXIS2_PLACEMENT_3D('',#60863,#48135,#48136);
#37910=AXIS2_PLACEMENT_3D('',#60868,#48138,#48139);
#37911=AXIS2_PLACEMENT_3D('',#60874,#48142,#48143);
#37912=AXIS2_PLACEMENT_3D('',#60877,#48145,#48146);
#37913=AXIS2_PLACEMENT_3D('',#60878,#48147,#48148);
#37914=AXIS2_PLACEMENT_3D('',#60880,#48149,#48150);
#37915=AXIS2_PLACEMENT_3D('',#60884,#48152,#48153);
#37916=AXIS2_PLACEMENT_3D('',#60885,#48154,#48155);
#37917=AXIS2_PLACEMENT_3D('',#60886,#48156,#48157);
#37918=AXIS2_PLACEMENT_3D('',#60892,#48161,#48162);
#37919=AXIS2_PLACEMENT_3D('',#60898,#48166,#48167);
#37920=AXIS2_PLACEMENT_3D('',#60904,#48171,#48172);
#37921=AXIS2_PLACEMENT_3D('',#60910,#48176,#48177);
#37922=AXIS2_PLACEMENT_3D('',#60922,#48185,#48186);
#37923=AXIS2_PLACEMENT_3D('',#60925,#48188,#48189);
#37924=AXIS2_PLACEMENT_3D('',#60926,#48190,#48191);
#37925=AXIS2_PLACEMENT_3D('',#60936,#48198,#48199);
#37926=AXIS2_PLACEMENT_3D('',#60939,#48201,#48202);
#37927=AXIS2_PLACEMENT_3D('',#60940,#48203,#48204);
#37928=AXIS2_PLACEMENT_3D('',#60953,#48212,#48213);
#37929=AXIS2_PLACEMENT_3D('',#60955,#48214,#48215);
#37930=AXIS2_PLACEMENT_3D('',#60958,#48217,#48218);
#37931=AXIS2_PLACEMENT_3D('',#60959,#48219,#48220);
#37932=AXIS2_PLACEMENT_3D('',#60964,#48222,#48223);
#37933=AXIS2_PLACEMENT_3D('',#60968,#48225,#48226);
#37934=AXIS2_PLACEMENT_3D('',#60978,#48233,#48234);
#37935=AXIS2_PLACEMENT_3D('',#60979,#48235,#48236);
#37936=AXIS2_PLACEMENT_3D('',#60980,#48237,#48238);
#37937=AXIS2_PLACEMENT_3D('',#60986,#48241,#48242);
#37938=AXIS2_PLACEMENT_3D('',#60991,#48245,#48246);
#37939=AXIS2_PLACEMENT_3D('',#60996,#48249,#48250);
#37940=AXIS2_PLACEMENT_3D('',#61000,#48253,#48254);
#37941=AXIS2_PLACEMENT_3D('',#61001,#48255,#48256);
#37942=AXIS2_PLACEMENT_3D('',#61005,#48259,#48260);
#37943=AXIS2_PLACEMENT_3D('',#61007,#48261,#48262);
#37944=AXIS2_PLACEMENT_3D('',#61009,#48264,#48265);
#37945=AXIS2_PLACEMENT_3D('',#61011,#48267,#48268);
#37946=AXIS2_PLACEMENT_3D('',#61013,#48270,#48271);
#37947=AXIS2_PLACEMENT_3D('',#61015,#48273,#48274);
#37948=AXIS2_PLACEMENT_3D('',#61016,#48275,#48276);
#37949=AXIS2_PLACEMENT_3D('',#61018,#48278,#48279);
#37950=AXIS2_PLACEMENT_3D('',#61020,#48281,#48282);
#37951=AXIS2_PLACEMENT_3D('',#61021,#48283,#48284);
#37952=AXIS2_PLACEMENT_3D('',#61023,#48286,#48287);
#37953=AXIS2_PLACEMENT_3D('',#61025,#48289,#48290);
#37954=AXIS2_PLACEMENT_3D('',#61026,#48291,#48292);
#37955=AXIS2_PLACEMENT_3D('',#61027,#48293,#48294);
#37956=AXIS2_PLACEMENT_3D('',#61028,#48295,#48296);
#37957=AXIS2_PLACEMENT_3D('',#61029,#48297,#48298);
#37958=AXIS2_PLACEMENT_3D('',#61030,#48299,#48300);
#37959=AXIS2_PLACEMENT_3D('',#61031,#48301,#48302);
#37960=AXIS2_PLACEMENT_3D('',#61034,#48303,#48304);
#37961=AXIS2_PLACEMENT_3D('',#61038,#48306,#48307);
#37962=AXIS2_PLACEMENT_3D('',#61040,#48309,#48310);
#37963=AXIS2_PLACEMENT_3D('',#61046,#48314,#48315);
#37964=AXIS2_PLACEMENT_3D('',#61048,#48316,#48317);
#37965=AXIS2_PLACEMENT_3D('',#61051,#48319,#48320);
#37966=AXIS2_PLACEMENT_3D('',#61052,#48321,#48322);
#37967=AXIS2_PLACEMENT_3D('',#61054,#48323,#48324);
#37968=AXIS2_PLACEMENT_3D('',#61057,#48326,#48327);
#37969=AXIS2_PLACEMENT_3D('',#61058,#48328,#48329);
#37970=AXIS2_PLACEMENT_3D('',#61060,#48330,#48331);
#37971=AXIS2_PLACEMENT_3D('',#61063,#48333,#48334);
#37972=AXIS2_PLACEMENT_3D('',#61064,#48335,#48336);
#37973=AXIS2_PLACEMENT_3D('',#61070,#48340,#48341);
#37974=AXIS2_PLACEMENT_3D('',#61072,#48342,#48343);
#37975=AXIS2_PLACEMENT_3D('',#61075,#48345,#48346);
#37976=AXIS2_PLACEMENT_3D('',#61076,#48347,#48348);
#37977=AXIS2_PLACEMENT_3D('',#61077,#48349,#48350);
#37978=AXIS2_PLACEMENT_3D('',#61078,#48351,#48352);
#37979=AXIS2_PLACEMENT_3D('',#61079,#48353,#48354);
#37980=AXIS2_PLACEMENT_3D('',#61080,#48355,#48356);
#37981=AXIS2_PLACEMENT_3D('',#61089,#48361,#48362);
#37982=AXIS2_PLACEMENT_3D('',#61091,#48363,#48364);
#37983=AXIS2_PLACEMENT_3D('',#61094,#48366,#48367);
#37984=AXIS2_PLACEMENT_3D('',#61095,#48368,#48369);
#37985=AXIS2_PLACEMENT_3D('',#61097,#48370,#48371);
#37986=AXIS2_PLACEMENT_3D('',#61100,#48373,#48374);
#37987=AXIS2_PLACEMENT_3D('',#61101,#48375,#48376);
#37988=AXIS2_PLACEMENT_3D('',#61103,#48377,#48378);
#37989=AXIS2_PLACEMENT_3D('',#61106,#48380,#48381);
#37990=AXIS2_PLACEMENT_3D('',#61107,#48382,#48383);
#37991=AXIS2_PLACEMENT_3D('',#61113,#48387,#48388);
#37992=AXIS2_PLACEMENT_3D('',#61115,#48389,#48390);
#37993=AXIS2_PLACEMENT_3D('',#61118,#48392,#48393);
#37994=AXIS2_PLACEMENT_3D('',#61119,#48394,#48395);
#37995=AXIS2_PLACEMENT_3D('',#61121,#48396,#48397);
#37996=AXIS2_PLACEMENT_3D('',#61124,#48399,#48400);
#37997=AXIS2_PLACEMENT_3D('',#61125,#48401,#48402);
#37998=AXIS2_PLACEMENT_3D('',#61126,#48403,#48404);
#37999=AXIS2_PLACEMENT_3D('',#61127,#48405,#48406);
#38000=AXIS2_PLACEMENT_3D('',#61128,#48407,#48408);
#38001=AXIS2_PLACEMENT_3D('',#61129,#48409,#48410);
#38002=AXIS2_PLACEMENT_3D('',#61132,#48411,#48412);
#38003=AXIS2_PLACEMENT_3D('',#61136,#48414,#48415);
#38004=AXIS2_PLACEMENT_3D('',#61138,#48417,#48418);
#38005=AXIS2_PLACEMENT_3D('',#61140,#48419,#48420);
#38006=AXIS2_PLACEMENT_3D('',#61143,#48422,#48423);
#38007=AXIS2_PLACEMENT_3D('',#61144,#48424,#48425);
#38008=AXIS2_PLACEMENT_3D('',#61150,#48429,#48430);
#38009=AXIS2_PLACEMENT_3D('',#61152,#48431,#48432);
#38010=AXIS2_PLACEMENT_3D('',#61155,#48434,#48435);
#38011=AXIS2_PLACEMENT_3D('',#61156,#48436,#48437);
#38012=AXIS2_PLACEMENT_3D('',#61158,#48438,#48439);
#38013=AXIS2_PLACEMENT_3D('',#61161,#48441,#48442);
#38014=AXIS2_PLACEMENT_3D('',#61162,#48443,#48444);
#38015=AXIS2_PLACEMENT_3D('',#61164,#48445,#48446);
#38016=AXIS2_PLACEMENT_3D('',#61167,#48448,#48449);
#38017=AXIS2_PLACEMENT_3D('',#61168,#48450,#48451);
#38018=AXIS2_PLACEMENT_3D('',#61174,#48455,#48456);
#38019=AXIS2_PLACEMENT_3D('',#61175,#48457,#48458);
#38020=AXIS2_PLACEMENT_3D('',#61176,#48459,#48460);
#38021=AXIS2_PLACEMENT_3D('',#61177,#48461,#48462);
#38022=AXIS2_PLACEMENT_3D('',#61178,#48463,#48464);
#38023=AXIS2_PLACEMENT_3D('',#61181,#48465,#48466);
#38024=AXIS2_PLACEMENT_3D('',#61185,#48468,#48469);
#38025=AXIS2_PLACEMENT_3D('',#61187,#48471,#48472);
#38026=AXIS2_PLACEMENT_3D('',#61189,#48473,#48474);
#38027=AXIS2_PLACEMENT_3D('',#61192,#48476,#48477);
#38028=AXIS2_PLACEMENT_3D('',#61193,#48478,#48479);
#38029=AXIS2_PLACEMENT_3D('',#61199,#48483,#48484);
#38030=AXIS2_PLACEMENT_3D('',#61201,#48485,#48486);
#38031=AXIS2_PLACEMENT_3D('',#61204,#48488,#48489);
#38032=AXIS2_PLACEMENT_3D('',#61205,#48490,#48491);
#38033=AXIS2_PLACEMENT_3D('',#61207,#48492,#48493);
#38034=AXIS2_PLACEMENT_3D('',#61210,#48495,#48496);
#38035=AXIS2_PLACEMENT_3D('',#61211,#48497,#48498);
#38036=AXIS2_PLACEMENT_3D('',#61213,#48499,#48500);
#38037=AXIS2_PLACEMENT_3D('',#61216,#48502,#48503);
#38038=AXIS2_PLACEMENT_3D('',#61217,#48504,#48505);
#38039=AXIS2_PLACEMENT_3D('',#61223,#48509,#48510);
#38040=AXIS2_PLACEMENT_3D('',#61224,#48511,#48512);
#38041=AXIS2_PLACEMENT_3D('',#61225,#48513,#48514);
#38042=AXIS2_PLACEMENT_3D('',#61226,#48515,#48516);
#38043=AXIS2_PLACEMENT_3D('',#61227,#48517,#48518);
#38044=AXIS2_PLACEMENT_3D('',#61230,#48519,#48520);
#38045=AXIS2_PLACEMENT_3D('',#61233,#48523,#48524);
#38046=AXIS2_PLACEMENT_3D('',#61235,#48525,#48526);
#38047=AXIS2_PLACEMENT_3D('',#61237,#48528,#48529);
#38048=AXIS2_PLACEMENT_3D('',#61241,#48532,#48533);
#38049=AXIS2_PLACEMENT_3D('',#61243,#48534,#48535);
#38050=AXIS2_PLACEMENT_3D('',#61245,#48537,#48538);
#38051=AXIS2_PLACEMENT_3D('',#61247,#48539,#48540);
#38052=AXIS2_PLACEMENT_3D('',#61249,#48542,#48543);
#38053=AXIS2_PLACEMENT_3D('',#61251,#48544,#48545);
#38054=AXIS2_PLACEMENT_3D('',#61253,#48547,#48548);
#38055=AXIS2_PLACEMENT_3D('',#61255,#48549,#48550);
#38056=AXIS2_PLACEMENT_3D('',#61257,#48552,#48553);
#38057=AXIS2_PLACEMENT_3D('',#61259,#48555,#48556);
#38058=AXIS2_PLACEMENT_3D('',#61261,#48557,#48558);
#38059=AXIS2_PLACEMENT_3D('',#61262,#48559,#48560);
#38060=AXIS2_PLACEMENT_3D('',#61263,#48561,#48562);
#38061=AXIS2_PLACEMENT_3D('',#61280,#48571,#48572);
#38062=AXIS2_PLACEMENT_3D('',#61283,#48575,#48576);
#38063=AXIS2_PLACEMENT_3D('',#61286,#48579,#48580);
#38064=AXIS2_PLACEMENT_3D('',#61287,#48581,#48582);
#38065=AXIS2_PLACEMENT_3D('',#61290,#48585,#48586);
#38066=AXIS2_PLACEMENT_3D('',#61292,#48588,#48589);
#38067=AXIS2_PLACEMENT_3D('',#61293,#48590,#48591);
#38068=AXIS2_PLACEMENT_3D('',#61295,#48593,#48594);
#38069=AXIS2_PLACEMENT_3D('',#61296,#48595,#48596);
#38070=AXIS2_PLACEMENT_3D('',#61297,#48597,#48598);
#38071=AXIS2_PLACEMENT_3D('',#61298,#48599,#48600);
#38072=AXIS2_PLACEMENT_3D('',#61301,#48601,#48602);
#38073=AXIS2_PLACEMENT_3D('',#61302,#48603,#48604);
#38074=AXIS2_PLACEMENT_3D('',#61305,#48606,#48607);
#38075=AXIS2_PLACEMENT_3D('',#61306,#48608,#48609);
#38076=AXIS2_PLACEMENT_3D('',#61310,#48611,#48612);
#38077=AXIS2_PLACEMENT_3D('',#61311,#48613,#48614);
#38078=AXIS2_PLACEMENT_3D('',#61312,#48615,#48616);
#38079=AXIS2_PLACEMENT_3D('',#61314,#48618,#48619);
#38080=AXIS2_PLACEMENT_3D('',#61323,#48624,#48625);
#38081=AXIS2_PLACEMENT_3D('',#61329,#48629,#48630);
#38082=AXIS2_PLACEMENT_3D('',#61335,#48634,#48635);
#38083=AXIS2_PLACEMENT_3D('',#61341,#48639,#48640);
#38084=AXIS2_PLACEMENT_3D('',#61347,#48644,#48645);
#38085=AXIS2_PLACEMENT_3D('',#61349,#48647,#48648);
#38086=AXIS2_PLACEMENT_3D('',#61351,#48650,#48651);
#46290=DIRECTION('axis',(0.,0.,1.));
#46291=DIRECTION('refdir',(1.,0.,0.));
#46292=DIRECTION('center_axis',(-6.49090813559456E-14,1.,-2.55622388633908E-14));
#46293=DIRECTION('ref_axis',(0.581108581114938,5.85224396950113E-14,0.813826036051062));
#46294=DIRECTION('center_axis',(-7.0376604876213E-14,1.,-8.61946552381524E-15));
#46295=DIRECTION('ref_axis',(-2.74761886345665E-15,8.61946552381505E-15,
1.));
#46296=DIRECTION('center_axis',(-7.0376604876213E-14,1.,-8.61946552381524E-15));
#46297=DIRECTION('ref_axis',(-2.74761886345665E-15,8.61946552381505E-15,
1.));
#46298=DIRECTION('',(0.410905818312113,-0.707106781186504,0.575461908797893));
#46299=DIRECTION('center_axis',(6.80591214965025E-14,-1.,9.9941788598046E-15));
#46300=DIRECTION('ref_axis',(0.581108581114922,4.76832624898209E-14,0.813826036051073));
#46301=DIRECTION('center_axis',(6.76186946307289E-14,-1.,8.61946552381525E-15));
#46302=DIRECTION('ref_axis',(2.76820162751153E-15,8.61946552381544E-15,
1.));
#46303=DIRECTION('center_axis',(-6.65083299171228E-14,1.,-9.75928747178892E-15));
#46304=DIRECTION('ref_axis',(0.581108581114964,4.65909234683137E-14,0.813826036051043));
#46305=DIRECTION('',(-0.503254793602722,0.499999999999961,-0.704794021481398));
#46306=DIRECTION('center_axis',(6.76186946307289E-14,-1.,8.61946552381525E-15));
#46307=DIRECTION('ref_axis',(8.28402211847971E-15,8.61946552381581E-15,
1.));
#46308=DIRECTION('center_axis',(6.76186946307289E-14,-1.,8.61946552381525E-15));
#46309=DIRECTION('ref_axis',(8.28402211847971E-15,8.61946552381581E-15,
1.));
#46310=DIRECTION('center_axis',(-6.76186946307289E-14,1.,-8.61946552381525E-15));
#46311=DIRECTION('ref_axis',(-2.76820162751153E-15,-8.61946552381544E-15,
-1.));
#46312=DIRECTION('',(-6.76186946307289E-14,1.,-8.61946552381525E-15));
#46313=DIRECTION('center_axis',(-6.76186946307289E-14,1.,-8.61946552381525E-15));
#46314=DIRECTION('ref_axis',(-2.76820162751153E-15,-8.61946552381544E-15,
-1.));
#46315=DIRECTION('center_axis',(7.67012022460283E-14,-1.,8.61946552381523E-15));
#46316=DIRECTION('ref_axis',(-7.30945543516121E-15,-8.61946552381579E-15,
-1.));
#46317=DIRECTION('',(6.76186946307289E-14,-1.,8.61946552381525E-15));
#46318=DIRECTION('center_axis',(6.30774408230792E-14,-1.,8.61946552381526E-15));
#46319=DIRECTION('ref_axis',(-7.30945543516121E-15,-8.61946552381573E-15,
-1.));
#46320=DIRECTION('center_axis',(6.76186946307289E-14,-1.,8.61946552381525E-15));
#46321=DIRECTION('ref_axis',(2.76820162751153E-15,8.61946552381544E-15,
1.));
#46322=DIRECTION('center_axis',(6.82810966368524E-14,-1.,1.06870343811432E-14));
#46323=DIRECTION('ref_axis',(0.581108581114924,4.83761180111596E-14,0.813826036051071));
#46324=DIRECTION('center_axis',(-6.76186946307289E-14,1.,-8.61946552381525E-15));
#46325=DIRECTION('ref_axis',(-2.76820162751153E-15,-8.61946552381544E-15,
-1.));
#46326=DIRECTION('center_axis',(-6.69562926246054E-14,1.,-1.06870343811432E-14));
#46327=DIRECTION('ref_axis',(-0.581108581114914,-3.0211489376252E-14,0.813826036051079));
#46328=DIRECTION('center_axis',(6.76186946307289E-14,-1.,8.61946552381525E-15));
#46329=DIRECTION('ref_axis',(2.76820162751153E-15,8.61946552381544E-15,
1.));
#46330=DIRECTION('',(6.76186946307289E-14,-1.,8.61946552381525E-15));
#46331=DIRECTION('center_axis',(-6.13660760090327E-14,1.,9.49534209067263E-15));
#46332=DIRECTION('ref_axis',(0.581108581114914,2.79327967435979E-14,0.813826036051078));
#46333=DIRECTION('center_axis',(-6.76186946307289E-14,1.,-8.61946552381525E-15));
#46334=DIRECTION('ref_axis',(7.34396516680413E-14,8.61946552382022E-15,
1.));
#46335=DIRECTION('center_axis',(-6.76186946307289E-14,1.,-8.61946552381525E-15));
#46336=DIRECTION('ref_axis',(7.34396516680413E-14,8.61946552382022E-15,
1.));
#46337=DIRECTION('',(0.410905818312066,-0.707106781186573,0.575461908797841));
#46338=DIRECTION('center_axis',(6.25513333585901E-14,-1.,7.93981538629056E-15));
#46339=DIRECTION('ref_axis',(0.581108581114919,4.28107450576588E-14,0.813826036051075));
#46340=DIRECTION('center_axis',(6.76186946307289E-14,-1.,8.61946552381525E-15));
#46341=DIRECTION('ref_axis',(2.76820162751153E-15,8.61946552381544E-15,
1.));
#46342=DIRECTION('center_axis',(-6.82145042037028E-14,1.,-8.5945800386633E-15));
#46343=DIRECTION('ref_axis',(0.581108581114921,4.66345267536606E-14,0.813826036051073));
#46344=DIRECTION('',(-0.503254793602685,0.499999999999963,-0.704794021481423));
#46345=DIRECTION('center_axis',(6.76186946307289E-14,-1.,8.61946552381525E-15));
#46346=DIRECTION('ref_axis',(3.45767918888255E-15,8.61946552381548E-15,
1.));
#46347=DIRECTION('center_axis',(6.76186946307289E-14,-1.,8.61946552381525E-15));
#46348=DIRECTION('ref_axis',(3.45767918888255E-15,8.61946552381548E-15,
1.));
#46349=DIRECTION('center_axis',(-6.76186946307289E-14,1.,-8.61946552381525E-15));
#46350=DIRECTION('ref_axis',(-2.76820162751153E-15,-8.61946552381544E-15,
-1.));
#46351=DIRECTION('',(-6.76186946307289E-14,1.,-8.61946552381525E-15));
#46352=DIRECTION('center_axis',(-6.76186946307289E-14,1.,-8.61946552381525E-15));
#46353=DIRECTION('ref_axis',(-2.76820162751153E-15,-8.61946552381544E-15,
-1.));
#46354=DIRECTION('center_axis',(7.67012022460283E-14,-1.,8.61946552381523E-15));
#46355=DIRECTION('ref_axis',(-3.19394417197869E-15,-8.61946552381547E-15,
-1.));
#46356=DIRECTION('',(6.76186946307289E-14,-1.,8.61946552381525E-15));
#46357=DIRECTION('center_axis',(6.30774408230794E-14,-1.,8.61946552381514E-15));
#46358=DIRECTION('ref_axis',(5.55585269644891E-14,-8.61946552381163E-15,
-1.));
#46359=DIRECTION('center_axis',(6.76186946307289E-14,-1.,8.61946552381525E-15));
#46360=DIRECTION('ref_axis',(2.76820162751153E-15,8.61946552381544E-15,
1.));
#46361=DIRECTION('center_axis',(6.82810966368524E-14,-1.,1.06870343811432E-14));
#46362=DIRECTION('ref_axis',(0.581108581114918,4.83761180111593E-14,0.813826036051075));
#46363=DIRECTION('center_axis',(-6.76186946307289E-14,1.,-8.61946552381525E-15));
#46364=DIRECTION('ref_axis',(-2.76820162751153E-15,-8.61946552381544E-15,
-1.));
#46365=DIRECTION('center_axis',(-6.69562926246054E-14,1.,-1.06870343811432E-14));
#46366=DIRECTION('ref_axis',(-0.58110858111492,-3.02114893762525E-14,0.813826036051075));
#46367=DIRECTION('center_axis',(6.76186946307289E-14,-1.,8.61946552381525E-15));
#46368=DIRECTION('ref_axis',(4.22518722413247E-15,8.61946552381554E-15,
1.));
#46369=DIRECTION('',(6.76186946307289E-14,-1.,8.61946552381525E-15));
#46370=DIRECTION('center_axis',(-1.04261204031615E-14,-3.33541910048363E-16,
1.));
#46371=DIRECTION('ref_axis',(-0.581108581114994,0.813826036051022,-5.7872629435037E-15));
#46372=DIRECTION('center_axis',(2.76820162751153E-15,8.61946552381544E-15,
1.));
#46373=DIRECTION('ref_axis',(0.581108581114867,0.813826036051112,-8.62337118012903E-15));
#46374=DIRECTION('',(-0.410905818312093,0.575461908797838,-0.70710678118656));
#46375=DIRECTION('center_axis',(-3.80148262708044E-15,-5.39426451924816E-15,
-1.));
#46376=DIRECTION('ref_axis',(-0.581108581114975,0.813826036051035,-2.18091873555453E-15));
#46377=DIRECTION('center_axis',(2.76820162751153E-15,8.61946552381544E-15,
1.));
#46378=DIRECTION('ref_axis',(0.581108581114867,0.813826036051112,-8.62337118012903E-15));
#46379=DIRECTION('center_axis',(-2.76820162751153E-15,-8.61946552381544E-15,
-1.));
#46380=DIRECTION('ref_axis',(6.76186946307289E-14,-1.,8.61946552381525E-15));
#46381=DIRECTION('center_axis',(2.76820162751153E-15,8.61946552381544E-15,
1.));
#46382=DIRECTION('ref_axis',(-6.76186946307289E-14,1.,-8.61946552381525E-15));
#46383=DIRECTION('center_axis',(4.6446765469921E-16,-8.61946552381522E-15,
-1.));
#46384=DIRECTION('ref_axis',(-6.11533560663074E-14,1.,-8.61946552381525E-15));
#46385=DIRECTION('center_axis',(4.6446765469921E-16,-8.61946552381522E-15,
-1.));
#46386=DIRECTION('ref_axis',(-6.11533560663074E-14,1.,-8.61946552381525E-15));
#46387=DIRECTION('',(2.76820162751153E-15,8.61946552381544E-15,1.));
#46388=DIRECTION('center_axis',(-3.46259038420886E-16,8.70807119655905E-15,
1.));
#46389=DIRECTION('ref_axis',(0.581108581114959,-0.813826036051046,7.28806916206094E-15));
#46390=DIRECTION('',(-0.503254793602683,0.704794021481399,0.499999999999998));
#46391=DIRECTION('center_axis',(2.76820162751153E-15,8.61946552381544E-15,
1.));
#46392=DIRECTION('ref_axis',(6.76186946307289E-14,-1.,8.61946552381525E-15));
#46393=DIRECTION('center_axis',(-1.33644605120271E-14,-8.61946552381615E-15,
-1.));
#46394=DIRECTION('ref_axis',(4.11280474194391E-14,-1.,8.6194655238156E-15));
#46395=DIRECTION('',(-2.76820162751153E-15,-8.61946552381544E-15,-1.));
#46396=DIRECTION('center_axis',(-2.76820162751153E-15,-8.61946552381544E-15,
-1.));
#46397=DIRECTION('ref_axis',(0.58110858111497,-0.813826036051039,5.40611974012193E-15));
#46398=DIRECTION('center_axis',(-2.76820162751153E-15,-8.61946552381544E-15,
-1.));
#46399=DIRECTION('ref_axis',(6.76186946307289E-14,-1.,8.61946552381525E-15));
#46400=DIRECTION('center_axis',(-2.76820162751153E-15,-8.61946552381544E-15,
-1.));
#46401=DIRECTION('ref_axis',(-0.581108581114972,0.813826036051037,-5.40611974012191E-15));
#46402=DIRECTION('center_axis',(2.76820162751153E-15,8.61946552381544E-15,
1.));
#46403=DIRECTION('ref_axis',(-6.76186946307289E-14,1.,-8.61946552381525E-15));
#46404=DIRECTION('center_axis',(1.07977124127116E-14,7.41326354248036E-15,
1.));
#46405=DIRECTION('ref_axis',(0.581108581114866,0.813826036051113,-1.23077502224163E-14));
#46406=DIRECTION('',(2.76820162751153E-15,8.61946552381544E-15,1.));
#46407=DIRECTION('center_axis',(2.76820162751153E-15,8.61946552381544E-15,
1.));
#46408=DIRECTION('ref_axis',(-6.76186946307289E-14,1.,-8.61946552381525E-15));
#46409=DIRECTION('center_axis',(-6.76186946307289E-14,1.,-8.61946552381525E-15));
#46410=DIRECTION('ref_axis',(-1.91671653857721E-15,-8.61946552381538E-15,
-1.));
#46411=DIRECTION('center_axis',(7.67012022460283E-14,-1.,8.61946552381523E-15));
#46412=DIRECTION('ref_axis',(-3.33585835346774E-15,-8.61946552381548E-15,
-1.));
#46413=DIRECTION('',(6.76186946307289E-14,-1.,8.61946552381525E-15));
#46414=DIRECTION('center_axis',(6.30774408230794E-14,-1.,8.61946552381514E-15));
#46415=DIRECTION('ref_axis',(5.57004411459782E-14,-8.61946552381162E-15,
-1.));
#46416=DIRECTION('center_axis',(6.76186946307289E-14,-1.,8.61946552381525E-15));
#46417=DIRECTION('ref_axis',(2.76820162751153E-15,8.61946552381544E-15,
1.));
#46418=DIRECTION('center_axis',(6.82810966368524E-14,-1.,1.06870343811432E-14));
#46419=DIRECTION('ref_axis',(0.581108581114921,4.83761180111595E-14,0.813826036051073));
#46420=DIRECTION('center_axis',(6.76186946307289E-14,-1.,8.61946552381525E-15));
#46421=DIRECTION('ref_axis',(3.56292104385022E-15,8.61946552381549E-15,
1.));
#46422=DIRECTION('',(6.76186946307289E-14,-1.,8.61946552381525E-15));
#46423=DIRECTION('center_axis',(-6.69562926246054E-14,1.,-1.06870343811432E-14));
#46424=DIRECTION('ref_axis',(-0.581108581114923,-3.02114893762527E-14,0.813826036051072));
#46425=DIRECTION('center_axis',(-6.76186946307289E-14,1.,-8.61946552381525E-15));
#46426=DIRECTION('ref_axis',(-2.76820162751153E-15,-8.61946552381544E-15,
-1.));
#46427=DIRECTION('center_axis',(-6.72644410420969E-14,1.,-1.18043088936533E-14));
#46428=DIRECTION('ref_axis',(0.581108581114921,4.86945978087055E-14,0.813826036051073));
#46429=DIRECTION('center_axis',(-6.76186946307289E-14,1.,-8.61946552381525E-15));
#46430=DIRECTION('ref_axis',(7.32672822776985E-14,8.6194655238202E-15,1.));
#46431=DIRECTION('center_axis',(-6.76186946307289E-14,1.,-8.61946552381525E-15));
#46432=DIRECTION('ref_axis',(7.32672822776985E-14,8.6194655238202E-15,1.));
#46433=DIRECTION('',(0.410905818312108,-0.707106781186502,0.575461908797899));
#46434=DIRECTION('center_axis',(6.25513333585901E-14,-1.,7.93981538629056E-15));
#46435=DIRECTION('ref_axis',(0.581108581114918,4.28107450576588E-14,0.813826036051075));
#46436=DIRECTION('center_axis',(6.76186946307289E-14,-1.,8.61946552381525E-15));
#46437=DIRECTION('ref_axis',(2.76820162751153E-15,8.61946552381544E-15,
1.));
#46438=DIRECTION('center_axis',(-6.76186946307289E-14,1.,-8.61946552381525E-15));
#46439=DIRECTION('ref_axis',(-1.733985285455E-15,-8.61946552381537E-15,
-1.));
#46440=DIRECTION('center_axis',(6.76186946307289E-14,-1.,8.61946552381525E-15));
#46441=DIRECTION('ref_axis',(-3.63004857922531E-15,-8.6194655238155E-15,
-1.));
#46442=DIRECTION('center_axis',(6.76186946307289E-14,-1.,8.61946552381525E-15));
#46443=DIRECTION('ref_axis',(-3.63004857922531E-15,-8.6194655238155E-15,
-1.));
#46444=DIRECTION('',(-6.76186946307289E-14,1.,-8.61946552381525E-15));
#46445=DIRECTION('center_axis',(-6.81874306457619E-14,1.,-9.83494824371944E-15));
#46446=DIRECTION('ref_axis',(0.581108581114921,4.76282380163844E-14,0.813826036051073));
#46447=DIRECTION('',(-0.503254793602685,0.499999999999962,-0.704794021481423));
#46448=DIRECTION('center_axis',(-6.76186946307289E-14,1.,-8.61946552381525E-15));
#46449=DIRECTION('ref_axis',(-2.76820162751153E-15,-8.61946552381544E-15,
-1.));
#46450=DIRECTION('center_axis',(7.67012022460283E-14,-1.,8.61946552381523E-15));
#46451=DIRECTION('ref_axis',(-7.30945543516121E-15,-8.61946552381579E-15,
-1.));
#46452=DIRECTION('',(6.76186946307289E-14,-1.,8.61946552381525E-15));
#46453=DIRECTION('center_axis',(6.30774408230792E-14,-1.,8.61946552381526E-15));
#46454=DIRECTION('ref_axis',(-7.30945543516121E-15,-8.61946552381573E-15,
-1.));
#46455=DIRECTION('center_axis',(6.76186946307289E-14,-1.,8.61946552381525E-15));
#46456=DIRECTION('ref_axis',(2.76820162751153E-15,8.61946552381544E-15,
1.));
#46457=DIRECTION('center_axis',(6.82810966368524E-14,-1.,1.06870343811432E-14));
#46458=DIRECTION('ref_axis',(0.58110858111492,4.83761180111593E-14,0.813826036051075));
#46459=DIRECTION('center_axis',(6.76186946307289E-14,-1.,8.61946552381525E-15));
#46460=DIRECTION('ref_axis',(2.76820162751153E-15,8.61946552381544E-15,
1.));
#46461=DIRECTION('',(6.76186946307289E-14,-1.,8.61946552381525E-15));
#46462=DIRECTION('center_axis',(-6.69562926246054E-14,1.,-1.06870343811432E-14));
#46463=DIRECTION('ref_axis',(-0.581108581114923,-3.02114893762527E-14,0.813826036051073));
#46464=DIRECTION('center_axis',(-6.76186946307289E-14,1.,-8.61946552381525E-15));
#46465=DIRECTION('ref_axis',(-2.76820162751153E-15,-8.61946552381544E-15,
-1.));
#46466=DIRECTION('center_axis',(-6.50143608507664E-14,1.,-1.90373382615731E-14));
#46467=DIRECTION('ref_axis',(0.581108581114934,5.32734845204624E-14,0.813826036051064));
#46468=DIRECTION('center_axis',(-7.0376604876213E-14,1.,-8.61946552381524E-15));
#46469=DIRECTION('ref_axis',(-2.74761886345663E-15,8.61946552381505E-15,
1.));
#46470=DIRECTION('center_axis',(-7.0376604876213E-14,1.,-8.61946552381524E-15));
#46471=DIRECTION('ref_axis',(-2.74761886345663E-15,8.61946552381505E-15,
1.));
#46472=DIRECTION('',(0.410905818312139,-0.707106781186458,0.575461908797931));
#46473=DIRECTION('center_axis',(6.76186946307289E-14,-1.,8.61946552381525E-15));
#46474=DIRECTION('ref_axis',(0.58110858111492,4.63085491538314E-14,0.813826036051074));
#46475=DIRECTION('center_axis',(6.76186946307289E-14,-1.,8.61946552381525E-15));
#46476=DIRECTION('ref_axis',(2.76820162751153E-15,8.61946552381544E-15,
1.));
#46477=DIRECTION('center_axis',(-6.76186946307289E-14,1.,-8.61946552381525E-15));
#46478=DIRECTION('ref_axis',(-2.76820162751153E-15,-8.61946552381544E-15,
-1.));
#46479=DIRECTION('center_axis',(6.76186946307289E-14,-1.,8.61946552381525E-15));
#46480=DIRECTION('ref_axis',(-1.37998426094479E-14,-8.61946552381618E-15,
-1.));
#46481=DIRECTION('center_axis',(6.76186946307289E-14,-1.,8.61946552381525E-15));
#46482=DIRECTION('ref_axis',(-1.37998426094479E-14,-8.61946552381618E-15,
-1.));
#46483=DIRECTION('',(-6.76186946307289E-14,1.,-8.61946552381525E-15));
#46484=DIRECTION('center_axis',(-6.63187474944986E-14,1.,-8.81955372150551E-15));
#46485=DIRECTION('ref_axis',(0.581108581114964,4.57159757027617E-14,0.813826036051043));
#46486=DIRECTION('',(-0.503254793602721,0.499999999999963,-0.704794021481396));
#46487=DIRECTION('center_axis',(-6.76186946307289E-14,1.,-8.61946552381525E-15));
#46488=DIRECTION('ref_axis',(-2.76820162751153E-15,-8.61946552381544E-15,
-1.));
#46489=DIRECTION('',(-2.76820162751153E-15,-8.61946552381544E-15,-1.));
#46490=DIRECTION('',(1.,6.76186946307289E-14,-2.76820162751211E-15));
#46491=DIRECTION('',(-2.76820162751153E-15,-8.61946552381544E-15,-1.));
#46492=DIRECTION('',(1.,6.76186946307289E-14,-2.76820162751211E-15));
#46493=DIRECTION('',(-1.,-6.76186946307289E-14,2.76820162751211E-15));
#46494=DIRECTION('',(-0.70710678118655,-5.39085200304644E-14,-0.707106781186545));
#46495=DIRECTION('',(-2.76820162751153E-15,-8.61946552381544E-15,-1.));
#46496=DIRECTION('',(0.707106781186546,4.17187549862773E-14,-0.707106781186549));
#46497=DIRECTION('',(1.,6.76186946307289E-14,-2.76820162751211E-15));
#46498=DIRECTION('',(0.707106781186549,5.39085200304643E-14,0.707106781186546));
#46499=DIRECTION('',(2.76820162751153E-15,8.61946552381544E-15,1.));
#46500=DIRECTION('',(-0.707106781186542,-4.1718754986277E-14,0.707106781186553));
#46501=DIRECTION('',(0.532208296737218,4.32845857166654E-14,0.846613447143423));
#46502=DIRECTION('',(1.,6.76186946307289E-14,-2.76820162751211E-15));
#46503=DIRECTION('center_axis',(-6.17447804712825E-15,0.0512482385726126,
-0.998685945652188));
#46504=DIRECTION('ref_axis',(-0.111182235210154,0.992494128249466,0.0509305013131333));
#46505=DIRECTION('center_axis',(2.76820162751153E-15,8.61946552381544E-15,
1.));
#46506=DIRECTION('ref_axis',(-0.139174864659284,0.990267820868208,-8.15031525445884E-15));
#46507=DIRECTION('',(0.0050617559519412,-0.0872986470839505,0.996169325388006));
#46508=DIRECTION('center_axis',(-2.76820162751153E-15,-8.61946552381544E-15,
-1.));
#46509=DIRECTION('ref_axis',(0.139174864659155,0.990267820868226,-8.92084342817569E-15));
#46510=DIRECTION('',(0.00506175595192408,0.0872986470839512,-0.996169325388006));
#46511=DIRECTION('center_axis',(0.138643505293337,0.986499799769915,0.087155742747649));
#46512=DIRECTION('ref_axis',(-8.7256367158859E-15,0.0880056703438852,-0.996119973691585));
#46513=DIRECTION('',(0.99026806874158,-0.139173100959999,-1.54166393399594E-15));
#46514=DIRECTION('',(0.0121297349846599,0.0863075490504521,-0.996194698091746));
#46515=DIRECTION('',(-0.99026806874158,0.139173100959999,1.54166393399594E-15));
#46516=DIRECTION('center_axis',(-1.0957857610087E-16,-0.0512482385723115,
-0.998685945652203));
#46517=DIRECTION('ref_axis',(0.111182235210143,-0.992494128249482,0.0509305013128334));
#46518=DIRECTION('center_axis',(2.76820162751153E-15,8.61946552381544E-15,
1.));
#46519=DIRECTION('ref_axis',(0.139174864659253,-0.990267820868213,8.15031525445896E-15));
#46520=DIRECTION('',(-0.00506175595193837,0.0872986470839675,0.996169325388004));
#46521=DIRECTION('center_axis',(-2.76820162751272E-15,6.38329582726006E-15,
-1.));
#46522=DIRECTION('ref_axis',(-0.13917486465911,-0.990267820868233,-5.93590836195989E-15));
#46523=DIRECTION('',(-0.00506175595193187,-0.0872986470839681,-0.996169325388004));
#46524=DIRECTION('center_axis',(-0.138643505293338,-0.986499799769913,0.0871557427476672));
#46525=DIRECTION('ref_axis',(-3.15693842339108E-15,0.0880056703439027,0.996119973691583));
#46526=DIRECTION('',(-0.99026806874158,0.139173100959998,1.54166393399595E-15));
#46527=DIRECTION('',(-0.698023464708466,0.159770101811378,0.698023464708437));
#46528=DIRECTION('',(-0.532208296737254,-4.32845857166677E-14,-0.8466134471434));
#46529=DIRECTION('',(-0.012129734984676,-0.0863075490504701,-0.996194698091745));
#46530=DIRECTION('',(0.99026806874158,-0.139173100959997,-1.54166393399596E-15));
#46531=DIRECTION('center_axis',(-0.13864350529347,0.986499799769896,0.0871557427476489));
#46532=DIRECTION('ref_axis',(-8.76900480278526E-15,0.0880056703438843,-0.996119973691585));
#46533=DIRECTION('',(-0.990268068741561,-0.139173100960131,3.94085942513142E-15));
#46534=DIRECTION('',(-0.0121297349846877,0.0863075490504512,-0.996194698091746));
#46535=DIRECTION('',(0.698023464708433,0.159770101811467,-0.698023464708449));
#46536=DIRECTION('',(0.99026806874156,0.139173100960136,-3.94085942513146E-15));
#46537=DIRECTION('center_axis',(-2.76820162751153E-15,-8.61946552381544E-15,
-1.));
#46538=DIRECTION('ref_axis',(6.76186946307289E-14,-1.,8.61946552381525E-15));
#46539=DIRECTION('',(-6.76186946307289E-14,1.,-8.61946552381525E-15));
#46540=DIRECTION('',(1.,6.76186946307289E-14,-2.76820162751211E-15));
#46541=DIRECTION('',(-6.76186946307289E-14,1.,-8.61946552381525E-15));
#46542=DIRECTION('center_axis',(3.60302193317522E-14,1.60759898378342E-13,
-1.));
#46543=DIRECTION('ref_axis',(0.305752646092157,0.952110980614993,1.64077599388534E-13));
#46544=DIRECTION('center_axis',(-2.76820162751153E-15,-8.61946552381544E-15,
-1.));
#46545=DIRECTION('ref_axis',(6.76186946307289E-14,-1.,8.61946552381525E-15));
#46546=DIRECTION('',(-0.990268068741561,-0.139173100960133,3.94085942513144E-15));
#46547=DIRECTION('center_axis',(-4.15666225867972E-14,1.6075989837832E-13,
-1.));
#46548=DIRECTION('ref_axis',(0.139173100960163,-0.990268068741557,-1.64980349860033E-13));
#46549=DIRECTION('',(1.,6.76186946307289E-14,-2.76820162751211E-15));
#46550=DIRECTION('',(-6.76186946307289E-14,1.,-8.61946552381525E-15));
#46551=DIRECTION('',(1.,6.76186946307289E-14,-2.76820162751211E-15));
#46552=DIRECTION('',(-6.76186946307289E-14,1.,-8.61946552381525E-15));
#46553=DIRECTION('center_axis',(0.138643505293472,-0.986499799769894,0.0871557427476665));
#46554=DIRECTION('ref_axis',(-3.24020515023797E-15,0.0880056703439028,0.996119973691583));
#46555=DIRECTION('',(0.990268068741561,0.139173100960135,-3.94085942513146E-15));
#46556=DIRECTION('',(0.0121297349846716,-0.08630754905047,-0.996194698091745));
#46557=DIRECTION('center_axis',(-2.76820162751153E-15,-8.61946552381544E-15,
-1.));
#46558=DIRECTION('ref_axis',(6.76186946307289E-14,-1.,8.61946552381525E-15));
#46559=DIRECTION('center_axis',(1.261874465981E-15,8.2847073667892E-15,
1.));
#46560=DIRECTION('ref_axis',(0.139173100959999,0.99026806874158,-8.3797001466523E-15));
#46561=DIRECTION('',(-1.,-6.76186946307289E-14,2.76820162751211E-15));
#46562=DIRECTION('',(-6.76186946307289E-14,1.,-8.61946552381525E-15));
#46563=DIRECTION('',(1.,6.76186946307289E-14,-2.76820162751211E-15));
#46564=DIRECTION('center_axis',(-2.44452695549615E-16,9.28898183786753E-15,
1.));
#46565=DIRECTION('ref_axis',(0.545502031847834,0.838109499558312,-7.6518344774284E-15));
#46566=DIRECTION('center_axis',(2.76820162751153E-15,8.61946552381544E-15,
1.));
#46567=DIRECTION('ref_axis',(-0.139173100960041,-0.990268068741574,8.9208406824367E-15));
#46568=DIRECTION('',(1.,6.76186946307289E-14,-2.76820162751211E-15));
#46569=DIRECTION('',(6.76186946307289E-14,-1.,8.61946552381525E-15));
#46570=DIRECTION('',(-1.,-6.76186946307289E-14,2.76820162751211E-15));
#46571=DIRECTION('center_axis',(2.76820162751153E-15,8.61946552381544E-15,
1.));
#46572=DIRECTION('ref_axis',(-0.54550203184785,-0.838109499558302,8.73411554899706E-15));
#46573=DIRECTION('center_axis',(-2.86014741974442E-15,-8.33247325201429E-15,
-1.));
#46574=DIRECTION('ref_axis',(-0.581108581114976,0.813826036051034,-5.11912746832073E-15));
#46575=DIRECTION('center_axis',(-1.,-6.76186946307289E-14,2.76820162751211E-15));
#46576=DIRECTION('ref_axis',(6.76186946307289E-14,-1.,8.61946552381525E-15));
#46577=DIRECTION('center_axis',(-1.,-6.76186946307289E-14,2.76820162751211E-15));
#46578=DIRECTION('ref_axis',(5.34212284942708E-14,-0.813826036051078,-0.581108581114915));
#46579=DIRECTION('',(-1.,-6.76186946307289E-14,2.76820162751211E-15));
#46580=DIRECTION('center_axis',(1.,6.76186946307289E-14,-2.53239663548226E-15));
#46581=DIRECTION('ref_axis',(6.76186946307289E-14,-1.,4.84658565133759E-15));
#46582=DIRECTION('center_axis',(1.,6.76186946307289E-14,-2.53239663548226E-15));
#46583=DIRECTION('ref_axis',(6.76186946307289E-14,-1.,4.84658565133759E-15));
#46584=DIRECTION('center_axis',(-5.05637727264981E-14,0.719339800338649,
-0.694658370458999));
#46585=DIRECTION('ref_axis',(4.49806146187151E-14,-0.694658370458999,-0.719339800338649));
#46586=DIRECTION('center_axis',(-3.56199649102086E-14,0.719339800338649,
-0.694658370458999));
#46587=DIRECTION('ref_axis',(-4.85907466234332E-15,0.694658370458999,0.719339800338649));
#46588=DIRECTION('',(-4.49806146187153E-14,0.694658370459002,0.719339800338646));
#46589=DIRECTION('center_axis',(1.,6.76186946307289E-14,-2.76820162751211E-15));
#46590=DIRECTION('ref_axis',(-6.76186946307289E-14,1.,-8.61946552381525E-15));
#46591=DIRECTION('',(4.8963169830778E-14,-0.694658370458992,0.719339800338656));
#46592=DIRECTION('',(-6.76741119925271E-14,0.999390827019096,-0.0348994967025082));
#46593=DIRECTION('',(-6.74808943053847E-14,0.999390827019096,0.0348994967024911));
#46594=DIRECTION('',(4.49806146187149E-14,-0.694658370458996,-0.719339800338652));
#46595=DIRECTION('',(2.76820162751153E-15,8.61946552381544E-15,1.));
#46596=DIRECTION('',(4.89631698307778E-14,-0.694658370458988,0.71933980033866));
#46597=DIRECTION('center_axis',(-1.,-6.76186946307289E-14,2.76820162751211E-15));
#46598=DIRECTION('ref_axis',(5.34212284942709E-14,-0.813826036051079,-0.581108581114913));
#46599=DIRECTION('center_axis',(-1.,-6.76186946307289E-14,2.76820162751211E-15));
#46600=DIRECTION('ref_axis',(5.34212284942708E-14,-0.813826036051078,-0.581108581114915));
#46601=DIRECTION('center_axis',(-1.,-6.71637446241253E-14,6.1602351414295E-15));
#46602=DIRECTION('ref_axis',(5.10798385514284E-14,-0.813826036051077,-0.581108581114916));
#46603=DIRECTION('center_axis',(-1.,-6.76186946307289E-14,2.76820162751211E-15));
#46604=DIRECTION('ref_axis',(6.76186946307289E-14,-1.,8.61946552381525E-15));
#46605=DIRECTION('',(-1.,-6.76186946307289E-14,2.76820162751211E-15));
#46606=DIRECTION('center_axis',(1.,6.76186946307289E-14,-2.53239663548226E-15));
#46607=DIRECTION('ref_axis',(6.76186946307289E-14,-1.,6.73302558757642E-15));
#46608=DIRECTION('center_axis',(1.,6.76186946307289E-14,-2.53239663548226E-15));
#46609=DIRECTION('ref_axis',(6.76186946307289E-14,-1.,6.73302558757642E-15));
#46610=DIRECTION('center_axis',(4.67178638631601E-14,-0.719339800338664,
-0.694658370458984));
#46611=DIRECTION('ref_axis',(4.89631698307775E-14,-0.694658370458984,0.719339800338664));
#46612=DIRECTION('',(1.,6.76186946307289E-14,-2.76820162751211E-15));
#46613=DIRECTION('center_axis',(6.48738920511758E-14,-0.719339800338663,
-0.694658370458985));
#46614=DIRECTION('ref_axis',(7.79045361699332E-14,-0.694658370458985,0.719339800338663));
#46615=DIRECTION('center_axis',(5.12637372416684E-15,-0.0348994967024915,
0.999390827019096));
#46616=DIRECTION('ref_axis',(-6.74808943053847E-14,0.999390827019096,0.0348994967024915));
#46617=DIRECTION('',(1.,6.76186946307289E-14,-2.76820162751211E-15));
#46618=DIRECTION('',(1.,6.76186946307289E-14,-2.76820162751211E-15));
#46619=DIRECTION('center_axis',(-7.21499697121947E-15,-0.0348994967024795,
0.999390827019097));
#46620=DIRECTION('ref_axis',(2.54229873860636E-12,0.999390827019096,0.0348994967024795));
#46621=DIRECTION('',(1.,6.76186946307289E-14,-2.76820162751211E-15));
#46622=DIRECTION('center_axis',(3.92980782396055E-15,-0.0348994967025042,
0.999390827019096));
#46623=DIRECTION('ref_axis',(1.41395947801337E-12,0.999390827019096,0.0348994967025042));
#46624=DIRECTION('',(1.,6.76186946307289E-14,-2.76820162751211E-15));
#46625=DIRECTION('',(0.0174417781380274,0.999238800303652,0.0348941878126054));
#46626=DIRECTION('',(0.713036894919998,0.70069940513849,0.0244689624098382));
#46627=DIRECTION('',(1.,6.76186946307289E-14,-2.76820162751211E-15));
#46628=DIRECTION('',(-6.74808943053847E-14,0.999390827019096,0.0348994967024838));
#46629=DIRECTION('center_axis',(-1.,-6.76186946307289E-14,2.76820162751211E-15));
#46630=DIRECTION('ref_axis',(6.76186946307289E-14,-1.,8.61946552381525E-15));
#46631=DIRECTION('',(-1.,-6.76186946307289E-14,2.76820162751211E-15));
#46632=DIRECTION('center_axis',(1.,6.76186946307289E-14,-2.53239663548226E-15));
#46633=DIRECTION('ref_axis',(6.76186946307289E-14,-1.,1.05059054600541E-14));
#46634=DIRECTION('center_axis',(1.,6.76186946307289E-14,-2.53239663548226E-15));
#46635=DIRECTION('ref_axis',(6.76186946307289E-14,-1.,1.05059054600541E-14));
#46636=DIRECTION('center_axis',(5.03724005550908E-14,-0.719339800338648,
0.694658370459));
#46637=DIRECTION('ref_axis',(-4.49806146187152E-14,0.694658370459,0.719339800338648));
#46638=DIRECTION('',(-4.49806146187149E-14,0.694658370458996,0.719339800338652));
#46639=DIRECTION('',(1.,6.76186946307289E-14,-2.76820162751211E-15));
#46640=DIRECTION('center_axis',(-4.67178638631599E-14,0.71933980033866,
0.694658370458988));
#46641=DIRECTION('ref_axis',(-4.89631698307778E-14,0.694658370458988,-0.71933980033866));
#46642=DIRECTION('',(-4.8963169830778E-14,0.694658370458991,-0.719339800338657));
#46643=DIRECTION('',(1.,6.76186946307289E-14,-2.76820162751211E-15));
#46644=DIRECTION('center_axis',(-1.,-6.76186946307289E-14,2.76820162751211E-15));
#46645=DIRECTION('ref_axis',(6.76186946307289E-14,-1.,8.61946552381525E-15));
#46646=DIRECTION('',(-1.,-6.76186946307289E-14,2.76820162751211E-15));
#46647=DIRECTION('center_axis',(1.,6.76186946307289E-14,-2.53239663548226E-15));
#46648=DIRECTION('ref_axis',(6.76186946307289E-14,-1.,-2.69917409361775E-15));
#46649=DIRECTION('center_axis',(1.,6.76186946307289E-14,-2.53239663548226E-15));
#46650=DIRECTION('ref_axis',(6.76186946307289E-14,-1.,-2.69917409361775E-15));
#46651=DIRECTION('center_axis',(4.06656903581742E-16,0.0348994967025106,
0.999390827019095));
#46652=DIRECTION('ref_axis',(-6.76741119925271E-14,0.999390827019096,-0.0348994967025106));
#46653=DIRECTION('',(-6.7674111992527E-14,0.999390827019096,-0.0348994967025031));
#46654=DIRECTION('',(-1.,-6.76186946307289E-14,2.76820162751211E-15));
#46655=DIRECTION('',(-0.713036894920085,0.700699405138401,-0.0244689624098501));
#46656=DIRECTION('',(-0.0174417781381626,0.999238800303649,-0.0348941878126222));
#46657=DIRECTION('center_axis',(-9.8008354509373E-16,0.0348994967025452,
0.999390827019094));
#46658=DIRECTION('ref_axis',(-1.55020631512074E-12,-0.999390827019094,0.0348994967025452));
#46659=DIRECTION('center_axis',(3.48081291315565E-15,0.034899496702521,
0.999390827019095));
#46660=DIRECTION('ref_axis',(-4.33836829016131E-13,-0.999390827019095,0.034899496702521));
#46661=DIRECTION('center_axis',(6.76186946307289E-14,-1.,8.61946552381525E-15));
#46662=DIRECTION('ref_axis',(2.76820162751153E-15,8.61946552381544E-15,
1.));
#46663=DIRECTION('',(2.76820162751153E-15,8.61946552381544E-15,1.));
#46664=DIRECTION('center_axis',(6.42420170581153E-14,-1.,8.11391641182261E-15));
#46665=DIRECTION('ref_axis',(0.664254779227899,4.87382700579703E-14,0.747506246310287));
#46666=DIRECTION('',(2.76820162751153E-15,8.61946552381544E-15,1.));
#46667=DIRECTION('',(1.,6.76186946307289E-14,-2.76820162751211E-15));
#46668=DIRECTION('',(0.70710678118654,4.17187549862768E-14,-0.707106781186555));
#46669=DIRECTION('',(-2.76820162751153E-15,-8.61946552381544E-15,-1.));
#46670=DIRECTION('',(-0.707106781186549,-5.39085200304643E-14,-0.707106781186546));
#46671=DIRECTION('',(-1.,-6.76186946307289E-14,2.76820162751211E-15));
#46672=DIRECTION('',(-0.707106781186546,-4.17187549862773E-14,0.707106781186549));
#46673=DIRECTION('',(2.76820162751153E-15,8.61946552381544E-15,1.));
#46674=DIRECTION('',(0.707106781186549,5.39085200304643E-14,0.707106781186546));
#46675=DIRECTION('center_axis',(2.76820162751153E-15,8.61946552381544E-15,
1.));
#46676=DIRECTION('ref_axis',(-6.76186946307289E-14,1.,-8.61946552381525E-15));
#46677=DIRECTION('center_axis',(-5.20004799022464E-15,-4.34637833531572E-15,
-1.));
#46678=DIRECTION('ref_axis',(-6.57727994239961E-14,1.,-4.34637833531538E-15));
#46679=DIRECTION('',(2.76820162751153E-15,8.61946552381544E-15,1.));
#46680=DIRECTION('center_axis',(-2.15290322526726E-15,-8.6194655238154E-15,
-1.));
#46681=DIRECTION('ref_axis',(-6.82339930329732E-14,1.,-8.61946552381525E-15));
#46682=DIRECTION('center_axis',(-2.15290322526726E-15,-8.6194655238154E-15,
-1.));
#46683=DIRECTION('ref_axis',(-6.82339930329732E-14,1.,-8.61946552381525E-15));
#46684=DIRECTION('center_axis',(-5.20004799022464E-15,-4.34637833531572E-15,
-1.));
#46685=DIRECTION('ref_axis',(-6.57727994239961E-14,1.,-4.34637833531538E-15));
#46686=DIRECTION('',(-2.76820162751153E-15,-8.61946552381544E-15,-1.));
#46687=DIRECTION('center_axis',(5.12637372416674E-15,-0.0348994967024901,
0.999390827019096));
#46688=DIRECTION('ref_axis',(-6.74808943053847E-14,0.999390827019096,0.0348994967024901));
#46689=DIRECTION('center_axis',(4.06656903581789E-16,0.0348994967025099,
0.999390827019095));
#46690=DIRECTION('ref_axis',(-6.7674111992527E-14,0.999390827019095,-0.0348994967025099));
#46691=DIRECTION('',(2.76820162751153E-15,8.61946552381544E-15,1.));
#46692=DIRECTION('center_axis',(-2.76820162751153E-15,-8.61946552381544E-15,
-1.));
#46693=DIRECTION('ref_axis',(6.76186946307289E-14,-1.,8.61946552381525E-15));
#46694=DIRECTION('center_axis',(-3.27006405595157E-15,2.95336814164933E-15,
1.));
#46695=DIRECTION('ref_axis',(7.06970933615109E-14,-1.,2.95336814164956E-15));
#46696=DIRECTION('',(2.76820162751153E-15,8.61946552381544E-15,1.));
#46697=DIRECTION('center_axis',(-2.76820162751153E-15,-8.61946552381544E-15,
-1.));
#46698=DIRECTION('ref_axis',(-6.88500541230417E-14,1.,-8.61946552381525E-15));
#46699=DIRECTION('center_axis',(-3.27006405595157E-15,2.95336814164933E-15,
1.));
#46700=DIRECTION('ref_axis',(7.06970933615109E-14,-1.,2.95336814164956E-15));
#46701=DIRECTION('',(-2.76820162751153E-15,-8.61946552381544E-15,-1.));
#46702=DIRECTION('center_axis',(-4.06656903581438E-16,-0.0348994967025151,
-0.999390827019095));
#46703=DIRECTION('ref_axis',(6.7674111992527E-14,-0.999390827019095,0.0348994967025151));
#46704=DIRECTION('center_axis',(-5.12637372416635E-15,0.0348994967024843,
-0.999390827019096));
#46705=DIRECTION('ref_axis',(6.74808943053847E-14,-0.999390827019096,-0.0348994967024843));
#46706=DIRECTION('',(2.76820162751153E-15,8.61946552381544E-15,1.));
#46707=DIRECTION('center_axis',(-4.06656903581438E-16,-0.0348994967025151,
-0.999390827019095));
#46708=DIRECTION('ref_axis',(6.7674111992527E-14,-0.999390827019095,0.0348994967025151));
#46709=DIRECTION('',(-6.7674111992527E-14,0.999390827019096,-0.0348994967025004));
#46710=DIRECTION('',(-1.,-6.76186946307289E-14,2.76820162751211E-15));
#46711=DIRECTION('center_axis',(-5.12637372416635E-15,0.0348994967024843,
-0.999390827019096));
#46712=DIRECTION('ref_axis',(6.74808943053847E-14,-0.999390827019096,-0.0348994967024843));
#46713=DIRECTION('',(-6.74808943053847E-14,0.999390827019096,0.0348994967024933));
#46714=DIRECTION('center_axis',(0.500000000000092,4.12740234260384E-14,
0.866025403784385));
#46715=DIRECTION('ref_axis',(-6.76186946307289E-14,1.,-8.61946552381525E-15));
#46716=DIRECTION('',(0.866025403784435,5.42497745590457E-14,-0.500000000000006));
#46717=DIRECTION('',(6.76186946307289E-14,-1.,8.61946552381525E-15));
#46718=DIRECTION('',(0.866025403784435,5.42497745590457E-14,-0.500000000000006));
#46719=DIRECTION('',(6.76186946307289E-14,-1.,8.61946552381525E-15));
#46720=DIRECTION('center_axis',(1.,6.76186946307289E-14,-2.76820162751211E-15));
#46721=DIRECTION('ref_axis',(-6.76186946307289E-14,1.,-8.61946552381525E-15));
#46722=DIRECTION('',(-2.76820162751153E-15,-8.61946552381544E-15,-1.));
#46723=DIRECTION('',(6.76186946307289E-14,-1.,8.61946552381525E-15));
#46724=DIRECTION('',(-2.76820162751153E-15,-8.61946552381544E-15,-1.));
#46725=DIRECTION('center_axis',(0.500000000000088,2.63446712047027E-14,
-0.866025403784388));
#46726=DIRECTION('ref_axis',(6.76186946307289E-14,-1.,8.61946552381525E-15));
#46727=DIRECTION('',(-0.866025403784438,-6.28692400828612E-14,-0.500000000000002));
#46728=DIRECTION('',(6.76186946307289E-14,-1.,8.61946552381525E-15));
#46729=DIRECTION('',(-0.866025403784438,-6.28692400828612E-14,-0.500000000000002));
#46730=DIRECTION('center_axis',(2.76820162751153E-15,8.61946552381544E-15,
1.));
#46731=DIRECTION('ref_axis',(-6.76186946307289E-14,1.,-8.61946552381525E-15));
#46732=DIRECTION('',(-6.76186946307289E-14,1.,-8.61946552381525E-15));
#46733=DIRECTION('center_axis',(6.59733936268404E-14,-4.45999109629057E-16,
1.));
#46734=DIRECTION('ref_axis',(1.,5.89801867114909E-14,-6.59733936268404E-14));
#46735=DIRECTION('center_axis',(3.08914665434315E-15,8.61946552381546E-15,
1.));
#46736=DIRECTION('ref_axis',(-0.979681390452711,0.200560148585511,1.29765820345512E-15));
#46737=DIRECTION('center_axis',(-2.76820162751153E-15,-8.61946552381544E-15,
-1.));
#46738=DIRECTION('ref_axis',(6.76186946307289E-14,-1.,8.61946552381525E-15));
#46739=DIRECTION('',(6.76186946307289E-14,-1.,8.61946552381525E-15));
#46740=DIRECTION('center_axis',(3.58207973448846E-15,8.61946552381549E-15,
1.));
#46741=DIRECTION('ref_axis',(6.76186946307289E-14,-1.,8.61946552381525E-15));
#46742=DIRECTION('center_axis',(-1.,-6.76186946307289E-14,2.76820162751211E-15));
#46743=DIRECTION('ref_axis',(6.76186946307289E-14,-1.,8.61946552381525E-15));
#46744=DIRECTION('center_axis',(1.,6.76186946307288E-14,-6.54108149998981E-15));
#46745=DIRECTION('ref_axis',(6.7618694630729E-14,-1.,1.80516652050094E-14));
#46746=DIRECTION('center_axis',(1.,6.76186946307288E-14,-6.54108149998981E-15));
#46747=DIRECTION('ref_axis',(6.7618694630729E-14,-1.,1.80516652050094E-14));
#46748=DIRECTION('',(-1.,-6.76186946307289E-14,2.76820162751211E-15));
#46749=DIRECTION('center_axis',(1.,6.57782599518977E-14,-2.17856824283608E-15));
#46750=DIRECTION('ref_axis',(5.47980452554462E-14,-0.813826036051068,0.581108581114929));
#46751=DIRECTION('center_axis',(-1.,-6.76186946307289E-14,2.76820162751211E-15));
#46752=DIRECTION('ref_axis',(6.76186946307289E-14,-1.,8.61946552381525E-15));
#46753=DIRECTION('center_axis',(1.,6.76186946307288E-14,-6.54108149998976E-15));
#46754=DIRECTION('ref_axis',(6.76186946307289E-14,-1.,4.84658565133759E-15));
#46755=DIRECTION('center_axis',(1.,6.76186946307288E-14,-6.54108149998976E-15));
#46756=DIRECTION('ref_axis',(6.76186946307289E-14,-1.,4.84658565133759E-15));
#46757=DIRECTION('',(-1.,-6.76186946307289E-14,2.76820162751211E-15));
#46758=DIRECTION('center_axis',(1.,6.48270906338569E-14,-2.13515025569885E-14));
#46759=DIRECTION('ref_axis',(6.51655155548385E-14,-0.813826036051071,0.581108581114924));
#46760=DIRECTION('center_axis',(-1.,-6.76186946307289E-14,2.76820162751211E-15));
#46761=DIRECTION('ref_axis',(6.76186946307289E-14,-1.,8.61946552381525E-15));
#46762=DIRECTION('center_axis',(1.,6.76186946307288E-14,-6.54108149998976E-15));
#46763=DIRECTION('ref_axis',(6.76186946307289E-14,-1.,6.73302558757642E-15));
#46764=DIRECTION('center_axis',(1.,6.76186946307288E-14,-6.54108149998976E-15));
#46765=DIRECTION('ref_axis',(6.76186946307289E-14,-1.,6.73302558757642E-15));
#46766=DIRECTION('',(-1.,-6.76186946307289E-14,2.76820162751211E-15));
#46767=DIRECTION('center_axis',(1.,6.57576252994809E-14,-1.51570689138297E-14));
#46768=DIRECTION('ref_axis',(6.23231703479847E-14,-0.813826036051068,0.581108581114929));
#46769=DIRECTION('center_axis',(-1.,-6.76186946307289E-14,2.76820162751211E-15));
#46770=DIRECTION('ref_axis',(6.76186946307289E-14,-1.,8.61946552381525E-15));
#46771=DIRECTION('center_axis',(1.,6.76186946307288E-14,-6.54108149998981E-15));
#46772=DIRECTION('ref_axis',(6.7618694630729E-14,-1.,1.80516652050094E-14));
#46773=DIRECTION('center_axis',(1.,6.76186946307288E-14,-6.54108149998981E-15));
#46774=DIRECTION('ref_axis',(6.7618694630729E-14,-1.,1.80516652050094E-14));
#46775=DIRECTION('',(-1.,-6.76186946307289E-14,2.76820162751211E-15));
#46776=DIRECTION('center_axis',(1.,6.94384946571432E-14,-1.63363356831818E-14));
#46777=DIRECTION('ref_axis',(6.60040397056471E-14,-0.813826036051069,0.581108581114927));
#46778=DIRECTION('center_axis',(-1.,-6.76186946307289E-14,2.76820162751211E-15));
#46779=DIRECTION('ref_axis',(6.76186946307289E-14,-1.,8.61946552381525E-15));
#46780=DIRECTION('center_axis',(-4.06656903581789E-16,-0.0348994967025099,
-0.999390827019095));
#46781=DIRECTION('ref_axis',(6.7674111992527E-14,-0.999390827019096,0.0348994967025099));
#46782=DIRECTION('',(-1.,-6.76186946307289E-14,2.76820162751211E-15));
#46783=DIRECTION('',(-0.0174417781380384,-0.999238800303652,0.0348941878126222));
#46784=DIRECTION('',(-0.713036894919993,-0.700699405138495,0.0244689624098544));
#46785=DIRECTION('',(-1.,-6.76186946307289E-14,2.76820162751211E-15));
#46786=DIRECTION('',(-6.76741119925271E-14,0.999390827019096,-0.0348994967025096));
#46787=DIRECTION('center_axis',(-5.12637372416674E-15,0.0348994967024901,
-0.999390827019096));
#46788=DIRECTION('ref_axis',(6.74808943053847E-14,-0.999390827019096,-0.0348994967024901));
#46789=DIRECTION('',(-6.74808943053847E-14,0.999390827019096,0.0348994967024924));
#46790=DIRECTION('',(1.,6.76186946307289E-14,-2.76820162751211E-15));
#46791=DIRECTION('',(0.713036894920087,-0.700699405138399,-0.0244689624098423));
#46792=DIRECTION('',(0.0174417781381465,-0.99923880030365,-0.034894187812605));
#46793=DIRECTION('center_axis',(-6.76186946307289E-14,1.,-8.61946552381525E-15));
#46794=DIRECTION('ref_axis',(-2.76820162751153E-15,-8.61946552381544E-15,
-1.));
#46795=DIRECTION('',(2.76820162751153E-15,8.61946552381544E-15,1.));
#46796=DIRECTION('center_axis',(7.38750159181778E-14,-1.,1.0997592254033E-14));
#46797=DIRECTION('ref_axis',(0.664254779227879,4.08510634849217E-14,-0.747506246310305));
#46798=DIRECTION('center_axis',(7.38750159181778E-14,-1.,1.0997592254033E-14));
#46799=DIRECTION('ref_axis',(0.664254779227879,4.08510634849217E-14,-0.747506246310305));
#46800=DIRECTION('',(0.866025403784436,6.28692400828612E-14,0.500000000000004));
#46801=DIRECTION('',(2.76820162751153E-15,8.61946552381544E-15,1.));
#46802=DIRECTION('',(-0.866025403784434,-5.42497745590456E-14,0.500000000000009));
#46803=DIRECTION('center_axis',(-6.76186946307289E-14,1.,-8.61946552381525E-15));
#46804=DIRECTION('ref_axis',(-2.76820162751153E-15,-8.61946552381544E-15,
-1.));
#46805=DIRECTION('',(-2.76820162751153E-15,-8.61946552381544E-15,-1.));
#46806=DIRECTION('',(-1.,-6.76186946307289E-14,2.76820162751211E-15));
#46807=DIRECTION('center_axis',(-6.76186946307289E-14,1.,-8.61946552381525E-15));
#46808=DIRECTION('ref_axis',(0.973373605804438,6.77940443873129E-14,0.229224395567456));
#46809=DIRECTION('',(1.,6.76186946307289E-14,-2.76820162751211E-15));
#46810=DIRECTION('center_axis',(6.59789806251287E-14,-1.,8.3132822970341E-15));
#46811=DIRECTION('ref_axis',(-1.,-6.59789806251287E-14,2.7682016275121E-15));
#46812=DIRECTION('center_axis',(6.72378933645552E-14,-1.,1.14586580466301E-14));
#46813=DIRECTION('ref_axis',(-0.813826036051072,-4.80612237103423E-14,0.581108581114923));
#46814=DIRECTION('',(-6.59789806251287E-14,1.,-8.3132822970341E-15));
#46815=DIRECTION('center_axis',(-6.74261350511498E-14,1.,-8.55777381697828E-15));
#46816=DIRECTION('ref_axis',(-0.813826036051075,-5.98461400152083E-14,-0.58110858111492));
#46817=DIRECTION('center_axis',(6.76186946307289E-14,-1.,8.61946552381525E-15));
#46818=DIRECTION('ref_axis',(2.76820162751153E-15,8.61946552381544E-15,
1.));
#46819=DIRECTION('center_axis',(0.86602540378444,5.42497745590461E-14,-0.499999999999998));
#46820=DIRECTION('ref_axis',(-6.76186946307289E-14,1.,-8.61946552381525E-15));
#46821=DIRECTION('',(0.500000000000023,4.1274023426034E-14,0.866025403784425));
#46822=DIRECTION('',(6.76186946307289E-14,-1.,8.61946552381525E-15));
#46823=DIRECTION('',(0.500000000000005,4.12740234260329E-14,0.866025403784436));
#46824=DIRECTION('',(6.76186946307289E-14,-1.,8.61946552381525E-15));
#46825=DIRECTION('center_axis',(-2.76820162751153E-15,-8.61946552381544E-15,
-1.));
#46826=DIRECTION('ref_axis',(6.76186946307289E-14,-1.,8.61946552381525E-15));
#46827=DIRECTION('',(1.,6.76186946307289E-14,-2.76820162751211E-15));
#46828=DIRECTION('',(1.,6.76186946307289E-14,-2.76820162751211E-15));
#46829=DIRECTION('',(6.76186946307289E-14,-1.,8.61946552381525E-15));
#46830=DIRECTION('center_axis',(-0.86602540378444,-6.28692400828613E-14,
-0.499999999999998));
#46831=DIRECTION('ref_axis',(6.76186946307289E-14,-1.,8.61946552381525E-15));
#46832=DIRECTION('',(0.500000000000008,2.63446712046968E-14,-0.866025403784434));
#46833=DIRECTION('',(0.499999999999997,2.63446712046961E-14,-0.86602540378444));
#46834=DIRECTION('',(6.76186946307289E-14,-1.,8.61946552381525E-15));
#46835=DIRECTION('center_axis',(-0.866025403784437,-5.42497745590459E-14,
0.500000000000003));
#46836=DIRECTION('ref_axis',(-6.76186946307289E-14,1.,-8.61946552381525E-15));
#46837=DIRECTION('',(-0.500000000000012,-4.12740234260334E-14,-0.866025403784431));
#46838=DIRECTION('',(-0.500000000000003,-4.12740234260328E-14,-0.866025403784437));
#46839=DIRECTION('',(6.76186946307289E-14,-1.,8.61946552381525E-15));
#46840=DIRECTION('center_axis',(4.50475380710499E-14,-1.,4.08063979811324E-14));
#46841=DIRECTION('ref_axis',(-0.218698251317282,2.99667608013125E-14,0.975792536798044));
#46842=DIRECTION('center_axis',(8.99762615155132E-14,-1.,-3.01049762542494E-14));
#46843=DIRECTION('ref_axis',(-0.783876701585605,-8.92229719919495E-14,0.620916513479286));
#46844=DIRECTION('center_axis',(1.6283363940689E-13,-1.,6.3627469085968E-15));
#46845=DIRECTION('ref_axis',(-0.954410251348989,-1.53510827315915E-13,0.298498026995086));
#46846=DIRECTION('center_axis',(6.76186946307289E-14,-1.,8.61946552381525E-15));
#46847=DIRECTION('ref_axis',(-0.929667825095141,-6.60383262206062E-14,-0.368398880268208));
#46848=DIRECTION('center_axis',(1.01926724028163E-13,-1.,4.4055959896663E-14));
#46849=DIRECTION('ref_axis',(0.735712000031743,1.04827573753555E-13,0.677294509803005));
#46850=DIRECTION('center_axis',(4.52611277459444E-14,-1.,-3.01049762542494E-14));
#46851=DIRECTION('ref_axis',(0.145791123509555,-2.31846457713419E-14,0.989315393747526));
#46852=DIRECTION('center_axis',(-3.59257197464621E-14,-1.,1.00257629324988E-14));
#46853=DIRECTION('ref_axis',(0.954410251348985,-3.72805456675856E-14,-0.298498026995101));
#46854=DIRECTION('center_axis',(6.76186946307289E-14,-1.,8.61946552381525E-15));
#46855=DIRECTION('ref_axis',(0.929667825095138,6.60383262206061E-14,0.368398880268216));
#46856=DIRECTION('center_axis',(-5.66109027953888E-14,-1.,1.00181373700227E-13));
#46857=DIRECTION('ref_axis',(0.218698251317116,-1.10136942229696E-13,-0.975792536798082));
#46858=DIRECTION('center_axis',(8.99762615155134E-14,-1.,-3.01049762542516E-14));
#46859=DIRECTION('ref_axis',(0.783876701585584,8.922297199195E-14,-0.620916513479312));
#46860=DIRECTION('center_axis',(0.866025403784441,6.28692400828614E-14,
0.499999999999996));
#46861=DIRECTION('ref_axis',(-6.76186946307289E-14,1.,-8.61946552381525E-15));
#46862=DIRECTION('',(-0.500000000000018,-2.63446712046976E-14,0.866025403784428));
#46863=DIRECTION('',(6.76186946307289E-14,-1.,8.61946552381525E-15));
#46864=DIRECTION('',(-0.499999999999999,-2.63446712046962E-14,0.866025403784439));
#46865=DIRECTION('center_axis',(2.76820162751153E-15,8.61946552381544E-15,
1.));
#46866=DIRECTION('ref_axis',(-6.76186946307289E-14,1.,-8.61946552381525E-15));
#46867=DIRECTION('',(-1.,-6.76186946307289E-14,2.76820162751211E-15));
#46868=DIRECTION('',(-1.,-6.76186946307289E-14,2.76820162751211E-15));
#46869=DIRECTION('center_axis',(3.81897507906258E-14,-1.,-3.71109083284009E-14));
#46870=DIRECTION('ref_axis',(-0.735712000031729,-2.96164347025554E-15,-0.67729450980302));
#46871=DIRECTION('center_axis',(4.52611277459447E-14,-1.,-3.01049762542507E-14));
#46872=DIRECTION('ref_axis',(-0.145791123509541,2.31846457713439E-14,-0.989315393747528));
#46873=DIRECTION('center_axis',(-6.76186946307289E-14,1.,-8.61946552381525E-15));
#46874=DIRECTION('ref_axis',(-2.76820162751153E-15,-8.61946552381544E-15,
-1.));
#46875=DIRECTION('center_axis',(0.866025403784432,5.42497745590455E-14,
-0.500000000000011));
#46876=DIRECTION('ref_axis',(6.76186946307289E-14,-1.,8.61946552381525E-15));
#46877=DIRECTION('',(0.499999999999968,4.12740234260306E-14,0.866025403784457));
#46878=DIRECTION('',(6.76186946307289E-14,-1.,8.61946552381525E-15));
#46879=DIRECTION('',(0.5,4.12740234260326E-14,0.866025403784438));
#46880=DIRECTION('',(6.76186946307289E-14,-1.,8.61946552381525E-15));
#46881=DIRECTION('center_axis',(-2.76820162751153E-15,-8.61946552381544E-15,
-1.));
#46882=DIRECTION('ref_axis',(6.76186946307289E-14,-1.,8.61946552381525E-15));
#46883=DIRECTION('',(1.,6.76186946307289E-14,-2.76820162751211E-15));
#46884=DIRECTION('',(1.,6.76186946307289E-14,-2.76820162751211E-15));
#46885=DIRECTION('',(6.76186946307289E-14,-1.,8.61946552381525E-15));
#46886=DIRECTION('center_axis',(-0.866025403784448,-6.28692400828618E-14,
-0.499999999999984));
#46887=DIRECTION('ref_axis',(6.76186946307289E-14,-1.,8.61946552381525E-15));
#46888=DIRECTION('',(0.499999999999689,2.63446712046737E-14,-0.866025403784618));
#46889=DIRECTION('',(0.499999999999926,2.63446712046909E-14,-0.866025403784482));
#46890=DIRECTION('',(6.76186946307289E-14,-1.,8.61946552381525E-15));
#46891=DIRECTION('center_axis',(-0.866025403784445,-5.42497745590466E-14,
0.499999999999988));
#46892=DIRECTION('ref_axis',(6.76186946307289E-14,-1.,8.61946552381525E-15));
#46893=DIRECTION('',(-0.499999999999693,-4.12740234260134E-14,-0.866025403784616));
#46894=DIRECTION('',(-0.499999999999929,-4.12740234260282E-14,-0.866025403784479));
#46895=DIRECTION('',(6.76186946307289E-14,-1.,8.61946552381525E-15));
#46896=DIRECTION('center_axis',(-2.89017677254347E-14,-1.,-4.80410785544967E-13));
#46897=DIRECTION('ref_axis',(-0.218698251317561,-4.62460493070496E-13,0.975792536797982));
#46898=DIRECTION('center_axis',(6.76186946307289E-14,-1.,8.61946552381525E-15));
#46899=DIRECTION('ref_axis',(-0.78387670158548,-4.76527508315479E-14,0.620916513479444));
#46900=DIRECTION('center_axis',(5.90197180282114E-13,-1.,8.61724231507531E-15));
#46901=DIRECTION('ref_axis',(-0.954410251348957,-5.60718009349308E-13,0.29849802699519));
#46902=DIRECTION('center_axis',(6.76186946307289E-14,-1.,8.61946552381525E-15));
#46903=DIRECTION('ref_axis',(-0.929667825095052,-6.60383262206021E-14,-0.368398880268433));
#46904=DIRECTION('center_axis',(2.6777905538118E-13,-1.,2.85289344946059E-13));
#46905=DIRECTION('ref_axis',(0.735712000031681,3.90233171438362E-13,0.677294509803073));
#46906=DIRECTION('center_axis',(6.76186946307289E-14,-1.,8.61946552381525E-15));
#46907=DIRECTION('ref_axis',(0.145791123509563,1.83855753890505E-14,0.989315393747524));
#46908=DIRECTION('center_axis',(-3.756532448168E-13,-1.,8.55192630619435E-15));
#46909=DIRECTION('ref_axis',(0.95441025134894,-3.61080040935055E-13,-0.298498026995244));
#46910=DIRECTION('center_axis',(6.76186946307289E-14,-1.,8.61946552381525E-15));
#46911=DIRECTION('ref_axis',(0.929667825095137,6.6038326220606E-14,0.368398880268219));
#46912=DIRECTION('center_axis',(1.00002048887206E-13,-1.,-1.99696937105634E-15));
#46913=DIRECTION('ref_axis',(0.218698251317296,2.38189010282698E-14,-0.975792536798041));
#46914=DIRECTION('center_axis',(6.76186946307289E-14,-1.,8.61946552381525E-15));
#46915=DIRECTION('ref_axis',(0.783876701585569,4.76527508315549E-14,-0.620916513479332));
#46916=DIRECTION('center_axis',(0.866025403784435,6.28692400828611E-14,
0.500000000000006));
#46917=DIRECTION('ref_axis',(-6.76186946307289E-14,1.,-8.61946552381525E-15));
#46918=DIRECTION('',(-0.499999999999964,-2.63446712046937E-14,0.86602540378446));
#46919=DIRECTION('',(6.76186946307289E-14,-1.,8.61946552381525E-15));
#46920=DIRECTION('',(-0.499999999999995,-2.63446712046959E-14,0.866025403784442));
#46921=DIRECTION('center_axis',(2.76820162751153E-15,8.61946552381544E-15,
1.));
#46922=DIRECTION('ref_axis',(-6.76186946307289E-14,1.,-8.61946552381525E-15));
#46923=DIRECTION('',(-1.,-6.76186946307289E-14,2.76820162751211E-15));
#46924=DIRECTION('',(-1.,-6.76186946307289E-14,2.76820162751211E-15));
#46925=DIRECTION('center_axis',(-5.10570936524672E-13,-1.,-3.40477006188309E-13));
#46926=DIRECTION('ref_axis',(-0.735712000031916,6.06236371874177E-13,-0.677294509802817));
#46927=DIRECTION('center_axis',(6.76186946307289E-14,-1.,8.61946552381525E-15));
#46928=DIRECTION('ref_axis',(-0.145791123509724,-1.83855753890612E-14,-0.989315393747501));
#46929=DIRECTION('center_axis',(-6.76186946307289E-14,1.,-8.61946552381525E-15));
#46930=DIRECTION('ref_axis',(-2.76820162751153E-15,-8.61946552381544E-15,
-1.));
#46931=DIRECTION('center_axis',(-0.707106781186558,-5.39085200304648E-14,
-0.707106781186537));
#46932=DIRECTION('ref_axis',(6.76186946307289E-14,-1.,8.61946552381525E-15));
#46933=DIRECTION('',(0.707106781186545,4.17187549862772E-14,-0.70710678118655));
#46934=DIRECTION('',(-6.76186946307289E-14,1.,-8.61946552381525E-15));
#46935=DIRECTION('center_axis',(-1.,-6.76186946307289E-14,2.76820162751211E-15));
#46936=DIRECTION('ref_axis',(6.76186946307289E-14,-1.,8.61946552381525E-15));
#46937=DIRECTION('',(-6.76186946307289E-14,1.,-8.61946552381525E-15));
#46938=DIRECTION('',(-6.76186946307289E-14,1.,-8.61946552381525E-15));
#46939=DIRECTION('',(-2.76820162751153E-15,-8.61946552381544E-15,-1.));
#46940=DIRECTION('center_axis',(-0.707106781186553,-4.17187549862778E-14,
0.707106781186542));
#46941=DIRECTION('ref_axis',(-6.76186946307289E-14,1.,-8.61946552381525E-15));
#46942=DIRECTION('',(-6.76186946307289E-14,1.,-8.61946552381525E-15));
#46943=DIRECTION('',(-0.707106781186549,-5.39085200304643E-14,-0.707106781186546));
#46944=DIRECTION('center_axis',(2.76820162751153E-15,8.61946552381544E-15,
1.));
#46945=DIRECTION('ref_axis',(-6.76186946307289E-14,1.,-8.61946552381525E-15));
#46946=DIRECTION('',(-6.76186946307289E-14,1.,-8.61946552381525E-15));
#46947=DIRECTION('',(-1.,-6.76186946307289E-14,2.76820162751211E-15));
#46948=DIRECTION('center_axis',(0.707106781186549,5.39085200304643E-14,
0.707106781186546));
#46949=DIRECTION('ref_axis',(-6.76186946307289E-14,1.,-8.61946552381525E-15));
#46950=DIRECTION('',(-6.76186946307289E-14,1.,-8.61946552381525E-15));
#46951=DIRECTION('',(-0.707106781186546,-4.17187549862773E-14,0.707106781186549));
#46952=DIRECTION('center_axis',(1.,6.76186946307289E-14,-2.76820162751211E-15));
#46953=DIRECTION('ref_axis',(-6.76186946307289E-14,1.,-8.61946552381525E-15));
#46954=DIRECTION('',(-6.76186946307289E-14,1.,-8.61946552381525E-15));
#46955=DIRECTION('',(2.76820162751153E-15,8.61946552381544E-15,1.));
#46956=DIRECTION('center_axis',(0.707106781186547,4.17187549862773E-14,
-0.707106781186548));
#46957=DIRECTION('ref_axis',(6.76186946307289E-14,-1.,8.61946552381525E-15));
#46958=DIRECTION('',(0.70710678118655,5.39085200304644E-14,0.707106781186545));
#46959=DIRECTION('center_axis',(4.671786386316E-14,-0.719339800338662,-0.694658370458986));
#46960=DIRECTION('ref_axis',(4.89631698307776E-14,-0.694658370458986,0.719339800338662));
#46961=DIRECTION('center_axis',(2.74445416328055E-14,-0.719339800338663,
-0.694658370458985));
#46962=DIRECTION('ref_axis',(-4.40030170723143E-14,-0.694658370458985,0.719339800338663));
#46963=DIRECTION('',(4.89631698307777E-14,-0.694658370458988,0.719339800338661));
#46964=DIRECTION('center_axis',(-5.05637727264981E-14,0.719339800338649,
-0.694658370458999));
#46965=DIRECTION('ref_axis',(4.49806146187151E-14,-0.694658370458999,-0.719339800338649));
#46966=DIRECTION('',(4.49806146187153E-14,-0.694658370459002,-0.719339800338646));
#46967=DIRECTION('center_axis',(-6.62058893192496E-14,0.719339800338649,
-0.694658370458999));
#46968=DIRECTION('ref_axis',(-1.53038824229755E-13,0.694658370458999,0.719339800338649));
#46969=DIRECTION('center_axis',(-2.80868565487176E-15,-1.41842548064666E-14,
-1.));
#46970=DIRECTION('ref_axis',(-0.725826090825681,-0.687878249312123,1.17956576933031E-14));
#46971=DIRECTION('center_axis',(-6.72195880142588E-14,6.28549570584167E-14,
-1.));
#46972=DIRECTION('ref_axis',(-7.55372801463421E-14,1.,6.28549570584218E-14));
#46973=DIRECTION('center_axis',(-2.76820162751178E-15,-6.59025840835834E-15,
-1.));
#46974=DIRECTION('ref_axis',(0.723116678427596,-0.690725900325043,2.55032940638382E-15));
#46975=DIRECTION('center_axis',(2.93997442168891E-14,-8.30723103291069E-13,
-1.));
#46976=DIRECTION('ref_axis',(-0.60420794012745,0.796826684472191,-6.79705895003432E-13));
#46977=DIRECTION('center_axis',(-2.76820162751272E-15,2.47371373313956E-15,
-1.));
#46978=DIRECTION('ref_axis',(0.723116678427503,0.69072590032514,-2.93074620635121E-16));
#46979=DIRECTION('center_axis',(2.76820162751153E-15,8.61946552381544E-15,
1.));
#46980=DIRECTION('ref_axis',(-6.76186946307289E-14,1.,-8.61946552381525E-15));
#46981=DIRECTION('',(6.76186946307289E-14,-1.,8.61946552381525E-15));
#46982=DIRECTION('',(0.86602540378447,-0.499999999999946,1.91239982968476E-15));
#46983=DIRECTION('',(0.866025403784402,0.500000000000063,-6.70706569413058E-15));
#46984=DIRECTION('',(-6.76186946307289E-14,1.,-8.61946552381525E-15));
#46985=DIRECTION('',(-0.866025403784484,0.499999999999922,-1.9123998296845E-15));
#46986=DIRECTION('',(-0.866025403784416,-0.500000000000039,6.7070656941304E-15));
#46987=DIRECTION('center_axis',(0.500000000000052,-0.866025403784409,6.08057529691215E-15));
#46988=DIRECTION('ref_axis',(2.76820162751153E-15,8.61946552381544E-15,
1.));
#46989=DIRECTION('',(-0.866025403784416,-0.500000000000039,6.7070656941304E-15));
#46990=DIRECTION('',(2.76820162751153E-15,8.61946552381544E-15,1.));
#46991=DIRECTION('',(2.76820162751153E-15,8.61946552381544E-15,1.));
#46992=DIRECTION('center_axis',(-0.499999999999935,-0.866025403784476,8.84877692442422E-15));
#46993=DIRECTION('ref_axis',(2.76820162751153E-15,8.61946552381544E-15,
1.));
#46994=DIRECTION('',(-0.866025403784484,0.499999999999922,-1.9123998296845E-15));
#46995=DIRECTION('',(2.76820162751153E-15,8.61946552381544E-15,1.));
#46996=DIRECTION('center_axis',(-1.,-6.76186946307289E-14,2.76820162751211E-15));
#46997=DIRECTION('ref_axis',(6.76186946307289E-14,-1.,8.61946552381525E-15));
#46998=DIRECTION('',(2.76820162751153E-15,8.61946552381544E-15,1.));
#46999=DIRECTION('',(6.76186946307289E-14,-1.,8.61946552381525E-15));
#47000=DIRECTION('center_axis',(-0.500000000000052,0.866025403784409,-6.08057529691215E-15));
#47001=DIRECTION('ref_axis',(-2.76820162751153E-15,-8.61946552381544E-15,
-1.));
#47002=DIRECTION('',(0.866025403784402,0.500000000000063,-6.70706569413058E-15));
#47003=DIRECTION('',(2.76820162751153E-15,8.61946552381544E-15,1.));
#47004=DIRECTION('center_axis',(0.499999999999935,0.866025403784476,-8.84877692442422E-15));
#47005=DIRECTION('ref_axis',(-2.76820162751153E-15,-8.61946552381544E-15,
-1.));
#47006=DIRECTION('',(0.86602540378447,-0.499999999999946,1.91239982968476E-15));
#47007=DIRECTION('',(2.76820162751153E-15,8.61946552381544E-15,1.));
#47008=DIRECTION('center_axis',(1.,6.76186946307289E-14,-2.76820162751211E-15));
#47009=DIRECTION('ref_axis',(-6.76186946307289E-14,1.,-8.61946552381525E-15));
#47010=DIRECTION('',(6.76186946307289E-14,-1.,8.61946552381525E-15));
#47011=DIRECTION('center_axis',(1.81869877965002E-13,-7.82952713580378E-13,
-1.));
#47012=DIRECTION('ref_axis',(0.604207940126797,-0.796826684472686,7.33764839197491E-13));
#47013=DIRECTION('center_axis',(-2.76820162751153E-15,-8.61946552381544E-15,
-1.));
#47014=DIRECTION('ref_axis',(-0.723116678427418,-0.690725900325229,7.9554208503632E-15));
#47015=DIRECTION('center_axis',(2.76820162751153E-15,8.61946552381544E-15,
1.));
#47016=DIRECTION('ref_axis',(-6.76186946307289E-14,1.,-8.61946552381525E-15));
#47017=DIRECTION('center_axis',(2.76820162751153E-15,8.61946552381544E-15,
1.));
#47018=DIRECTION('ref_axis',(-6.76186946307289E-14,1.,-8.61946552381525E-15));
#47019=DIRECTION('',(6.76186946307289E-14,-1.,8.61946552381525E-15));
#47020=DIRECTION('',(0.86602540378447,-0.499999999999946,1.91239982968475E-15));
#47021=DIRECTION('',(0.866025403784403,0.500000000000063,-6.70706569413057E-15));
#47022=DIRECTION('',(-6.76186946307289E-14,1.,-8.61946552381525E-15));
#47023=DIRECTION('',(-0.866025403784483,0.499999999999923,-1.91239982968452E-15));
#47024=DIRECTION('',(-0.866025403784416,-0.50000000000004,6.70706569413041E-15));
#47025=DIRECTION('center_axis',(0.500000000000042,-0.866025403784415,6.08057529691222E-15));
#47026=DIRECTION('ref_axis',(2.76820162751153E-15,8.61946552381544E-15,
1.));
#47027=DIRECTION('',(-0.866025403784416,-0.50000000000004,6.70706569413041E-15));
#47028=DIRECTION('',(2.76820162751153E-15,8.61946552381544E-15,1.));
#47029=DIRECTION('',(2.76820162751153E-15,8.61946552381544E-15,1.));
#47030=DIRECTION('center_axis',(-0.499999999999925,-0.866025403784482,8.84877692442425E-15));
#47031=DIRECTION('ref_axis',(2.76820162751153E-15,8.61946552381544E-15,
1.));
#47032=DIRECTION('',(-0.866025403784483,0.499999999999923,-1.91239982968452E-15));
#47033=DIRECTION('',(2.76820162751153E-15,8.61946552381544E-15,1.));
#47034=DIRECTION('center_axis',(-1.,-6.76186946307289E-14,2.76820162751211E-15));
#47035=DIRECTION('ref_axis',(6.76186946307289E-14,-1.,8.61946552381525E-15));
#47036=DIRECTION('',(2.76820162751153E-15,8.61946552381544E-15,1.));
#47037=DIRECTION('',(6.76186946307289E-14,-1.,8.61946552381525E-15));
#47038=DIRECTION('center_axis',(-0.500000000000067,0.8660254037844,-6.08057529691203E-15));
#47039=DIRECTION('ref_axis',(-2.76820162751153E-15,-8.61946552381544E-15,
-1.));
#47040=DIRECTION('',(0.866025403784403,0.500000000000063,-6.70706569413057E-15));
#47041=DIRECTION('',(2.76820162751153E-15,8.61946552381544E-15,1.));
#47042=DIRECTION('center_axis',(0.499999999999949,0.866025403784468,-8.84877692442419E-15));
#47043=DIRECTION('ref_axis',(-2.76820162751153E-15,-8.61946552381544E-15,
-1.));
#47044=DIRECTION('',(0.86602540378447,-0.499999999999946,1.91239982968475E-15));
#47045=DIRECTION('',(2.76820162751153E-15,8.61946552381544E-15,1.));
#47046=DIRECTION('center_axis',(1.,6.76186946307289E-14,-2.76820162751211E-15));
#47047=DIRECTION('ref_axis',(-6.76186946307289E-14,1.,-8.61946552381525E-15));
#47048=DIRECTION('',(6.76186946307289E-14,-1.,8.61946552381525E-15));
#47049=DIRECTION('center_axis',(-1.41326950697088E-14,6.61744312041589E-15,
-1.));
#47050=DIRECTION('ref_axis',(1.00411787721427E-13,-1.,-6.61744312041731E-15));
#47051=DIRECTION('center_axis',(-2.76820162751153E-15,-8.61946552381544E-15,
-1.));
#47052=DIRECTION('ref_axis',(-0.723116678427638,0.690725900324999,-3.95195531815359E-15));
#47053=DIRECTION('center_axis',(2.76820162751153E-15,8.61946552381544E-15,
1.));
#47054=DIRECTION('ref_axis',(-6.76186946307289E-14,1.,-8.61946552381525E-15));
#47055=DIRECTION('center_axis',(-0.500000000000092,-4.12740234260384E-14,
-0.866025403784385));
#47056=DIRECTION('ref_axis',(6.76186946307289E-14,-1.,8.61946552381525E-15));
#47057=DIRECTION('',(6.76186946307289E-14,-1.,8.61946552381525E-15));
#47058=DIRECTION('',(-0.866025403784434,-5.42497745590456E-14,0.500000000000009));
#47059=DIRECTION('center_axis',(-1.,-6.76186946307289E-14,2.76820162751211E-15));
#47060=DIRECTION('ref_axis',(6.76186946307289E-14,-1.,8.61946552381525E-15));
#47061=DIRECTION('',(6.76186946307289E-14,-1.,8.61946552381525E-15));
#47062=DIRECTION('',(-2.76820162751153E-15,-8.61946552381544E-15,-1.));
#47063=DIRECTION('center_axis',(-0.500000000000086,-2.63446712047025E-14,
0.866025403784389));
#47064=DIRECTION('ref_axis',(-6.76186946307289E-14,1.,-8.61946552381525E-15));
#47065=DIRECTION('',(0.866025403784436,6.28692400828612E-14,0.500000000000004));
#47066=DIRECTION('center_axis',(6.76186946307289E-14,-1.,8.61946552381525E-15));
#47067=DIRECTION('ref_axis',(2.76820162751153E-15,8.61946552381544E-15,
1.));
#47068=DIRECTION('center_axis',(6.64065221755448E-14,-1.,9.21875409050844E-15));
#47069=DIRECTION('ref_axis',(0.581108581114921,4.60918619770155E-14,0.813826036051073));
#47070=DIRECTION('center_axis',(-9.65575655111783E-14,1.,-1.71288144210529E-13));
#47071=DIRECTION('ref_axis',(0.581108581115006,1.95509181315509E-13,0.813826036051013));
#47072=DIRECTION('',(0.404443987336382,-0.718054433443912,0.56641229834723));
#47073=DIRECTION('center_axis',(5.6099210001032E-16,9.3655835268151E-15,
1.));
#47074=DIRECTION('ref_axis',(0.581108581115001,-0.813826036051017,7.29595839367891E-15));
#47075=DIRECTION('',(-0.503254793602719,0.704794021481373,0.499999999999998));
#47076=DIRECTION('center_axis',(-2.76820162751153E-15,-8.61946552381544E-15,
-1.));
#47077=DIRECTION('ref_axis',(6.76186946307289E-14,-1.,8.61946552381525E-15));
#47078=DIRECTION('center_axis',(-2.76820162751153E-15,-8.61946552381544E-15,
-1.));
#47079=DIRECTION('ref_axis',(6.76186946307289E-14,-1.,8.61946552381525E-15));
#47080=DIRECTION('center_axis',(2.76820162751153E-15,8.61946552381544E-15,
1.));
#47081=DIRECTION('ref_axis',(-6.76186946307289E-14,1.,-8.61946552381525E-15));
#47082=DIRECTION('',(2.76820162751153E-15,8.61946552381544E-15,1.));
#47083=DIRECTION('center_axis',(3.69713693691E-15,-8.619465523815E-15,-1.));
#47084=DIRECTION('ref_axis',(-6.76186946307289E-14,1.,-8.61946552381525E-15));
#47085=DIRECTION('center_axis',(3.69713693691E-15,-8.619465523815E-15,-1.));
#47086=DIRECTION('ref_axis',(-6.76186946307289E-14,1.,-8.61946552381525E-15));
#47087=DIRECTION('center_axis',(4.30983829725209E-15,4.10806165286643E-16,
1.));
#47088=DIRECTION('ref_axis',(0.581108581114977,-0.813826036051033,-2.17015926467059E-15));
#47089=DIRECTION('',(-0.410905818312085,0.575461908797847,0.707106781186558));
#47090=DIRECTION('center_axis',(-2.76820162751153E-15,-8.61946552381544E-15,
-1.));
#47091=DIRECTION('ref_axis',(0.58110858111497,-0.813826036051039,5.40611974012193E-15));
#47092=DIRECTION('center_axis',(-3.59801443811168E-16,8.889746359504E-15,
1.));
#47093=DIRECTION('ref_axis',(0.581108581114948,-0.813826036051054,7.44379074775065E-15));
#47094=DIRECTION('',(-0.503254793602674,0.704794021481406,0.499999999999998));
#47095=DIRECTION('center_axis',(-2.76820162751153E-15,-8.61946552381544E-15,
-1.));
#47096=DIRECTION('ref_axis',(6.76186946307289E-14,-1.,8.61946552381525E-15));
#47097=DIRECTION('center_axis',(-2.76820162751153E-15,-8.61946552381544E-15,
-1.));
#47098=DIRECTION('ref_axis',(6.76186946307289E-14,-1.,8.61946552381525E-15));
#47099=DIRECTION('center_axis',(2.76820162751153E-15,8.61946552381544E-15,
1.));
#47100=DIRECTION('ref_axis',(-6.76186946307289E-14,1.,-8.61946552381525E-15));
#47101=DIRECTION('',(2.76820162751153E-15,8.61946552381544E-15,1.));
#47102=DIRECTION('center_axis',(3.69713693690996E-15,-8.619465523815E-15,
-1.));
#47103=DIRECTION('ref_axis',(-6.11533560663074E-14,1.,-8.61946552381523E-15));
#47104=DIRECTION('center_axis',(3.69713693690996E-15,-8.619465523815E-15,
-1.));
#47105=DIRECTION('ref_axis',(-6.11533560663074E-14,1.,-8.61946552381523E-15));
#47106=DIRECTION('center_axis',(3.29485372431133E-15,4.95596058581936E-15,
1.));
#47107=DIRECTION('ref_axis',(0.581108581114976,-0.813826036051034,2.11862198566658E-15));
#47108=DIRECTION('',(-0.410905818312097,0.575461908797867,0.707106781186535));
#47109=DIRECTION('center_axis',(-1.06388358038234E-14,-1.25106454085894E-14,
-1.));
#47110=DIRECTION('ref_axis',(0.581108581114972,-0.813826036051037,3.99917018263746E-15));
#47111=DIRECTION('center_axis',(5.88076910790884E-16,9.00223320092517E-15,
1.));
#47112=DIRECTION('ref_axis',(0.581108581115008,-0.813826036051012,6.98451522229955E-15));
#47113=DIRECTION('',(-0.503254793602725,0.704794021481369,0.499999999999999));
#47114=DIRECTION('center_axis',(-2.76820162751153E-15,-8.61946552381544E-15,
-1.));
#47115=DIRECTION('ref_axis',(6.76186946307289E-14,-1.,8.61946552381525E-15));
#47116=DIRECTION('center_axis',(-2.76820162751153E-15,-8.61946552381544E-15,
-1.));
#47117=DIRECTION('ref_axis',(6.76186946307289E-14,-1.,8.61946552381525E-15));
#47118=DIRECTION('center_axis',(2.76820162751153E-15,8.61946552381544E-15,
1.));
#47119=DIRECTION('ref_axis',(-6.76186946307289E-14,1.,-8.61946552381525E-15));
#47120=DIRECTION('',(2.76820162751153E-15,8.61946552381544E-15,1.));
#47121=DIRECTION('center_axis',(3.69713693691E-15,-8.619465523815E-15,-1.));
#47122=DIRECTION('ref_axis',(-6.76186946307289E-14,1.,-8.61946552381525E-15));
#47123=DIRECTION('center_axis',(3.69713693691E-15,-8.619465523815E-15,-1.));
#47124=DIRECTION('ref_axis',(-6.76186946307289E-14,1.,-8.61946552381525E-15));
#47125=DIRECTION('center_axis',(4.86521817410701E-15,-3.63808999178412E-15,
1.));
#47126=DIRECTION('ref_axis',(0.581108581114975,-0.813826036051035,-5.78799238678073E-15));
#47127=DIRECTION('',(-0.410905818312084,0.575461908797846,0.707106781186559));
#47128=DIRECTION('center_axis',(-1.06388358038235E-14,-1.25106454085894E-14,
-1.));
#47129=DIRECTION('ref_axis',(0.581108581114972,-0.813826036051037,3.99917018263743E-15));
#47130=DIRECTION('center_axis',(6.33479347696713E-14,-1.,5.11722901977433E-14));
#47131=DIRECTION('ref_axis',(0.581108581114944,-4.83331359671811E-15,-0.813826036051057));
#47132=DIRECTION('center_axis',(6.76186946307289E-14,-1.,8.61946552381525E-15));
#47133=DIRECTION('ref_axis',(-2.48314835913838E-14,-8.61946552381693E-15,
-1.));
#47134=DIRECTION('center_axis',(6.76186946307289E-14,-1.,8.61946552381525E-15));
#47135=DIRECTION('ref_axis',(-2.48314835913838E-14,-8.61946552381693E-15,
-1.));
#47136=DIRECTION('',(-0.410905818312021,-0.70710678118655,0.575461908797901));
#47137=DIRECTION('center_axis',(6.76186946307289E-14,-1.,8.61946552381525E-15));
#47138=DIRECTION('ref_axis',(2.76820162751153E-15,8.61946552381544E-15,
1.));
#47139=DIRECTION('center_axis',(-6.76186946307289E-14,1.,-8.61946552381525E-15));
#47140=DIRECTION('ref_axis',(-2.76820162751153E-15,-8.61946552381544E-15,
-1.));
#47141=DIRECTION('',(-6.76186946307289E-14,1.,-8.61946552381525E-15));
#47142=DIRECTION('center_axis',(6.76186946307289E-14,-1.,8.61946552381525E-15));
#47143=DIRECTION('ref_axis',(-2.48314835913838E-14,-8.61946552381693E-15,
-1.));
#47144=DIRECTION('center_axis',(6.76186946307289E-14,-1.,8.61946552381525E-15));
#47145=DIRECTION('ref_axis',(-2.48314835913838E-14,-8.61946552381693E-15,
-1.));
#47146=DIRECTION('center_axis',(7.65423745898236E-14,-1.,-2.05160675258287E-15));
#47147=DIRECTION('ref_axis',(0.581108581114976,4.61490816840534E-14,-0.813826036051034));
#47148=DIRECTION('',(-0.503254793602654,-0.500000000000061,0.704794021481375));
#47149=DIRECTION('center_axis',(6.53682722901527E-14,-1.,5.01484468347945E-14));
#47150=DIRECTION('ref_axis',(0.581108581114942,-2.82604774121214E-15,-0.813826036051058));
#47151=DIRECTION('center_axis',(6.76186946307289E-14,-1.,8.61946552381525E-15));
#47152=DIRECTION('ref_axis',(-3.63004857922531E-15,-8.6194655238155E-15,
-1.));
#47153=DIRECTION('center_axis',(6.76186946307289E-14,-1.,8.61946552381525E-15));
#47154=DIRECTION('ref_axis',(-3.63004857922531E-15,-8.6194655238155E-15,
-1.));
#47155=DIRECTION('',(-0.410905818312018,-0.707106781186553,0.5754619087979));
#47156=DIRECTION('center_axis',(6.76186946307289E-14,-1.,8.61946552381525E-15));
#47157=DIRECTION('ref_axis',(3.05202999048964E-15,8.61946552381546E-15,
1.));
#47158=DIRECTION('center_axis',(-6.76186946307289E-14,1.,-8.61946552381525E-15));
#47159=DIRECTION('ref_axis',(-1.733985285455E-15,-8.61946552381537E-15,
-1.));
#47160=DIRECTION('',(-6.76186946307289E-14,1.,-8.61946552381525E-15));
#47161=DIRECTION('center_axis',(6.76186946307289E-14,-1.,8.61946552381525E-15));
#47162=DIRECTION('ref_axis',(-3.63004857922531E-15,-8.6194655238155E-15,
-1.));
#47163=DIRECTION('center_axis',(6.76186946307289E-14,-1.,8.61946552381525E-15));
#47164=DIRECTION('ref_axis',(-3.63004857922531E-15,-8.6194655238155E-15,
-1.));
#47165=DIRECTION('center_axis',(6.78759665746252E-14,-1.,9.97879302069915E-15));
#47166=DIRECTION('ref_axis',(0.581108581114945,3.13223050593763E-14,-0.813826036051057));
#47167=DIRECTION('',(-0.503254793602635,-0.500000000000038,0.704794021481405));
#47168=DIRECTION('center_axis',(6.67758619002206E-14,-1.,4.14702793352544E-14));
#47169=DIRECTION('ref_axis',(0.581108581114937,5.05443331622382E-15,-0.813826036051062));
#47170=DIRECTION('center_axis',(6.76186946307289E-14,-1.,8.61946552381525E-15));
#47171=DIRECTION('ref_axis',(-9.49060785087889E-15,-8.61946552381589E-15,
-1.));
#47172=DIRECTION('center_axis',(6.76186946307289E-14,-1.,8.61946552381525E-15));
#47173=DIRECTION('ref_axis',(-9.49060785087889E-15,-8.61946552381589E-15,
-1.));
#47174=DIRECTION('',(-0.410905818312006,-0.707106781186571,0.575461908797887));
#47175=DIRECTION('center_axis',(6.76186946307289E-14,-1.,8.61946552381525E-15));
#47176=DIRECTION('ref_axis',(3.05202999048964E-15,8.61946552381546E-15,
1.));
#47177=DIRECTION('center_axis',(-6.76186946307289E-14,1.,-8.61946552381525E-15));
#47178=DIRECTION('ref_axis',(-2.76820162751153E-15,-8.61946552381544E-15,
-1.));
#47179=DIRECTION('',(-6.76186946307289E-14,1.,-8.61946552381525E-15));
#47180=DIRECTION('center_axis',(6.76186946307289E-14,-1.,8.61946552381525E-15));
#47181=DIRECTION('ref_axis',(-9.49060785087889E-15,-8.61946552381589E-15,
-1.));
#47182=DIRECTION('center_axis',(6.76186946307289E-14,-1.,8.61946552381525E-15));
#47183=DIRECTION('ref_axis',(-9.49060785087889E-15,-8.61946552381589E-15,
-1.));
#47184=DIRECTION('center_axis',(6.72666596076196E-14,-1.,3.72070857470792E-15));
#47185=DIRECTION('ref_axis',(0.581108581114906,3.60612236102673E-14,-0.813826036051084));
#47186=DIRECTION('',(-0.503254793602603,-0.500000000000039,0.704794021481428));
#47187=DIRECTION('center_axis',(6.32234636366842E-14,-1.,5.05743183170403E-14));
#47188=DIRECTION('ref_axis',(0.581108581114942,-4.41899975485568E-15,-0.813826036051059));
#47189=DIRECTION('center_axis',(6.76186946307289E-14,-1.,8.61946552381525E-15));
#47190=DIRECTION('ref_axis',(-1.37998426094478E-14,-8.61946552381618E-15,
-1.));
#47191=DIRECTION('center_axis',(6.76186946307289E-14,-1.,8.61946552381525E-15));
#47192=DIRECTION('ref_axis',(-1.37998426094478E-14,-8.61946552381618E-15,
-1.));
#47193=DIRECTION('',(-0.41090581831202,-0.707106781186551,0.575461908797902));
#47194=DIRECTION('center_axis',(6.76186946307289E-14,-1.,8.61946552381525E-15));
#47195=DIRECTION('ref_axis',(2.76820162751153E-15,8.61946552381544E-15,
1.));
#47196=DIRECTION('center_axis',(-6.76186946307289E-14,1.,-8.61946552381525E-15));
#47197=DIRECTION('ref_axis',(-2.76820162751153E-15,-8.61946552381544E-15,
-1.));
#47198=DIRECTION('',(-6.76186946307289E-14,1.,-8.61946552381525E-15));
#47199=DIRECTION('center_axis',(6.76186946307289E-14,-1.,8.61946552381525E-15));
#47200=DIRECTION('ref_axis',(-1.37998426094478E-14,-8.61946552381618E-15,
-1.));
#47201=DIRECTION('center_axis',(6.76186946307289E-14,-1.,8.61946552381525E-15));
#47202=DIRECTION('ref_axis',(-1.37998426094478E-14,-8.61946552381618E-15,
-1.));
#47203=DIRECTION('center_axis',(9.67592503490828E-14,-1.,2.54696229331101E-15));
#47204=DIRECTION('ref_axis',(0.581108581114985,5.41548464529684E-14,-0.813826036051028));
#47205=DIRECTION('',(-0.503254793602645,-0.500000000000086,0.704794021481363));
#47206=DIRECTION('center_axis',(1.,6.71040227609779E-14,-6.15348789557069E-15));
#47207=DIRECTION('ref_axis',(5.10351562267452E-14,-0.813826036051079,-0.581108581114913));
#47208=DIRECTION('',(0.499999999999963,0.704794021481455,0.503254793602639));
#47209=DIRECTION('center_axis',(1.,6.74942672049691E-14,2.10846237357168E-16));
#47210=DIRECTION('ref_axis',(5.50511164934163E-14,-0.813826036051077,-0.581108581114916));
#47211=DIRECTION('',(0.49999999999996,0.704794021481453,0.503254793602645));
#47212=DIRECTION('center_axis',(-1.,-6.76943554026594E-14,4.44730235615136E-15));
#47213=DIRECTION('ref_axis',(-5.76757944823519E-14,0.813826036051088,-0.581108581114901));
#47214=DIRECTION('',(-0.499999999999891,-0.704794021481494,0.503254793602656));
#47215=DIRECTION('center_axis',(-1.,-6.73743035966667E-14,2.51091843077615E-15));
#47216=DIRECTION('ref_axis',(-5.62900786743789E-14,0.813826036051049,-0.581108581114955));
#47217=DIRECTION('',(-0.499999999999892,-0.70479402148146,0.503254793602702));
#47218=DIRECTION('center_axis',(-1.,-6.88839483209371E-14,2.14531849659727E-15));
#47219=DIRECTION('ref_axis',(-5.7306213597172E-14,0.813826036051065,-0.581108581114932));
#47220=DIRECTION('',(-0.49999999999989,-0.704794021481476,0.503254793602683));
#47221=DIRECTION('center_axis',(-1.,-7.05708043906952E-14,8.00863989428406E-15));
#47222=DIRECTION('ref_axis',(-6.20862473638422E-14,0.813826036051061,-0.581108581114939));
#47223=DIRECTION('',(-0.499999999999883,-0.704794021481474,0.503254793602693));
#47224=DIRECTION('center_axis',(1.,6.77182365713367E-14,-5.15143991940756E-15));
#47225=DIRECTION('ref_axis',(5.21173180949558E-14,-0.813826036051097,-0.581108581114889));
#47226=DIRECTION('',(0.499999999999958,0.704794021481473,0.50325479360262));
#47227=DIRECTION('center_axis',(1.,6.61468802924239E-14,-1.56305132901373E-15));
#47228=DIRECTION('ref_axis',(5.29237508455151E-14,-0.813826036051071,-0.581108581114924));
#47229=DIRECTION('',(0.499999999999957,0.70479402148145,0.503254793602653));
#47230=DIRECTION('center_axis',(0.700909264299893,-0.71325044915414,4.20757949015711E-15));
#47231=DIRECTION('ref_axis',(2.76820162751153E-15,8.61946552381544E-15,
1.));
#47232=DIRECTION('',(-2.76820162751153E-15,-8.61946552381544E-15,-1.));
#47233=DIRECTION('',(-2.76820162751153E-15,-8.61946552381544E-15,-1.));
#47234=DIRECTION('',(0.713250449154132,0.700909264299901,-8.01588429312764E-15));
#47235=DIRECTION('center_axis',(0.999847695156392,-0.0174524064372163,-2.61734960140238E-15));
#47236=DIRECTION('ref_axis',(0.0174524064372163,0.999847695156392,-8.66646451737035E-15));
#47237=DIRECTION('',(-2.76820162751153E-15,-8.61946552381544E-15,-1.));
#47238=DIRECTION('',(0.0174524064372164,0.999847695156392,-8.66646451737035E-15));
#47239=DIRECTION('center_axis',(-0.99984769515639,-0.0174524064373646,2.91821043259005E-15));
#47240=DIRECTION('ref_axis',(0.0174524064373646,-0.99984769515639,8.56984095756293E-15));
#47241=DIRECTION('',(-2.76820162751153E-15,-8.61946552381544E-15,-1.));
#47242=DIRECTION('',(-2.76820162751153E-15,-8.61946552381544E-15,-1.));
#47243=DIRECTION('',(0.0174524064373627,-0.99984769515639,8.56984095756293E-15));
#47244=DIRECTION('center_axis',(0.99984769515639,0.0174524064373491,-2.91821043258992E-15));
#47245=DIRECTION('ref_axis',(-0.0174524064373491,0.99984769515639,-8.56984095756297E-15));
#47246=DIRECTION('',(-2.76820162751153E-15,-8.61946552381544E-15,-1.));
#47247=DIRECTION('',(-0.0174524064373516,0.99984769515639,-8.56984095756296E-15));
#47248=DIRECTION('center_axis',(0.700909264299797,0.713250449154235,-8.08809582250341E-15));
#47249=DIRECTION('ref_axis',(-2.76820162751153E-15,-8.61946552381544E-15,
-1.));
#47250=DIRECTION('',(-2.76820162751153E-15,-8.61946552381544E-15,-1.));
#47251=DIRECTION('',(-0.713250449154234,0.700909264299797,-4.06704218478287E-15));
#47252=DIRECTION('center_axis',(-6.76186946307289E-14,1.,-8.61946552381525E-15));
#47253=DIRECTION('ref_axis',(-2.76820162751153E-15,-8.61946552381544E-15,
-1.));
#47254=DIRECTION('',(-2.76820162751153E-15,-8.61946552381544E-15,-1.));
#47255=DIRECTION('',(-1.,-6.76186946307289E-14,2.76820162751211E-15));
#47256=DIRECTION('center_axis',(-0.700909264299919,0.713250449154115,-4.20757949015682E-15));
#47257=DIRECTION('ref_axis',(-2.76820162751153E-15,-8.61946552381544E-15,
-1.));
#47258=DIRECTION('',(-2.76820162751153E-15,-8.61946552381544E-15,-1.));
#47259=DIRECTION('',(-0.713250449154127,-0.700909264299906,8.01588429312767E-15));
#47260=DIRECTION('center_axis',(-0.999847695156392,0.0174524064372294,2.61734960140226E-15));
#47261=DIRECTION('ref_axis',(-0.0174524064372294,-0.999847695156392,8.66646451737038E-15));
#47262=DIRECTION('',(-0.0174524064372275,-0.999847695156392,8.66646451737038E-15));
#47263=DIRECTION('center_axis',(2.76820162751153E-15,8.61946552381544E-15,
1.));
#47264=DIRECTION('ref_axis',(-6.76186946307289E-14,1.,-8.61946552381525E-15));
#47265=DIRECTION('',(0.713250449154216,-0.700909264299816,4.06704218478308E-15));
#47266=DIRECTION('',(1.,6.76186946307289E-14,-2.76820162751211E-15));
#47267=DIRECTION('',(1.,6.76186946307289E-14,-2.76820162751211E-15));
#47268=DIRECTION('',(0.707106781186591,-0.707106781186504,4.13746837958802E-15));
#47269=DIRECTION('',(6.76186946307289E-14,-1.,8.61946552381525E-15));
#47270=DIRECTION('',(-0.707106781186496,-0.707106781186599,8.05229666459889E-15));
#47271=DIRECTION('',(-1.,-6.76186946307289E-14,2.76820162751211E-15));
#47272=DIRECTION('',(-0.707106781186596,0.707106781186499,-4.13746837958796E-15));
#47273=DIRECTION('',(-6.76186946307289E-14,1.,-8.61946552381525E-15));
#47274=DIRECTION('',(0.707106781186499,0.707106781186596,-8.05229666459888E-15));
#47275=DIRECTION('center_axis',(-6.76186946307289E-14,1.,-8.61946552381525E-15));
#47276=DIRECTION('ref_axis',(-2.76820162751153E-15,-8.61946552381544E-15,
-1.));
#47277=DIRECTION('center_axis',(-6.76186946307289E-14,1.,-8.61946552381525E-15));
#47278=DIRECTION('ref_axis',(2.63574839145508E-15,8.61946552381543E-15,
1.));
#47279=DIRECTION('center_axis',(-6.76186946307289E-14,1.,-8.61946552381525E-15));
#47280=DIRECTION('ref_axis',(2.38983587987361E-15,8.61946552381541E-15,
1.));
#47281=DIRECTION('center_axis',(6.76186946307289E-14,-1.,8.61946552381525E-15));
#47282=DIRECTION('ref_axis',(2.76820162751153E-15,8.61946552381544E-15,
1.));
#47283=DIRECTION('',(6.76186946307289E-14,-1.,8.61946552381525E-15));
#47284=DIRECTION('center_axis',(6.79293010634548E-14,-1.,8.57280588232624E-15));
#47285=DIRECTION('ref_axis',(0.581108581114923,4.64510723861615E-14,0.813826036051072));
#47286=DIRECTION('center_axis',(9.1381416771988E-14,-1.,1.06325780643712E-14));
#47287=DIRECTION('ref_axis',(0.581108581114925,4.44494565815108E-14,-0.813826036051071));
#47288=DIRECTION('center_axis',(-6.76186946307289E-14,1.,-8.61946552381525E-15));
#47289=DIRECTION('ref_axis',(0.581108581114916,3.22790582335802E-14,-0.813826036051077));
#47290=DIRECTION('',(-0.290554290557368,-0.866025403784476,0.406913018025524));
#47291=DIRECTION('center_axis',(-6.76186946307289E-14,1.,-8.61946552381525E-15));
#47292=DIRECTION('ref_axis',(0.581108581114917,3.22790582335802E-14,-0.813826036051077));
#47293=DIRECTION('center_axis',(-6.76186946307289E-14,1.,-8.61946552381525E-15));
#47294=DIRECTION('ref_axis',(0.581108581114916,3.22790582335802E-14,-0.813826036051077));
#47295=DIRECTION('center_axis',(-1.,-6.76186946307289E-14,2.76820162751211E-15));
#47296=DIRECTION('ref_axis',(6.76186946307289E-14,-1.,8.61946552381525E-15));
#47297=DIRECTION('center_axis',(-0.707106781186559,-5.39085200304649E-14,
-0.707106781186537));
#47298=DIRECTION('ref_axis',(6.76186946307289E-14,-1.,8.61946552381525E-15));
#47299=DIRECTION('',(0.707106781186545,4.17187549862772E-14,-0.70710678118655));
#47300=DIRECTION('center_axis',(0.707106781186545,4.17187549862772E-14,
-0.70710678118655));
#47301=DIRECTION('ref_axis',(6.76186946307289E-14,-1.,8.61946552381525E-15));
#47302=DIRECTION('',(-6.76186946307289E-14,1.,-8.61946552381525E-15));
#47303=DIRECTION('',(0.70710678118655,5.39085200304644E-14,0.707106781186545));
#47304=DIRECTION('center_axis',(1.,6.76186946307289E-14,-2.76820162751211E-15));
#47305=DIRECTION('ref_axis',(-6.76186946307289E-14,1.,-8.61946552381525E-15));
#47306=DIRECTION('',(-6.76186946307289E-14,1.,-8.61946552381525E-15));
#47307=DIRECTION('',(2.76820162751153E-15,8.61946552381544E-15,1.));
#47308=DIRECTION('center_axis',(0.707106781186549,5.39085200304643E-14,
0.707106781186546));
#47309=DIRECTION('ref_axis',(-6.76186946307289E-14,1.,-8.61946552381525E-15));
#47310=DIRECTION('',(-6.76186946307289E-14,1.,-8.61946552381525E-15));
#47311=DIRECTION('',(-0.707106781186546,-4.17187549862773E-14,0.707106781186549));
#47312=DIRECTION('center_axis',(2.76820162751153E-15,8.61946552381544E-15,
1.));
#47313=DIRECTION('ref_axis',(-6.76186946307289E-14,1.,-8.61946552381525E-15));
#47314=DIRECTION('',(-6.76186946307289E-14,1.,-8.61946552381525E-15));
#47315=DIRECTION('',(-1.,-6.76186946307289E-14,2.76820162751211E-15));
#47316=DIRECTION('center_axis',(-0.707106781186553,-4.17187549862778E-14,
0.707106781186542));
#47317=DIRECTION('ref_axis',(-6.76186946307289E-14,1.,-8.61946552381525E-15));
#47318=DIRECTION('',(-6.76186946307289E-14,1.,-8.61946552381525E-15));
#47319=DIRECTION('',(-0.707106781186549,-5.39085200304643E-14,-0.707106781186546));
#47320=DIRECTION('center_axis',(-1.,-6.76186946307289E-14,2.76820162751211E-15));
#47321=DIRECTION('ref_axis',(6.76186946307289E-14,-1.,8.61946552381525E-15));
#47322=DIRECTION('',(-2.76820162751153E-15,-8.61946552381544E-15,-1.));
#47323=DIRECTION('center_axis',(6.76186946307289E-14,-1.,8.61946552381525E-15));
#47324=DIRECTION('ref_axis',(2.76820162751153E-15,8.61946552381544E-15,
1.));
#47325=DIRECTION('center_axis',(6.76186946307289E-14,-1.,8.61946552381525E-15));
#47326=DIRECTION('ref_axis',(2.76820162751153E-15,8.61946552381544E-15,
1.));
#47327=DIRECTION('',(-2.76820162751153E-15,-8.61946552381544E-15,-1.));
#47328=DIRECTION('center_axis',(-0.700909264299829,-0.713250449154203,8.08809582250323E-15));
#47329=DIRECTION('ref_axis',(2.76820162751153E-15,8.61946552381544E-15,
1.));
#47330=DIRECTION('center_axis',(1.2292818201763E-14,7.4680920425664E-16,
-1.));
#47331=DIRECTION('ref_axis',(-0.366154256380766,-0.930554168511564,-5.19601412559431E-15));
#47332=DIRECTION('center_axis',(-2.39129758992329E-13,1.,-5.41905209207291E-14));
#47333=DIRECTION('ref_axis',(0.58110858111488,1.83062011782837E-13,0.813826036051103));
#47334=DIRECTION('center_axis',(-6.78836011028418E-14,1.,-8.61946552381525E-15));
#47335=DIRECTION('ref_axis',(2.63574839145508E-15,8.61946552381543E-15,
1.));
#47336=DIRECTION('center_axis',(-6.78836011028418E-14,1.,-8.61946552381525E-15));
#47337=DIRECTION('ref_axis',(2.63574839145508E-15,8.61946552381543E-15,
1.));
#47338=DIRECTION('',(-0.290554290557731,0.866025403784264,-0.406913018025715));
#47339=DIRECTION('center_axis',(-6.76186946307289E-14,1.,-8.61946552381525E-15));
#47340=DIRECTION('ref_axis',(-4.34309224384834E-15,-8.61946552381555E-15,
-1.));
#47341=DIRECTION('center_axis',(2.76820162751153E-15,8.61946552381544E-15,
1.));
#47342=DIRECTION('ref_axis',(-6.76186946307289E-14,1.,-8.61946552381525E-15));
#47343=DIRECTION('',(2.76820162751153E-15,8.61946552381544E-15,1.));
#47344=DIRECTION('center_axis',(1.50856361455885E-14,-2.19155353757076E-14,
1.));
#47345=DIRECTION('ref_axis',(0.581108581114967,-0.813826036051041,-2.66018258985281E-14));
#47346=DIRECTION('',(-0.290554290557446,0.406913018025467,0.866025403784476));
#47347=DIRECTION('center_axis',(-3.76067249290565E-15,-8.76855559371899E-15,
-1.));
#47348=DIRECTION('ref_axis',(0.581108581114973,-0.813826036051036,4.95071978433895E-15));
#47349=DIRECTION('center_axis',(6.76186946307289E-14,-1.,8.61946552381525E-15));
#47350=DIRECTION('ref_axis',(2.76820162751153E-15,8.61946552381544E-15,
1.));
#47351=DIRECTION('',(6.76186946307289E-14,-1.,8.61946552381525E-15));
#47352=DIRECTION('',(6.76186946307289E-14,-1.,8.61946552381525E-15));
#47353=DIRECTION('center_axis',(-4.04868893599724E-15,-9.20599848666658E-15,
-1.));
#47354=DIRECTION('ref_axis',(0.366154256380767,0.930554168511563,-1.00491249537558E-14));
#47355=DIRECTION('center_axis',(-1.72513257807643E-16,-8.12510286167748E-15,
-1.));
#47356=DIRECTION('ref_axis',(0.725826090825689,0.687878249312113,-5.71429615550167E-15));
#47357=DIRECTION('center_axis',(-6.76186946307289E-14,1.,-8.61946552381525E-15));
#47358=DIRECTION('ref_axis',(-2.76820162751153E-15,-8.61946552381544E-15,
-1.));
#47359=DIRECTION('center_axis',(6.76186946307289E-14,-1.,8.61946552381525E-15));
#47360=DIRECTION('ref_axis',(-3.14656737514945E-15,-8.61946552381546E-15,
-1.));
#47361=DIRECTION('',(-6.76186946307289E-14,1.,-8.61946552381525E-15));
#47362=DIRECTION('center_axis',(-6.76186946307289E-14,1.,-8.61946552381525E-15));
#47363=DIRECTION('ref_axis',(2.95738450133049E-15,8.61946552381545E-15,
1.));
#47364=DIRECTION('center_axis',(-4.60290999893993E-14,1.,2.77991799241815E-14));
#47365=DIRECTION('ref_axis',(0.581108581114917,4.1242085816692E-15,0.813826036051076));
#47366=DIRECTION('center_axis',(6.76186946307289E-14,-1.,8.61946552381525E-15));
#47367=DIRECTION('ref_axis',(-2.95738450133049E-15,-8.61946552381545E-15,
-1.));
#47368=DIRECTION('center_axis',(6.76186946307289E-14,-1.,8.61946552381525E-15));
#47369=DIRECTION('ref_axis',(-2.95738450133049E-15,-8.61946552381545E-15,
-1.));
#47370=DIRECTION('',(-0.290554290557484,0.866025403784451,-0.406913018025494));
#47371=DIRECTION('center_axis',(6.76771833175434E-14,-1.,8.8020274518373E-15));
#47372=DIRECTION('ref_axis',(0.58110858111492,4.64911110818535E-14,0.813826036051074));
#47373=DIRECTION('center_axis',(-6.76186946307289E-14,1.,-8.61946552381525E-15));
#47374=DIRECTION('ref_axis',(-2.76820162751153E-15,-8.61946552381544E-15,
-1.));
#47375=DIRECTION('',(0.500000000000004,4.12740234260329E-14,0.866025403784436));
#47376=DIRECTION('',(-0.499999999999999,-2.63446712046962E-14,0.866025403784439));
#47377=DIRECTION('',(-1.,-6.76186946307289E-14,2.76820162751211E-15));
#47378=DIRECTION('',(-0.500000000000002,-4.12740234260327E-14,-0.866025403784437));
#47379=DIRECTION('',(0.499999999999999,2.63446712046962E-14,-0.866025403784439));
#47380=DIRECTION('',(1.,6.76186946307289E-14,-2.76820162751211E-15));
#47381=DIRECTION('',(0.50000000000001,4.12740234260332E-14,0.866025403784433));
#47382=DIRECTION('',(-0.499999999999996,-2.6344671204696E-14,0.866025403784441));
#47383=DIRECTION('',(-1.,-6.76186946307289E-14,2.76820162751211E-15));
#47384=DIRECTION('',(-0.49999999999993,-4.12740234260283E-14,-0.866025403784479));
#47385=DIRECTION('',(0.499999999999925,2.63446712046908E-14,-0.866025403784482));
#47386=DIRECTION('',(1.,6.76186946307289E-14,-2.76820162751211E-15));
#47387=DIRECTION('center_axis',(6.76186946307289E-14,-1.,8.61946552381525E-15));
#47388=DIRECTION('ref_axis',(2.76820162751153E-15,8.61946552381544E-15,
1.));
#47389=DIRECTION('center_axis',(6.76186946307289E-14,-1.,8.61946552381525E-15));
#47390=DIRECTION('ref_axis',(-3.56323905882275E-15,-8.61946552381549E-15,
-1.));
#47391=DIRECTION('center_axis',(-6.76186946307289E-14,1.,-8.61946552381525E-15));
#47392=DIRECTION('ref_axis',(-2.76820162751153E-15,-8.61946552381544E-15,
-1.));
#47393=DIRECTION('center_axis',(-6.76186946307289E-14,1.,-8.61946552381525E-15));
#47394=DIRECTION('ref_axis',(-3.29822658171901E-15,-8.61946552381547E-15,
-1.));
#47395=DIRECTION('',(6.76186946307289E-14,-1.,8.61946552381525E-15));
#47396=DIRECTION('center_axis',(6.76186946307289E-14,-1.,8.61946552381525E-15));
#47397=DIRECTION('ref_axis',(2.76820162751153E-15,8.61946552381544E-15,
1.));
#47398=DIRECTION('center_axis',(-1.,-6.76186946307289E-14,2.76820162751211E-15));
#47399=DIRECTION('ref_axis',(2.76820162751153E-15,8.61946552381544E-15,
1.));
#47400=DIRECTION('center_axis',(1.,6.76186946307289E-14,-2.76820162751211E-15));
#47401=DIRECTION('ref_axis',(2.76820162751109E-15,1.5084804088237E-14,1.));
#47402=DIRECTION('center_axis',(1.,6.76186946307289E-14,-2.76820162751211E-15));
#47403=DIRECTION('ref_axis',(2.76820162751109E-15,1.5084804088237E-14,1.));
#47404=DIRECTION('',(-1.,-6.76186946307289E-14,2.76820162751211E-15));
#47405=DIRECTION('center_axis',(1.,6.43860253485181E-14,-2.76820162751208E-15));
#47406=DIRECTION('ref_axis',(2.76820162751111E-15,1.5084804088237E-14,1.));
#47407=DIRECTION('center_axis',(7.73833815973895E-14,-1.,3.53499671313689E-15));
#47408=DIRECTION('ref_axis',(0.581108581114921,4.20912747194277E-14,-0.813826036051074));
#47409=DIRECTION('center_axis',(-6.71511025994635E-14,1.,-8.61946552381525E-15));
#47410=DIRECTION('ref_axis',(1.13162951808259E-15,8.61946552381533E-15,
1.));
#47411=DIRECTION('center_axis',(-6.71511025994635E-14,1.,-8.61946552381525E-15));
#47412=DIRECTION('ref_axis',(1.13162951808259E-15,8.61946552381533E-15,
1.));
#47413=DIRECTION('',(0.290554290557414,0.86602540378444,-0.406913018025568));
#47414=DIRECTION('center_axis',(-6.83991273732483E-14,1.,-8.73670299263603E-15));
#47415=DIRECTION('ref_axis',(0.581108581114917,3.26371634927143E-14,-0.813826036051076));
#47416=DIRECTION('center_axis',(-6.76186946307289E-14,1.,-8.61946552381525E-15));
#47417=DIRECTION('ref_axis',(-2.76820162751153E-15,-8.61946552381544E-15,
-1.));
#47418=DIRECTION('',(-2.76820162751153E-15,-8.61946552381544E-15,-1.));
#47419=DIRECTION('',(-1.,-6.76186946307289E-14,2.76820162751211E-15));
#47420=DIRECTION('center_axis',(-6.8232481380125E-14,1.,-8.61946552381525E-15));
#47421=DIRECTION('ref_axis',(0.973373605804438,6.83914882087676E-14,0.229224395567456));
#47422=DIRECTION('',(-1.,-6.76186946307289E-14,2.76820162751211E-15));
#47423=DIRECTION('center_axis',(-7.77848709450126E-14,1.,-1.22269303430102E-14));
#47424=DIRECTION('ref_axis',(-1.,-7.77848709450126E-14,2.86757946494294E-15));
#47425=DIRECTION('center_axis',(-6.69464950962383E-14,1.,-8.61946552381525E-15));
#47426=DIRECTION('ref_axis',(0.968149047511612,6.69722803755674E-14,0.250374563009819));
#47427=DIRECTION('center_axis',(6.76186946307289E-14,-1.,8.61946552381525E-15));
#47428=DIRECTION('ref_axis',(2.76820162751153E-15,8.61946552381544E-15,
1.));
#47429=DIRECTION('center_axis',(-6.76670427534324E-14,1.,-8.468555544848E-15));
#47430=DIRECTION('ref_axis',(-0.581108581114919,-3.24299682125476E-14,0.813826036051075));
#47431=DIRECTION('center_axis',(6.76186946307289E-14,-1.,8.61946552381525E-15));
#47432=DIRECTION('ref_axis',(-1.,-6.76186946307288E-14,9.21957871251919E-15));
#47433=DIRECTION('',(6.76186946307289E-14,-1.,8.61946552381525E-15));
#47434=DIRECTION('center_axis',(-6.76186946307289E-14,1.,-8.61946552381525E-15));
#47435=DIRECTION('ref_axis',(0.968149047511612,6.76230697146222E-14,0.250374563009819));
#47436=DIRECTION('',(-6.76186946307289E-14,1.,-8.61946552381525E-15));
#47437=DIRECTION('center_axis',(-1.,-6.76186946307289E-14,2.76820162751211E-15));
#47438=DIRECTION('ref_axis',(2.76820162751153E-15,8.61946552381544E-15,
1.));
#47439=DIRECTION('center_axis',(1.,6.76186946307289E-14,-2.76820162751211E-15));
#47440=DIRECTION('ref_axis',(2.76820162751153E-15,8.61946552381544E-15,
1.));
#47441=DIRECTION('center_axis',(1.,6.76186946307289E-14,-2.76820162751211E-15));
#47442=DIRECTION('ref_axis',(2.76820162751153E-15,8.61946552381544E-15,
1.));
#47443=DIRECTION('',(-1.,-6.76186946307289E-14,2.76820162751211E-15));
#47444=DIRECTION('center_axis',(1.,6.43860253485181E-14,-2.76820162751208E-15));
#47445=DIRECTION('ref_axis',(2.76820162751153E-15,8.61946552381544E-15,
1.));
#47446=DIRECTION('center_axis',(-1.,-6.76186946307289E-14,2.76820162751211E-15));
#47447=DIRECTION('ref_axis',(6.76186946307289E-14,-1.,8.61946552381525E-15));
#47448=DIRECTION('',(6.76186946307289E-14,-1.,8.61946552381525E-15));
#47449=DIRECTION('',(6.76186946307289E-14,-1.,8.61946552381525E-15));
#47450=DIRECTION('center_axis',(-0.500000000000017,-4.12740234260337E-14,
-0.866025403784429));
#47451=DIRECTION('ref_axis',(6.76186946307289E-14,-1.,8.61946552381525E-15));
#47452=DIRECTION('',(6.76186946307289E-14,-1.,8.61946552381525E-15));
#47453=DIRECTION('',(-0.749999999999989,-0.499999999999975,0.433012701892267));
#47454=DIRECTION('',(-0.750000000000098,0.499999999999848,0.433012701892225));
#47455=DIRECTION('',(-6.76186946307289E-14,1.,-8.61946552381525E-15));
#47456=DIRECTION('',(0.749999999999838,0.500000000000272,-0.433012701892185));
#47457=DIRECTION('',(0.749999999999937,-0.50000000000015,-0.433012701892155));
#47458=DIRECTION('center_axis',(-0.433012701892109,-0.866025403784401,0.250000000000323));
#47459=DIRECTION('ref_axis',(-1.5567093557564E-14,0.277350098112963,0.960768922830422));
#47460=DIRECTION('',(0.749999999999939,-0.50000000000015,-0.433012701892152));
#47461=DIRECTION('',(-0.500000000000001,-4.12740234260327E-14,-0.866025403784438));
#47462=DIRECTION('',(-0.49999999999991,-4.12740234260269E-14,-0.866025403784491));
#47463=DIRECTION('center_axis',(0.433012701892224,-0.866025403784343,-0.250000000000326));
#47464=DIRECTION('ref_axis',(2.1760598381141E-14,-0.277350098112966,0.960768922830421));
#47465=DIRECTION('',(0.749999999999837,0.500000000000272,-0.433012701892187));
#47466=DIRECTION('',(-0.500000000000001,-4.12740234260327E-14,-0.866025403784438));
#47467=DIRECTION('center_axis',(0.866025403784435,5.42497745590457E-14,
-0.500000000000007));
#47468=DIRECTION('ref_axis',(6.76186946307289E-14,-1.,8.61946552381525E-15));
#47469=DIRECTION('',(-0.500000000000001,-4.12740234260327E-14,-0.866025403784438));
#47470=DIRECTION('',(6.76186946307289E-14,-1.,8.61946552381525E-15));
#47471=DIRECTION('center_axis',(0.433012701892244,0.866025403784463,-0.249999999999873));
#47472=DIRECTION('ref_axis',(1.56781158599937E-14,-0.277350098112484,-0.96076892283056));
#47473=DIRECTION('',(-0.750000000000077,0.499999999999834,0.433012701892277));
#47474=DIRECTION('',(-0.49999999999991,-4.12740234260269E-14,-0.866025403784491));
#47475=DIRECTION('center_axis',(-0.433012701892222,0.866025403784471,0.249999999999885));
#47476=DIRECTION('ref_axis',(-2.1552431563991E-14,0.277350098112477,-0.960768922830563));
#47477=DIRECTION('',(-0.750000000000017,-0.499999999999952,0.433012701892245));
#47478=DIRECTION('',(-0.500000000000001,-4.12740234260327E-14,-0.866025403784438));
#47479=DIRECTION('center_axis',(-0.866025403784462,-5.42497745590479E-14,
0.49999999999996));
#47480=DIRECTION('ref_axis',(6.76186946307289E-14,-1.,8.61946552381525E-15));
#47481=DIRECTION('',(6.76186946307289E-14,-1.,8.61946552381525E-15));
#47482=DIRECTION('center_axis',(1.,6.76186946307289E-14,-2.76820162751211E-15));
#47483=DIRECTION('ref_axis',(-6.76186946307289E-14,1.,-8.61946552381525E-15));
#47484=DIRECTION('',(6.76186946307289E-14,-1.,8.61946552381525E-15));
#47485=DIRECTION('',(3.14120143831326E-14,-0.499999999999871,-0.866025403784513));
#47486=DIRECTION('',(-3.62066802475778E-14,0.499999999999855,-0.866025403784522));
#47487=DIRECTION('',(-6.76186946307289E-14,1.,-8.61946552381525E-15));
#47488=DIRECTION('',(-3.14120143831563E-14,0.500000000000213,0.866025403784315));
#47489=DIRECTION('',(3.62066802476004E-14,-0.500000000000198,0.866025403784324));
#47490=DIRECTION('center_axis',(5.71754065071898E-14,-0.866025403784331,
-0.500000000000186));
#47491=DIRECTION('ref_axis',(3.62066802475997E-14,-0.500000000000186,0.866025403784331));
#47492=DIRECTION('',(3.62066802476004E-14,-0.500000000000198,0.866025403784324));
#47493=DIRECTION('',(1.,6.76186946307289E-14,-2.76820162751211E-15));
#47494=DIRECTION('',(1.,6.76186946307289E-14,-2.76820162751211E-15));
#47495=DIRECTION('center_axis',(5.99436081347026E-14,-0.866025403784325,
0.500000000000197));
#47496=DIRECTION('ref_axis',(-3.14120143831551E-14,0.500000000000197,0.866025403784325));
#47497=DIRECTION('',(-3.14120143831563E-14,0.500000000000213,0.866025403784315));
#47498=DIRECTION('',(1.,6.76186946307289E-14,-2.76820162751211E-15));
#47499=DIRECTION('center_axis',(2.76820162751153E-15,8.61946552381544E-15,
1.));
#47500=DIRECTION('ref_axis',(-6.76186946307289E-14,1.,-8.61946552381525E-15));
#47501=DIRECTION('',(1.,6.76186946307289E-14,-2.76820162751211E-15));
#47502=DIRECTION('',(6.76186946307289E-14,-1.,8.61946552381525E-15));
#47503=DIRECTION('center_axis',(-5.71754065072035E-14,0.866025403784521,
0.499999999999857));
#47504=DIRECTION('ref_axis',(-3.62066802475779E-14,0.499999999999857,-0.866025403784521));
#47505=DIRECTION('',(-3.62066802475778E-14,0.499999999999855,-0.866025403784522));
#47506=DIRECTION('',(1.,6.76186946307289E-14,-2.76820162751211E-15));
#47507=DIRECTION('center_axis',(-5.99436081347142E-14,0.86602540378451,
-0.499999999999877));
#47508=DIRECTION('ref_axis',(3.1412014383133E-14,-0.499999999999877,-0.86602540378451));
#47509=DIRECTION('',(3.14120143831326E-14,-0.499999999999871,-0.866025403784513));
#47510=DIRECTION('',(1.,6.76186946307289E-14,-2.76820162751211E-15));
#47511=DIRECTION('center_axis',(-2.76820162751153E-15,-8.61946552381544E-15,
-1.));
#47512=DIRECTION('ref_axis',(6.76186946307289E-14,-1.,8.61946552381525E-15));
#47513=DIRECTION('',(6.76186946307289E-14,-1.,8.61946552381525E-15));
#47514=DIRECTION('center_axis',(-0.500000000000004,-4.12740234260329E-14,
-0.866025403784436));
#47515=DIRECTION('ref_axis',(6.76186946307289E-14,-1.,8.61946552381525E-15));
#47516=DIRECTION('center_axis',(-0.500000000000004,-3.44554207439535E-14,
-0.866025403784436));
#47517=DIRECTION('ref_axis',(-0.704794021481385,-0.581108581114958,0.406913018025544));
#47518=DIRECTION('center_axis',(0.500000000000014,4.21542315225752E-14,
0.866025403784431));
#47519=DIRECTION('ref_axis',(-0.704794021481382,-0.581108581114953,0.406913018025557));
#47520=DIRECTION('center_axis',(-0.500000000000004,-4.71998124407273E-14,
-0.866025403784436));
#47521=DIRECTION('ref_axis',(0.866025403784436,4.89516451167878E-14,-0.500000000000004));
#47522=DIRECTION('center_axis',(-0.500000000000004,-4.71998124407273E-14,
-0.866025403784436));
#47523=DIRECTION('ref_axis',(0.866025403784436,4.89516451167878E-14,-0.500000000000004));
#47524=DIRECTION('',(-0.851918022522507,-0.410905818312109,-0.324641481296827));
#47525=DIRECTION('center_axis',(0.499999999999998,-1.34221383908382E-14,
0.86602540378444));
#47526=DIRECTION('ref_axis',(0.86602540378444,5.42497745590461E-14,-0.499999999999998));
#47527=DIRECTION('',(-0.499999999999998,1.34221383908382E-14,-0.86602540378444));
#47528=DIRECTION('center_axis',(-0.5000000000008,2.7339420210613E-14,-0.866025403783977));
#47529=DIRECTION('ref_axis',(0.704794021480816,-0.581108581115277,-0.406913018026075));
#47530=DIRECTION('center_axis',(-0.500000000000004,-3.93436929775028E-14,
-0.866025403784436));
#47531=DIRECTION('ref_axis',(0.866025403784436,5.42497745590458E-14,-0.500000000000004));
#47532=DIRECTION('center_axis',(-0.500000000000004,-3.93436929775028E-14,
-0.866025403784436));
#47533=DIRECTION('ref_axis',(0.866025403784436,5.42497745590458E-14,-0.500000000000004));
#47534=DIRECTION('',(0.851918022522704,-0.410905818312444,0.324641481295884));
#47535=DIRECTION('center_axis',(-0.500000000000002,-3.17573814987145E-14,
-0.866025403784437));
#47536=DIRECTION('ref_axis',(-0.866025403784437,1.84782918280226E-14,0.500000000000002));
#47537=DIRECTION('center_axis',(0.500000000000004,4.12740234260329E-14,
0.866025403784436));
#47538=DIRECTION('ref_axis',(-6.76186946307289E-14,1.,-8.61946552381525E-15));
#47539=DIRECTION('center_axis',(1.,6.76186946307289E-14,-2.76820162751211E-15));
#47540=DIRECTION('ref_axis',(-6.76186946307289E-14,1.,-8.61946552381525E-15));
#47541=DIRECTION('center_axis',(1.,6.75541145682558E-14,-2.96977669029757E-15));
#47542=DIRECTION('ref_axis',(3.68393940734127E-14,-0.581108581114928,-0.813826036051068));
#47543=DIRECTION('center_axis',(-1.,-6.78676766814992E-14,-1.7058558528147E-15));
#47544=DIRECTION('ref_axis',(4.08267592067223E-14,-0.581108581114911,-0.81382603605108));
#47545=DIRECTION('center_axis',(1.,6.72875615405878E-14,-2.76820162751211E-15));
#47546=DIRECTION('ref_axis',(2.76820162751153E-15,8.61946552381544E-15,
1.));
#47547=DIRECTION('center_axis',(1.,6.72875615405878E-14,-2.76820162751211E-15));
#47548=DIRECTION('ref_axis',(2.76820162751153E-15,8.61946552381544E-15,
1.));
#47549=DIRECTION('',(0.707106781186583,-0.410905818311995,-0.575461908797881));
#47550=DIRECTION('center_axis',(1.,6.76186946307289E-14,-2.76820162751211E-15));
#47551=DIRECTION('ref_axis',(-6.76186946307289E-14,1.,-8.61946552381525E-15));
#47552=DIRECTION('',(6.76186946307289E-14,-1.,8.61946552381525E-15));
#47553=DIRECTION('',(3.14120143831426E-14,-0.500000000000016,-0.866025403784429));
#47554=DIRECTION('',(-3.62066802475874E-14,0.500000000000001,-0.866025403784438));
#47555=DIRECTION('',(-6.76186946307289E-14,1.,-8.61946552381525E-15));
#47556=DIRECTION('',(-3.14120143831427E-14,0.500000000000017,0.866025403784429));
#47557=DIRECTION('',(3.62066802475875E-14,-0.500000000000002,0.866025403784437));
#47558=DIRECTION('center_axis',(5.71754065071974E-14,-0.866025403784436,
-0.500000000000004));
#47559=DIRECTION('ref_axis',(3.62066802475877E-14,-0.500000000000004,0.866025403784436));
#47560=DIRECTION('',(3.62066802475875E-14,-0.500000000000002,0.866025403784437));
#47561=DIRECTION('',(1.,6.76186946307289E-14,-2.76820162751211E-15));
#47562=DIRECTION('',(1.,6.76186946307289E-14,-2.76820162751211E-15));
#47563=DIRECTION('center_axis',(5.99436081347093E-14,-0.866025403784432,
0.500000000000012));
#47564=DIRECTION('ref_axis',(-3.14120143831423E-14,0.500000000000012,0.866025403784432));
#47565=DIRECTION('',(-3.14120143831427E-14,0.500000000000017,0.866025403784429));
#47566=DIRECTION('',(1.,6.76186946307289E-14,-2.76820162751211E-15));
#47567=DIRECTION('center_axis',(2.76820162751153E-15,8.61946552381544E-15,
1.));
#47568=DIRECTION('ref_axis',(-6.76186946307289E-14,1.,-8.61946552381525E-15));
#47569=DIRECTION('',(1.,6.76186946307289E-14,-2.76820162751211E-15));
#47570=DIRECTION('',(6.76186946307289E-14,-1.,8.61946552381525E-15));
#47571=DIRECTION('center_axis',(-5.71754065071978E-14,0.866025403784442,
0.499999999999995));
#47572=DIRECTION('ref_axis',(-3.6206680247587E-14,0.499999999999995,-0.866025403784442));
#47573=DIRECTION('',(-3.62066802475874E-14,0.500000000000001,-0.866025403784438));
#47574=DIRECTION('',(1.,6.76186946307289E-14,-2.76820162751211E-15));
#47575=DIRECTION('center_axis',(-5.99436081347093E-14,0.866025403784433,
-0.50000000000001));
#47576=DIRECTION('ref_axis',(3.14120143831422E-14,-0.50000000000001,-0.866025403784433));
#47577=DIRECTION('',(3.14120143831426E-14,-0.500000000000016,-0.866025403784429));
#47578=DIRECTION('',(1.,6.76186946307289E-14,-2.76820162751211E-15));
#47579=DIRECTION('center_axis',(-2.76820162751153E-15,-8.61946552381544E-15,
-1.));
#47580=DIRECTION('ref_axis',(6.76186946307289E-14,-1.,8.61946552381525E-15));
#47581=DIRECTION('',(6.76186946307289E-14,-1.,8.61946552381525E-15));
#47582=DIRECTION('center_axis',(-0.500000000000013,-2.63446712046972E-14,
0.866025403784431));
#47583=DIRECTION('ref_axis',(-6.76186946307289E-14,1.,-8.61946552381525E-15));
#47584=DIRECTION('',(6.76186946307289E-14,-1.,8.61946552381525E-15));
#47585=DIRECTION('',(0.750000000000005,-0.499999999999972,0.433012701892242));
#47586=DIRECTION('',(0.749999999999971,0.500000000000053,0.433012701892208));
#47587=DIRECTION('',(-6.76186946307289E-14,1.,-8.61946552381525E-15));
#47588=DIRECTION('',(-0.750000000000011,0.499999999999969,-0.433012701892236));
#47589=DIRECTION('',(-0.749999999999938,-0.500000000000081,-0.433012701892234));
#47590=DIRECTION('center_axis',(0.433012701892257,-0.866025403784422,0.249999999999993));
#47591=DIRECTION('ref_axis',(-1.60944494942364E-14,0.277350098112605,0.960768922830526));
#47592=DIRECTION('',(-0.749999999999961,-0.500000000000034,-0.433012701892248));
#47593=DIRECTION('',(-0.499999999999997,-2.63446712046961E-14,0.86602540378444));
#47594=DIRECTION('',(-0.499999999999907,-2.63446712046895E-14,0.866025403784493));
#47595=DIRECTION('center_axis',(-0.433012701892182,-0.866025403784465,-0.249999999999974));
#47596=DIRECTION('ref_axis',(2.15107982005752E-14,-0.277350098112591,0.96076892283053));
#47597=DIRECTION('',(-0.750000000000039,0.499999999999944,-0.433012701892216));
#47598=DIRECTION('',(-0.499999999999997,-2.63446712046961E-14,0.86602540378444));
#47599=DIRECTION('center_axis',(-0.866025403784437,-6.28692400828612E-14,
-0.500000000000004));
#47600=DIRECTION('ref_axis',(6.76186946307289E-14,-1.,8.61946552381525E-15));
#47601=DIRECTION('',(-0.499999999999997,-2.63446712046961E-14,0.86602540378444));
#47602=DIRECTION('',(6.76186946307289E-14,-1.,8.61946552381525E-15));
#47603=DIRECTION('center_axis',(-0.433012701892302,0.866025403784399,-0.249999999999994));
#47604=DIRECTION('ref_axis',(1.60389383430057E-14,-0.277350098112613,-0.960768922830523));
#47605=DIRECTION('',(0.749999999999971,0.500000000000053,0.433012701892208));
#47606=DIRECTION('',(-0.499999999999907,-2.63446712046895E-14,0.866025403784493));
#47607=DIRECTION('center_axis',(0.433012701892141,0.866025403784476,0.250000000000007));
#47608=DIRECTION('ref_axis',(-2.16079427152319E-14,0.277350098112621,-0.960768922830521));
#47609=DIRECTION('',(0.750000000000027,-0.499999999999986,0.433012701892189));
#47610=DIRECTION('',(-0.499999999999997,-2.63446712046961E-14,0.86602540378444));
#47611=DIRECTION('center_axis',(0.866025403784438,6.28692400828612E-14,
0.500000000000002));
#47612=DIRECTION('ref_axis',(-6.76186946307289E-14,1.,-8.61946552381525E-15));
#47613=DIRECTION('',(6.76186946307289E-14,-1.,8.61946552381525E-15));
#47614=DIRECTION('center_axis',(-0.500000000000015,-3.45211617413146E-14,
0.86602540378443));
#47615=DIRECTION('ref_axis',(-6.77071775113598E-14,1.,7.70846885918756E-16));
#47616=DIRECTION('center_axis',(-0.499999999999998,-2.0534737558427E-14,
0.86602540378444));
#47617=DIRECTION('ref_axis',(0.704794021481457,-0.581108581114873,0.406913018025541));
#47618=DIRECTION('center_axis',(0.500000000000006,2.76649833495093E-14,
-0.866025403784435));
#47619=DIRECTION('ref_axis',(0.704794021481461,-0.581108581114863,0.406913018025548));
#47620=DIRECTION('center_axis',(-0.5,-3.47395389755134E-14,0.866025403784439));
#47621=DIRECTION('ref_axis',(-0.866025403784439,-7.34654989673773E-14,-0.5));
#47622=DIRECTION('center_axis',(-0.5,-3.47395389755134E-14,0.866025403784439));
#47623=DIRECTION('ref_axis',(-0.866025403784439,-7.34654989673773E-14,-0.5));
#47624=DIRECTION('',(0.14481124133601,-0.410905818312037,0.900103390094738));
#47625=DIRECTION('center_axis',(0.500000000000089,-5.99318293989482E-14,
-0.866025403784387));
#47626=DIRECTION('ref_axis',(-0.866025403784387,-6.28692400828585E-14,-0.500000000000089));
#47627=DIRECTION('',(-0.500000000000089,5.99318293989482E-14,0.866025403784387));
#47628=DIRECTION('center_axis',(-0.500000000000155,-4.05319142052322E-14,
0.866025403784349));
#47629=DIRECTION('ref_axis',(-0.704794021481363,-0.581108581114877,-0.406913018025699));
#47630=DIRECTION('center_axis',(-0.499999999999999,-2.67123531948925E-14,
0.866025403784439));
#47631=DIRECTION('ref_axis',(-0.866025403784439,-6.61019093650721E-14,-0.499999999999999));
#47632=DIRECTION('center_axis',(-0.499999999999999,-2.67123531948925E-14,
0.866025403784439));
#47633=DIRECTION('ref_axis',(-0.866025403784439,-6.61019093650721E-14,-0.499999999999999));
#47634=DIRECTION('',(-0.144811241336241,-0.410905818312194,-0.900103390094629));
#47635=DIRECTION('center_axis',(-0.499999999999998,-1.72125400623194E-14,
0.86602540378444));
#47636=DIRECTION('ref_axis',(0.86602540378444,6.28692400828614E-14,0.499999999999998));
#47637=DIRECTION('center_axis',(0.5,2.63446712046963E-14,-0.866025403784439));
#47638=DIRECTION('ref_axis',(6.76186946307289E-14,-1.,8.61946552381525E-15));
#47639=DIRECTION('center_axis',(1.,6.76186946307289E-14,-2.76820162751211E-15));
#47640=DIRECTION('ref_axis',(-6.76186946307289E-14,1.,-8.61946552381525E-15));
#47641=DIRECTION('center_axis',(1.,6.62617941496609E-14,-2.56436653811211E-15));
#47642=DIRECTION('ref_axis',(3.64183489257448E-14,-0.581108581114924,-0.813826036051071));
#47643=DIRECTION('center_axis',(-1.,-6.70346188016559E-14,2.66648801027148E-15));
#47644=DIRECTION('ref_axis',(3.67843348498335E-14,-0.581108581114929,-0.813826036051068));
#47645=DIRECTION('center_axis',(1.,6.72875615405878E-14,-2.76820162751211E-15));
#47646=DIRECTION('ref_axis',(2.76820162751189E-15,3.32133608155747E-15,
1.));
#47647=DIRECTION('center_axis',(1.,6.72875615405878E-14,-2.76820162751211E-15));
#47648=DIRECTION('ref_axis',(2.76820162751189E-15,3.32133608155747E-15,
1.));
#47649=DIRECTION('',(0.707106781186578,-0.410905818312009,-0.575461908797876));
#47650=DIRECTION('center_axis',(-1.,-6.76186946307289E-14,2.76820162751211E-15));
#47651=DIRECTION('ref_axis',(2.76820162751153E-15,8.61946552381544E-15,
1.));
#47652=DIRECTION('',(1.,6.76186946307289E-14,-2.76820162751211E-15));
#47653=DIRECTION('center_axis',(1.,7.70213952838427E-14,-6.44756718319748E-15));
#47654=DIRECTION('ref_axis',(5.00049917717591E-14,-0.581108581114909,0.813826036051082));
#47655=DIRECTION('',(-0.707106781186518,-0.410905818312096,0.575461908797887));
#47656=DIRECTION('center_axis',(1.,6.76186946307289E-14,-2.76820162751211E-15));
#47657=DIRECTION('ref_axis',(-2.76820162751153E-15,-8.61946552381544E-15,
-1.));
#47658=DIRECTION('center_axis',(-1.,-6.76186946307289E-14,2.76820162751211E-15));
#47659=DIRECTION('ref_axis',(6.76186946307289E-14,-1.,8.61946552381525E-15));
#47660=DIRECTION('center_axis',(0.500000000000054,2.69910524079384E-14,
-0.866025403784408));
#47661=DIRECTION('ref_axis',(-0.866025403784408,-6.28692400828597E-14,-0.500000000000054));
#47662=DIRECTION('',(0.500000000000054,2.69910524079384E-14,-0.866025403784408));
#47663=DIRECTION('center_axis',(0.499999999999999,6.67723902414026E-15,
0.866025403784439));
#47664=DIRECTION('ref_axis',(0.866025403784439,5.42497745590461E-14,-0.499999999999999));
#47665=DIRECTION('',(0.499999999999999,6.67723902414026E-15,0.866025403784439));
#47666=DIRECTION('center_axis',(-1.,-6.76186946307289E-14,2.76820162751211E-15));
#47667=DIRECTION('ref_axis',(6.76186946307289E-14,-1.,8.61946552381525E-15));
#47668=DIRECTION('center_axis',(1.,6.76186946307289E-14,-2.76820162751211E-15));
#47669=DIRECTION('ref_axis',(2.76820162751108E-15,1.52311079226398E-14,
1.));
#47670=DIRECTION('center_axis',(1.,9.21118303677479E-14,-3.4270382691727E-14));
#47671=DIRECTION('ref_axis',(8.14171047488604E-14,-0.5811085811149,0.813826036051089));
#47672=DIRECTION('',(-0.707106781186463,-0.41090581831212,0.575461908797939));
#47673=DIRECTION('center_axis',(-1.,-6.76186946307289E-14,2.76820162751211E-15));
#47674=DIRECTION('ref_axis',(2.76820162751153E-15,8.61946552381544E-15,
1.));
#47675=DIRECTION('',(1.,6.76186946307289E-14,-2.76820162751211E-15));
#47676=DIRECTION('center_axis',(6.76186946307289E-14,-1.,8.61946552381525E-15));
#47677=DIRECTION('ref_axis',(2.76820162751153E-15,8.61946552381544E-15,
1.));
#47678=DIRECTION('center_axis',(-6.76186946307289E-14,1.,-8.61946552381525E-15));
#47679=DIRECTION('ref_axis',(1.13162951808259E-15,8.61946552381533E-15,
1.));
#47680=DIRECTION('center_axis',(-6.76186946307289E-14,1.,-8.61946552381525E-15));
#47681=DIRECTION('ref_axis',(1.13162951808259E-15,8.61946552381533E-15,
1.));
#47682=DIRECTION('',(-6.76186946307289E-14,1.,-8.61946552381525E-15));
#47683=DIRECTION('center_axis',(6.72348409290947E-14,-1.,8.67712845096488E-15));
#47684=DIRECTION('ref_axis',(0.581108581114924,4.61324160653485E-14,0.813826036051072));
#47685=DIRECTION('center_axis',(-6.88812930816633E-14,1.,-7.96699432180128E-15));
#47686=DIRECTION('ref_axis',(0.581108581114922,4.65112578961994E-14,0.813826036051073));
#47687=DIRECTION('',(0.290554290557519,-0.866025403784417,0.406913018025541));
#47688=DIRECTION('center_axis',(-2.76820162751153E-15,-8.61946552381544E-15,
-1.));
#47689=DIRECTION('ref_axis',(6.76186946307289E-14,-1.,8.61946552381525E-15));
#47690=DIRECTION('center_axis',(7.36346859522553E-14,-1.,2.89474361586495E-15));
#47691=DIRECTION('ref_axis',(-1.,-7.36346859522553E-14,1.39282431154371E-15));
#47692=DIRECTION('center_axis',(2.76820162751153E-15,8.61946552381544E-15,
1.));
#47693=DIRECTION('ref_axis',(-6.76186946307289E-14,1.,-8.61946552381525E-15));
#47694=DIRECTION('center_axis',(6.76186946307289E-14,-1.,8.61946552381525E-15));
#47695=DIRECTION('ref_axis',(2.76820162751153E-15,8.61946552381544E-15,
1.));
#47696=DIRECTION('center_axis',(-6.76186946307289E-14,1.,-8.61946552381525E-15));
#47697=DIRECTION('ref_axis',(-0.581108581114919,-3.22790582335804E-14,0.813826036051075));
#47698=DIRECTION('',(-6.76186946307289E-14,1.,-8.61946552381525E-15));
#47699=DIRECTION('center_axis',(-6.76186946307289E-14,1.,-8.61946552381525E-15));
#47700=DIRECTION('ref_axis',(-2.76820162751153E-15,-8.61946552381544E-15,
-1.));
#47701=DIRECTION('center_axis',(-6.76186946307289E-14,1.,-8.61946552381525E-15));
#47702=DIRECTION('ref_axis',(-0.581108581114919,-3.22790582335804E-14,0.813826036051075));
#47703=DIRECTION('center_axis',(6.76186946307289E-14,-1.,8.61946552381525E-15));
#47704=DIRECTION('ref_axis',(2.76820162751153E-15,8.61946552381544E-15,
1.));
#47705=DIRECTION('center_axis',(6.76186946307289E-14,-1.,8.61946552381525E-15));
#47706=DIRECTION('ref_axis',(-2.95738450133049E-15,-8.61946552381545E-15,
-1.));
#47707=DIRECTION('center_axis',(-6.76186946307289E-14,1.,-8.61946552381525E-15));
#47708=DIRECTION('ref_axis',(-2.76820162751153E-15,-8.61946552381544E-15,
-1.));
#47709=DIRECTION('',(6.76186946307289E-14,-1.,8.61946552381525E-15));
#47710=DIRECTION('center_axis',(6.76186946307289E-14,-1.,8.61946552381525E-15));
#47711=DIRECTION('ref_axis',(2.76820162751153E-15,8.61946552381544E-15,
1.));
#47712=DIRECTION('',(-6.76186946307289E-14,1.,-8.61946552381525E-15));
#47713=DIRECTION('center_axis',(6.76186946307289E-14,-1.,8.61946552381525E-15));
#47714=DIRECTION('ref_axis',(0.581108581114924,4.63085491538316E-14,0.813826036051072));
#47715=DIRECTION('center_axis',(6.76186946307289E-14,-1.,8.61946552381525E-15));
#47716=DIRECTION('ref_axis',(2.76820162751153E-15,8.61946552381544E-15,
1.));
#47717=DIRECTION('center_axis',(-6.76186946307289E-14,1.,-8.61946552381525E-15));
#47718=DIRECTION('ref_axis',(-2.76820162751153E-15,-8.61946552381544E-15,
-1.));
#47719=DIRECTION('center_axis',(-6.68619631354531E-14,1.,-8.61946552381525E-15));
#47720=DIRECTION('ref_axis',(-3.9032988704253E-15,-8.61946552381551E-15,
-1.));
#47721=DIRECTION('center_axis',(6.76186946307289E-14,-1.,8.61946552381525E-15));
#47722=DIRECTION('ref_axis',(-2.76820162751153E-15,-8.61946552381544E-15,
-1.));
#47723=DIRECTION('',(-6.76186946307289E-14,1.,-8.61946552381525E-15));
#47724=DIRECTION('center_axis',(-6.76186946307289E-14,1.,-8.61946552381525E-15));
#47725=DIRECTION('ref_axis',(-2.76820162751153E-15,-8.61946552381544E-15,
-1.));
#47726=DIRECTION('center_axis',(6.76186946307289E-14,-1.,8.61946552381525E-15));
#47727=DIRECTION('ref_axis',(-0.929667825095055,-6.60383262206023E-14,-0.368398880268426));
#47728=DIRECTION('',(-0.499999999999721,-4.12740234260151E-14,-0.8660254037846));
#47729=DIRECTION('center_axis',(6.76186946307289E-14,-1.,8.61946552381525E-15));
#47730=DIRECTION('ref_axis',(-0.783876701585503,-4.76527508315497E-14,0.620916513479415));
#47731=DIRECTION('',(-1.,-6.76186946307289E-14,2.76820162751211E-15));
#47732=DIRECTION('center_axis',(6.76186946307289E-14,-1.,8.61946552381525E-15));
#47733=DIRECTION('ref_axis',(0.145791123509562,1.83855753890504E-14,0.989315393747525));
#47734=DIRECTION('',(-0.499999999999992,-2.63446712046958E-14,0.866025403784443));
#47735=DIRECTION('center_axis',(6.76186946307289E-14,-1.,8.61946552381525E-15));
#47736=DIRECTION('ref_axis',(0.92966782509514,6.60383262206061E-14,0.368398880268212));
#47737=DIRECTION('',(0.499999999999997,4.12740234260324E-14,0.86602540378444));
#47738=DIRECTION('center_axis',(6.76186946307289E-14,-1.,8.61946552381525E-15));
#47739=DIRECTION('ref_axis',(0.783876701585575,4.76527508315554E-14,-0.620916513479323));
#47740=DIRECTION('',(1.,6.76186946307289E-14,-2.76820162751211E-15));
#47741=DIRECTION('center_axis',(6.76186946307289E-14,-1.,8.61946552381525E-15));
#47742=DIRECTION('ref_axis',(-0.145791123509716,-1.83855753890607E-14,-0.989315393747502));
#47743=DIRECTION('',(0.499999999999717,2.63446712046757E-14,-0.866025403784602));
#47744=DIRECTION('center_axis',(-4.76493972863412E-13,-1.,-2.89681359328052E-13));
#47745=DIRECTION('ref_axis',(-0.735712000031937,5.46761928043604E-13,-0.677294509802794));
#47746=DIRECTION('center_axis',(2.76820162751153E-15,8.61946552381544E-15,
1.));
#47747=DIRECTION('ref_axis',(-6.76186946307289E-14,1.,-8.61946552381525E-15));
#47748=DIRECTION('',(6.76186946307289E-14,-1.,8.61946552381525E-15));
#47749=DIRECTION('',(6.76186946307289E-14,-1.,8.61946552381525E-15));
#47750=DIRECTION('center_axis',(0.866025403784435,7.09853627648186E-14,
0.500000000000007));
#47751=DIRECTION('ref_axis',(-6.75709603676437E-14,1.,-2.49343890566557E-14));
#47752=DIRECTION('',(6.76186946307289E-14,-1.,8.61946552381525E-15));
#47753=DIRECTION('center_axis',(1.0103337148294E-13,-1.,-5.27593924421864E-15));
#47754=DIRECTION('ref_axis',(0.218698251317296,2.72440438071183E-14,-0.975792536798041));
#47755=DIRECTION('center_axis',(-3.69810843763156E-13,-1.,8.6039702248726E-15));
#47756=DIRECTION('ref_axis',(0.95441025134894,-3.55519528484008E-13,-0.298498026995243));
#47757=DIRECTION('center_axis',(3.12821769014316E-13,-1.,5.09998858760493E-13));
#47758=DIRECTION('ref_axis',(0.735712000031524,5.75566156379323E-13,0.677294509803243));
#47759=DIRECTION('center_axis',(6.05237314895677E-13,-1.,7.97499678325301E-15));
#47760=DIRECTION('ref_axis',(-0.954410251348955,-5.75264177030255E-13,0.298498026995197));
#47761=DIRECTION('center_axis',(-1.09246500362634E-13,-1.,-3.34895822000761E-13));
#47762=DIRECTION('ref_axis',(-0.21869825131763,-3.02896825121284E-13,0.975792536797966));
#47763=DIRECTION('center_axis',(-0.866025403784445,-5.42497745590466E-14,
0.499999999999989));
#47764=DIRECTION('ref_axis',(6.76186946307289E-14,-1.,8.61946552381525E-15));
#47765=DIRECTION('',(6.76186946307289E-14,-1.,8.61946552381525E-15));
#47766=DIRECTION('center_axis',(-0.866025403784448,-6.28692400828618E-14,
-0.499999999999984));
#47767=DIRECTION('ref_axis',(6.76186946307289E-14,-1.,8.61946552381525E-15));
#47768=DIRECTION('',(6.76186946307289E-14,-1.,8.61946552381525E-15));
#47769=DIRECTION('center_axis',(-2.76820162751153E-15,-8.61946552381544E-15,
-1.));
#47770=DIRECTION('ref_axis',(6.76186946307289E-14,-1.,8.61946552381525E-15));
#47771=DIRECTION('',(6.76186946307289E-14,-1.,8.61946552381525E-15));
#47772=DIRECTION('center_axis',(0.866025403784432,5.42497745590455E-14,
-0.500000000000011));
#47773=DIRECTION('ref_axis',(6.76186946307289E-14,-1.,8.61946552381525E-15));
#47774=DIRECTION('center_axis',(-6.76186946307289E-14,1.,-8.61946552381525E-15));
#47775=DIRECTION('ref_axis',(-2.76820162751153E-15,-8.61946552381544E-15,
-1.));
#47776=DIRECTION('center_axis',(6.76186946307289E-14,-1.,8.61946552381525E-15));
#47777=DIRECTION('ref_axis',(-0.929667825095138,-6.60383262206061E-14,-0.368398880268217));
#47778=DIRECTION('',(-0.499999999999984,-4.12740234260316E-14,-0.866025403784448));
#47779=DIRECTION('center_axis',(8.99762615155139E-14,-1.,-3.01049762542524E-14));
#47780=DIRECTION('ref_axis',(-0.783876701585578,-8.92229719919505E-14,0.62091651347932));
#47781=DIRECTION('',(-1.,-6.76186946307289E-14,2.76820162751211E-15));
#47782=DIRECTION('center_axis',(4.52611277459437E-14,-1.,-3.01049762542524E-14));
#47783=DIRECTION('ref_axis',(0.145791123509556,-2.3184645771345E-14,0.989315393747526));
#47784=DIRECTION('',(-0.49999999999999,-2.63446712046956E-14,0.866025403784444));
#47785=DIRECTION('center_axis',(6.76186946307289E-14,-1.,8.61946552381525E-15));
#47786=DIRECTION('ref_axis',(0.929667825095135,6.60383262206059E-14,0.368398880268225));
#47787=DIRECTION('',(0.499999999999995,4.12740234260323E-14,0.866025403784441));
#47788=DIRECTION('center_axis',(8.99762615155135E-14,-1.,-3.0104976254252E-14));
#47789=DIRECTION('ref_axis',(0.78387670158558,8.92229719919501E-14,-0.620916513479317));
#47790=DIRECTION('',(1.,6.76186946307289E-14,-2.76820162751211E-15));
#47791=DIRECTION('center_axis',(4.52611277459445E-14,-1.,-3.01049762542512E-14));
#47792=DIRECTION('ref_axis',(-0.145791123509541,2.31846457713444E-14,-0.989315393747528));
#47793=DIRECTION('',(0.49999999999998,2.63446712046948E-14,-0.86602540378445));
#47794=DIRECTION('center_axis',(5.32380487750437E-14,-1.,-1.68089829306692E-14));
#47795=DIRECTION('ref_axis',(-0.735712000031734,-2.77832394877596E-14,-0.677294509803015));
#47796=DIRECTION('center_axis',(2.76820162751153E-15,8.61946552381544E-15,
1.));
#47797=DIRECTION('ref_axis',(-6.76186946307289E-14,1.,-8.61946552381525E-15));
#47798=DIRECTION('',(6.76186946307289E-14,-1.,8.61946552381525E-15));
#47799=DIRECTION('',(6.76186946307289E-14,-1.,8.61946552381525E-15));
#47800=DIRECTION('center_axis',(0.866025403784442,6.28692400828615E-14,
0.499999999999994));
#47801=DIRECTION('ref_axis',(-6.76186946307289E-14,1.,-8.61946552381525E-15));
#47802=DIRECTION('',(6.76186946307289E-14,-1.,8.61946552381525E-15));
#47803=DIRECTION('center_axis',(1.07211551699132E-13,-1.,-6.00968993881945E-14));
#47804=DIRECTION('ref_axis',(0.218698251317293,8.20890847853168E-14,-0.975792536798042));
#47805=DIRECTION('center_axis',(-3.96535780483983E-13,-1.,9.14212791933769E-15));
#47806=DIRECTION('ref_axis',(0.954410251348937,-3.81186721067026E-13,-0.298498026995254));
#47807=DIRECTION('center_axis',(8.58897203906712E-14,-1.,1.09683518814373E-14));
#47808=DIRECTION('ref_axis',(0.735712000031756,7.06189024816738E-14,0.67729450980299));
#47809=DIRECTION('center_axis',(3.00772197614464E-14,-1.,7.50882472388858E-15));
#47810=DIRECTION('ref_axis',(-0.954410251349009,-2.64646375072693E-14,0.298498026995022));
#47811=DIRECTION('center_axis',(1.80859439608356E-14,-1.,6.05685967206475E-14));
#47812=DIRECTION('ref_axis',(-0.218698251317317,5.51470203266801E-14,0.975792536798037));
#47813=DIRECTION('center_axis',(-0.866025403784437,-5.42497745590459E-14,
0.500000000000003));
#47814=DIRECTION('ref_axis',(-6.76186946307289E-14,1.,-8.61946552381525E-15));
#47815=DIRECTION('',(6.76186946307289E-14,-1.,8.61946552381525E-15));
#47816=DIRECTION('center_axis',(-0.86602540378444,-6.28692400828613E-14,
-0.499999999999998));
#47817=DIRECTION('ref_axis',(6.76186946307289E-14,-1.,8.61946552381525E-15));
#47818=DIRECTION('',(6.76186946307289E-14,-1.,8.61946552381525E-15));
#47819=DIRECTION('center_axis',(-2.76820162751153E-15,-8.61946552381544E-15,
-1.));
#47820=DIRECTION('ref_axis',(6.76186946307289E-14,-1.,8.61946552381525E-15));
#47821=DIRECTION('',(6.76186946307289E-14,-1.,8.61946552381525E-15));
#47822=DIRECTION('center_axis',(0.86602540378444,5.42497745590461E-14,-0.499999999999998));
#47823=DIRECTION('ref_axis',(-6.76186946307289E-14,1.,-8.61946552381525E-15));
#47824=DIRECTION('center_axis',(2.76820162751153E-15,8.61946552381544E-15,
1.));
#47825=DIRECTION('ref_axis',(-6.76186946307289E-14,1.,-8.61946552381525E-15));
#47826=DIRECTION('center_axis',(3.53251163457694E-15,1.10051218976555E-14,
1.));
#47827=DIRECTION('ref_axis',(0.581108581114865,0.813826036051113,-1.1009027553969E-14));
#47828=DIRECTION('center_axis',(2.76820162751153E-15,8.61946552381544E-15,
1.));
#47829=DIRECTION('ref_axis',(-6.76186946307289E-14,1.,-8.61946552381525E-15));
#47830=DIRECTION('center_axis',(3.53251163457696E-15,1.10051218976555E-14,
1.));
#47831=DIRECTION('ref_axis',(0.581108581114867,0.813826036051112,-1.1009027553969E-14));
#47832=DIRECTION('center_axis',(2.76820162751153E-15,8.61946552381544E-15,
1.));
#47833=DIRECTION('ref_axis',(-6.76186946307289E-14,1.,-8.61946552381525E-15));
#47834=DIRECTION('center_axis',(-5.26130915768847E-15,9.82566750515049E-15,
1.));
#47835=DIRECTION('ref_axis',(0.581108581114855,0.813826036051121,-4.93899213784198E-15));
#47836=DIRECTION('center_axis',(-2.76820162751153E-15,-8.61946552381544E-15,
-1.));
#47837=DIRECTION('ref_axis',(6.76186946307289E-14,-1.,8.61946552381525E-15));
#47838=DIRECTION('center_axis',(2.76820162751153E-15,8.61946552381544E-15,
1.));
#47839=DIRECTION('ref_axis',(6.11533560663074E-14,-1.,8.61946552381527E-15));
#47840=DIRECTION('',(-2.76820162751153E-15,-8.61946552381544E-15,-1.));
#47841=DIRECTION('center_axis',(-3.69713693691004E-15,8.619465523815E-15,
1.));
#47842=DIRECTION('ref_axis',(6.11533560663074E-14,-1.,8.61946552381523E-15));
#47843=DIRECTION('center_axis',(-2.76820162751153E-15,-8.61946552381544E-15,
-1.));
#47844=DIRECTION('ref_axis',(6.76186946307289E-14,-1.,8.61946552381525E-15));
#47845=DIRECTION('center_axis',(2.76820162751153E-15,8.61946552381544E-15,
1.));
#47846=DIRECTION('ref_axis',(6.11533560663074E-14,-1.,8.61946552381527E-15));
#47847=DIRECTION('',(-2.76820162751153E-15,-8.61946552381544E-15,-1.));
#47848=DIRECTION('center_axis',(-3.69713693691004E-15,8.619465523815E-15,
1.));
#47849=DIRECTION('ref_axis',(6.11533560663074E-14,-1.,8.61946552381523E-15));
#47850=DIRECTION('center_axis',(-2.76820162751153E-15,-8.61946552381544E-15,
-1.));
#47851=DIRECTION('ref_axis',(6.76186946307289E-14,-1.,8.61946552381525E-15));
#47852=DIRECTION('center_axis',(-2.76820162751153E-15,-8.61946552381544E-15,
-1.));
#47853=DIRECTION('ref_axis',(6.84325727377058E-14,-1.,8.61946552381525E-15));
#47854=DIRECTION('',(-2.76820162751153E-15,-8.61946552381544E-15,-1.));
#47855=DIRECTION('center_axis',(-2.76820162751153E-15,-8.61946552381544E-15,
-1.));
#47856=DIRECTION('ref_axis',(6.76186946307289E-14,-1.,8.61946552381525E-15));
#47857=DIRECTION('center_axis',(2.76820162751153E-15,8.61946552381544E-15,
1.));
#47858=DIRECTION('ref_axis',(7.73998566779744E-14,-1.,8.61946552381522E-15));
#47859=DIRECTION('',(-2.76820162751153E-15,-8.61946552381544E-15,-1.));
#47860=DIRECTION('center_axis',(-2.12237939611116E-15,8.61946552381511E-15,
1.));
#47861=DIRECTION('ref_axis',(7.73998566779744E-14,-1.,8.61946552381527E-15));
#47862=DIRECTION('center_axis',(-2.76820162751153E-15,-8.61946552381544E-15,
-1.));
#47863=DIRECTION('ref_axis',(6.76186946307289E-14,-1.,8.61946552381525E-15));
#47864=DIRECTION('center_axis',(2.76820162751153E-15,8.61946552381544E-15,
1.));
#47865=DIRECTION('ref_axis',(7.73998566779744E-14,-1.,8.61946552381522E-15));
#47866=DIRECTION('',(-2.76820162751153E-15,-8.61946552381544E-15,-1.));
#47867=DIRECTION('center_axis',(-2.12237939611116E-15,8.61946552381511E-15,
1.));
#47868=DIRECTION('ref_axis',(7.73998566779744E-14,-1.,8.61946552381527E-15));
#47869=DIRECTION('center_axis',(-2.76820162751153E-15,-8.61946552381544E-15,
-1.));
#47870=DIRECTION('ref_axis',(6.76186946307289E-14,-1.,8.61946552381525E-15));
#47871=DIRECTION('center_axis',(2.76820162751153E-15,8.61946552381544E-15,
1.));
#47872=DIRECTION('ref_axis',(7.73998566779744E-14,-1.,8.61946552381522E-15));
#47873=DIRECTION('',(-2.76820162751153E-15,-8.61946552381544E-15,-1.));
#47874=DIRECTION('center_axis',(-2.12237939611118E-15,8.61946552381511E-15,
1.));
#47875=DIRECTION('ref_axis',(7.73998566779744E-14,-1.,8.61946552381527E-15));
#47876=DIRECTION('center_axis',(-2.76820162751153E-15,-8.61946552381544E-15,
-1.));
#47877=DIRECTION('ref_axis',(6.76186946307289E-14,-1.,8.61946552381525E-15));
#47878=DIRECTION('center_axis',(2.76820162751153E-15,8.61946552381544E-15,
1.));
#47879=DIRECTION('ref_axis',(6.76186946307289E-14,-1.,8.61946552381525E-15));
#47880=DIRECTION('',(-2.76820162751153E-15,-8.61946552381544E-15,-1.));
#47881=DIRECTION('center_axis',(-2.12237939611118E-15,8.61946552381511E-15,
1.));
#47882=DIRECTION('ref_axis',(6.76186946307289E-14,-1.,8.61946552381525E-15));
#47883=DIRECTION('center_axis',(2.76820162751153E-15,8.61946552381544E-15,
1.));
#47884=DIRECTION('ref_axis',(-6.76186946307289E-14,1.,-8.61946552381525E-15));
#47885=DIRECTION('center_axis',(8.99982368058718E-15,2.43000874453087E-14,
1.));
#47886=DIRECTION('ref_axis',(0.160984848484786,0.986956877760285,-2.54319736859329E-14));
#47887=DIRECTION('center_axis',(2.76820162751153E-15,8.61946552381544E-15,
1.));
#47888=DIRECTION('ref_axis',(0.7071067811866,-0.707106781186495,4.13746837958792E-15));
#47889=DIRECTION('',(0.7071067811865,0.707106781186595,-8.05229666459887E-15));
#47890=DIRECTION('center_axis',(-2.0472413176489E-14,6.65582873155231E-15,
1.));
#47891=DIRECTION('ref_axis',(0.578440307445775,0.815724715036904,6.41274497658531E-15));
#47892=DIRECTION('center_axis',(7.02512538336182E-15,1.92786462781398E-14,
1.));
#47893=DIRECTION('ref_axis',(0.142617449664349,0.989777885715395,-2.00834832183795E-14));
#47894=DIRECTION('center_axis',(-1.29309139275503E-14,2.67428077770542E-14,
1.));
#47895=DIRECTION('ref_axis',(-1.,6.4834541425706E-14,-1.2930913927552E-14));
#47896=DIRECTION('',(6.76186946307289E-14,-1.,8.61946552381525E-15));
#47897=DIRECTION('center_axis',(-2.37218282461776E-14,-1.38997923373325E-14,
1.));
#47898=DIRECTION('ref_axis',(-0.160984848484789,-0.986956877760285,-1.75373505727631E-14));
#47899=DIRECTION('center_axis',(-6.76186946307289E-14,1.,-8.61946552381525E-15));
#47900=DIRECTION('ref_axis',(-2.76820162751153E-15,-8.61946552381544E-15,
-1.));
#47901=DIRECTION('',(1.,6.76186946307289E-14,-2.76820162751211E-15));
#47902=DIRECTION('',(2.76820162751153E-15,8.61946552381544E-15,1.));
#47903=DIRECTION('',(1.,6.76186946307289E-14,-2.76820162751211E-15));
#47904=DIRECTION('',(2.76820162751153E-15,8.61946552381544E-15,1.));
#47905=DIRECTION('center_axis',(-2.76820162751153E-15,-8.61946552381544E-15,
-1.));
#47906=DIRECTION('ref_axis',(0.985823585943277,0.1677851524955,-4.17517679239051E-15));
#47907=DIRECTION('center_axis',(2.76820162751153E-15,8.61946552381544E-15,
1.));
#47908=DIRECTION('ref_axis',(0.985823585943276,0.167785152495509,-4.17517679239058E-15));
#47909=DIRECTION('',(2.76820162751153E-15,8.61946552381544E-15,1.));
#47910=DIRECTION('center_axis',(2.76820162751153E-15,8.61946552381544E-15,
1.));
#47911=DIRECTION('ref_axis',(0.985823585943265,0.16778515249557,-4.17517679239108E-15));
#47912=DIRECTION('center_axis',(-2.76820162751153E-15,-8.61946552381544E-15,
-1.));
#47913=DIRECTION('ref_axis',(0.815724610137237,0.578440455376742,-7.24393775608304E-15));
#47914=DIRECTION('center_axis',(2.76820162751153E-15,8.61946552381544E-15,
1.));
#47915=DIRECTION('ref_axis',(0.81572461013724,0.578440455376738,-7.24393775608301E-15));
#47916=DIRECTION('',(2.76820162751153E-15,8.61946552381544E-15,1.));
#47917=DIRECTION('center_axis',(2.76820162751153E-15,8.61946552381544E-15,
1.));
#47918=DIRECTION('ref_axis',(0.81572461013724,0.578440455376738,-7.24393775608301E-15));
#47919=DIRECTION('center_axis',(-2.76820162751153E-15,-8.61946552381544E-15,
-1.));
#47920=DIRECTION('ref_axis',(-0.7071067811866,0.707106781186495,-4.13746837958792E-15));
#47921=DIRECTION('center_axis',(2.76820162751153E-15,8.61946552381544E-15,
1.));
#47922=DIRECTION('ref_axis',(-0.70710678118656,0.707106781186535,-4.13746837958837E-15));
#47923=DIRECTION('',(2.76820162751153E-15,8.61946552381544E-15,1.));
#47924=DIRECTION('center_axis',(2.76820162751153E-15,8.61946552381544E-15,
1.));
#47925=DIRECTION('ref_axis',(-0.707106781186629,0.707106781186466,-4.13746837958759E-15));
#47926=DIRECTION('center_axis',(0.70710678118658,-0.707106781186515,4.13746837958814E-15));
#47927=DIRECTION('ref_axis',(2.76820162751153E-15,8.61946552381544E-15,
1.));
#47928=DIRECTION('',(-0.7071067811865,-0.707106781186595,8.05229666459887E-15));
#47929=DIRECTION('',(2.76820162751153E-15,8.61946552381544E-15,1.));
#47930=DIRECTION('',(-0.7071067811865,-0.707106781186595,8.05229666459887E-15));
#47931=DIRECTION('center_axis',(-2.76820162751153E-15,-8.61946552381544E-15,
-1.));
#47932=DIRECTION('ref_axis',(-0.828230928818615,-0.560386945376366,7.12294616077891E-15));
#47933=DIRECTION('center_axis',(2.76820162751153E-15,8.61946552381544E-15,
1.));
#47934=DIRECTION('ref_axis',(-0.828230928818613,-0.560386945376369,7.12294616077893E-15));
#47935=DIRECTION('',(2.76820162751153E-15,8.61946552381544E-15,1.));
#47936=DIRECTION('center_axis',(2.76820162751153E-15,8.61946552381544E-15,
1.));
#47937=DIRECTION('ref_axis',(-0.828230928818613,-0.560386945376369,7.12294616077893E-15));
#47938=DIRECTION('center_axis',(-2.76820162751153E-15,-8.61946552381544E-15,
-1.));
#47939=DIRECTION('ref_axis',(0.828230715013045,0.560387261372865,-7.12294829264291E-15));
#47940=DIRECTION('center_axis',(2.76820162751153E-15,8.61946552381544E-15,
1.));
#47941=DIRECTION('ref_axis',(0.828230715013044,0.560387261372867,-7.12294829264292E-15));
#47942=DIRECTION('',(2.76820162751153E-15,8.61946552381544E-15,1.));
#47943=DIRECTION('center_axis',(2.76820162751153E-15,8.61946552381544E-15,
1.));
#47944=DIRECTION('ref_axis',(0.828230715013044,0.560387261372867,-7.12294829264292E-15));
#47945=DIRECTION('center_axis',(-2.76820162751153E-15,-8.61946552381544E-15,
-1.));
#47946=DIRECTION('ref_axis',(-1.49010911433646E-8,-1.,8.61946556506466E-15));
#47947=DIRECTION('center_axis',(-2.02627530217484E-14,-1.92783289800561E-14,
1.));
#47948=DIRECTION('ref_axis',(-1.49010911433648E-8,-1.,-1.92783292819933E-14));
#47949=DIRECTION('center_axis',(-2.02627530217484E-14,-1.92783289800561E-14,
1.));
#47950=DIRECTION('ref_axis',(-1.49010911433648E-8,-1.,-1.92783292819933E-14));
#47951=DIRECTION('center_axis',(2.76820162751153E-15,8.61946552381544E-15,
1.));
#47952=DIRECTION('ref_axis',(-6.76186946307289E-14,1.,-8.61946552381525E-15));
#47953=DIRECTION('center_axis',(0.707106781186502,0.707106781186593,-8.05229666459886E-15));
#47954=DIRECTION('ref_axis',(-2.76820162751153E-15,-8.61946552381544E-15,
-1.));
#47955=DIRECTION('',(0.707106781186597,-0.707106781186498,4.13746837958795E-15));
#47956=DIRECTION('',(2.76820162751153E-15,8.61946552381544E-15,1.));
#47957=DIRECTION('',(0.707106781186597,-0.707106781186498,4.13746837958795E-15));
#47958=DIRECTION('',(2.76820162751153E-15,8.61946552381544E-15,1.));
#47959=DIRECTION('center_axis',(-2.76820162751153E-15,-8.61946552381544E-15,
-1.));
#47960=DIRECTION('ref_axis',(0.815724561786183,-0.578440523562051,2.72775809088321E-15));
#47961=DIRECTION('center_axis',(4.73183590111844E-15,-1.46211561682312E-14,
1.));
#47962=DIRECTION('ref_axis',(0.8157245617862,-0.578440523562027,-1.23173439959179E-14));
#47963=DIRECTION('',(2.76820162751153E-15,8.61946552381544E-15,1.));
#47964=DIRECTION('center_axis',(8.04567353904598E-16,3.18600872158624E-14,
1.));
#47965=DIRECTION('ref_axis',(0.815724561786194,-0.578440523562036,1.77728601776843E-14));
#47966=DIRECTION('center_axis',(-2.76820162751153E-15,-8.61946552381544E-15,
-1.));
#47967=DIRECTION('ref_axis',(0.985823571918322,-0.167785234899263,-1.28273936860405E-15));
#47968=DIRECTION('center_axis',(2.76820162751153E-15,8.61946552381544E-15,
1.));
#47969=DIRECTION('ref_axis',(0.985823571918322,-0.167785234899264,-1.28273936860404E-15));
#47970=DIRECTION('',(2.76820162751153E-15,8.61946552381544E-15,1.));
#47971=DIRECTION('center_axis',(1.46062076622723E-14,3.71600285032592E-15,
1.));
#47972=DIRECTION('ref_axis',(0.985823571918322,-0.167785234899264,-1.37756533986737E-14));
#47973=DIRECTION('center_axis',(-2.76820162751153E-15,-8.61946552381544E-15,
-1.));
#47974=DIRECTION('ref_axis',(-1.49013091640289E-8,1.,-8.61946548256561E-15));
#47975=DIRECTION('center_axis',(2.76820162751153E-15,8.61946552381544E-15,
1.));
#47976=DIRECTION('ref_axis',(-1.49012263807535E-8,1.,-8.61946548256584E-15));
#47977=DIRECTION('',(2.76820162751153E-15,8.61946552381544E-15,1.));
#47978=DIRECTION('center_axis',(2.76820162751153E-15,8.61946552381544E-15,
1.));
#47979=DIRECTION('ref_axis',(-1.49012263807535E-8,1.,-8.61946548256584E-15));
#47980=DIRECTION('center_axis',(6.76186946307289E-14,-1.,8.61946552381525E-15));
#47981=DIRECTION('ref_axis',(2.76820162751153E-15,8.61946552381544E-15,
1.));
#47982=DIRECTION('',(-1.,-6.76186946307289E-14,2.76820162751211E-15));
#47983=DIRECTION('',(2.76820162751153E-15,8.61946552381544E-15,1.));
#47984=DIRECTION('',(-1.,-6.76186946307289E-14,2.76820162751211E-15));
#47985=DIRECTION('center_axis',(-2.76820162751153E-15,-8.61946552381544E-15,
-1.));
#47986=DIRECTION('ref_axis',(-0.981901142050496,0.189394158410264,1.08562392065031E-15));
#47987=DIRECTION('center_axis',(2.57991596261325E-14,-1.92783397979622E-14,
1.));
#47988=DIRECTION('ref_axis',(-0.981901142050477,0.18939415841036,2.89834292424261E-14));
#47989=DIRECTION('',(2.76820162751153E-15,8.61946552381544E-15,1.));
#47990=DIRECTION('center_axis',(2.5799159626134E-14,-1.92783397979624E-14,
1.));
#47991=DIRECTION('ref_axis',(-0.981901142050477,0.189394158410364,2.89834292424276E-14));
#47992=DIRECTION('center_axis',(-2.76820162751153E-15,-8.61946552381544E-15,
-1.));
#47993=DIRECTION('ref_axis',(0.981901186307147,-0.189393928964519,-1.08562602086133E-15));
#47994=DIRECTION('center_axis',(-1.51165338862552E-14,1.60275656363945E-14,
1.));
#47995=DIRECTION('ref_axis',(0.981901186307147,-0.189393928964522,1.78784661833796E-14));
#47996=DIRECTION('',(2.76820162751153E-15,8.61946552381544E-15,1.));
#47997=DIRECTION('center_axis',(-3.30012694000219E-14,2.34356657489735E-14,
1.));
#47998=DIRECTION('ref_axis',(0.981901186307147,-0.189393928964522,3.68425583876206E-14));
#47999=DIRECTION('center_axis',(-2.92006984084315E-15,-8.46759731048387E-15,
-1.));
#48000=DIRECTION('ref_axis',(-0.707106781186433,-0.707106781186662,8.05229666459926E-15));
#48001=DIRECTION('center_axis',(3.87802855472544E-14,1.2060850989616E-14,
1.));
#48002=DIRECTION('ref_axis',(-0.707106781186464,-0.707106781186631,3.59501124084499E-14));
#48003=DIRECTION('center_axis',(3.87802855472544E-14,1.20608509896159E-14,
1.));
#48004=DIRECTION('ref_axis',(-0.707106781186467,-0.707106781186628,3.595011240845E-14));
#48005=DIRECTION('center_axis',(2.76820162751153E-15,8.61946552381544E-15,
1.));
#48006=DIRECTION('ref_axis',(-6.76186946307289E-14,1.,-8.61946552381525E-15));
#48007=DIRECTION('center_axis',(1.,6.76186946307289E-14,-2.76820162751211E-15));
#48008=DIRECTION('ref_axis',(-6.76186946307289E-14,1.,-8.61946552381525E-15));
#48009=DIRECTION('',(6.76186946307289E-14,-1.,8.61946552381525E-15));
#48010=DIRECTION('',(2.76820162751153E-15,8.61946552381544E-15,1.));
#48011=DIRECTION('',(6.76186946307289E-14,-1.,8.61946552381525E-15));
#48012=DIRECTION('',(2.76820162751153E-15,8.61946552381544E-15,1.));
#48013=DIRECTION('center_axis',(-2.76820162751153E-15,-8.61946552381544E-15,
-1.));
#48014=DIRECTION('ref_axis',(0.142617449664331,-0.989777885715397,8.13656250588646E-15));
#48015=DIRECTION('center_axis',(-1.29309139275495E-14,-9.50387672942742E-15,
1.));
#48016=DIRECTION('ref_axis',(0.142617449664151,-0.989777885715423,-7.56255304917892E-15));
#48017=DIRECTION('',(2.76820162751153E-15,8.61946552381544E-15,1.));
#48018=DIRECTION('center_axis',(2.76820162751153E-15,8.61946552381544E-15,
1.));
#48019=DIRECTION('ref_axis',(0.142617449664151,-0.989777885715423,8.13656250588718E-15));
#48020=DIRECTION('center_axis',(-2.76820162751153E-15,-8.61946552381544E-15,
-1.));
#48021=DIRECTION('ref_axis',(0.578440455376734,-0.815724610137243,5.42987034401337E-15));
#48022=DIRECTION('center_axis',(7.02512529519986E-15,-2.03971490112667E-15,
1.));
#48023=DIRECTION('ref_axis',(0.578440455376738,-0.81572461013724,-5.72746231734672E-15));
#48024=DIRECTION('',(2.76820162751153E-15,8.61946552381544E-15,1.));
#48025=DIRECTION('center_axis',(-1.4887220401768E-15,1.92786459487576E-14,
1.));
#48026=DIRECTION('ref_axis',(0.578440455376738,-0.81572461013724,1.65872030053734E-14));
#48027=DIRECTION('center_axis',(-2.76820162751153E-15,-8.61946552381544E-15,
-1.));
#48028=DIRECTION('ref_axis',(0.707106781186598,0.707106781186497,-8.0522966645983E-15));
#48029=DIRECTION('center_axis',(7.2490060184047E-14,2.72856031906688E-15,
1.));
#48030=DIRECTION('ref_axis',(0.707106781186564,0.707106781186531,-5.31875966292505E-14));
#48031=DIRECTION('',(2.76820162751153E-15,8.61946552381544E-15,1.));
#48032=DIRECTION('center_axis',(2.60088211463569E-14,6.65583045556597E-15,
1.));
#48033=DIRECTION('ref_axis',(0.707106781186583,0.707106781186512,-2.30973966528164E-14));
#48034=DIRECTION('center_axis',(-0.707106781186506,-0.707106781186589,8.05229666459883E-15));
#48035=DIRECTION('ref_axis',(2.76820162751153E-15,8.61946552381544E-15,
1.));
#48036=DIRECTION('',(-0.707106781186597,0.707106781186498,-4.13746837958795E-15));
#48037=DIRECTION('',(2.76820162751153E-15,8.61946552381544E-15,1.));
#48038=DIRECTION('',(-0.707106781186588,0.707106781186507,-4.13746837958805E-15));
#48039=DIRECTION('center_axis',(-2.76820162751153E-15,-8.61946552381544E-15,
-1.));
#48040=DIRECTION('ref_axis',(-0.560387030549914,0.828230871189579,-5.58764314997358E-15));
#48041=DIRECTION('center_axis',(-6.73179990625715E-16,-2.73926102301024E-14,
1.));
#48042=DIRECTION('ref_axis',(-0.560387030549925,0.828230871189572,2.23101640990617E-14));
#48043=DIRECTION('',(2.76820162751153E-15,8.61946552381544E-15,1.));
#48044=DIRECTION('center_axis',(-6.73179990625995E-16,-2.73926102301055E-14,
1.));
#48045=DIRECTION('ref_axis',(-0.560387030549879,0.828230871189603,2.2310164099065E-14));
#48046=DIRECTION('center_axis',(-2.76820162751153E-15,-8.61946552381544E-15,
-1.));
#48047=DIRECTION('ref_axis',(0.560387257316999,-0.828230717757276,5.58764119973211E-15));
#48048=DIRECTION('center_axis',(2.76820162751153E-15,8.61946552381544E-15,
1.));
#48049=DIRECTION('ref_axis',(0.560387257316998,-0.828230717757276,5.58764119973212E-15));
#48050=DIRECTION('',(2.76820162751153E-15,8.61946552381544E-15,1.));
#48051=DIRECTION('center_axis',(2.76820162751153E-15,8.61946552381544E-15,
1.));
#48052=DIRECTION('ref_axis',(0.560387257316998,-0.828230717757276,5.58764119973212E-15));
#48053=DIRECTION('center_axis',(-2.76820162751153E-15,-8.61946552381544E-15,
-1.));
#48054=DIRECTION('ref_axis',(-1.,-6.34795310039648E-14,2.76820162751208E-15));
#48055=DIRECTION('center_axis',(2.76820162751153E-15,8.61946552381544E-15,
1.));
#48056=DIRECTION('ref_axis',(-1.,-2.00183129229455E-14,2.7682016275117E-15));
#48057=DIRECTION('center_axis',(-2.37218282461825E-14,3.11387233849614E-14,
1.));
#48058=DIRECTION('ref_axis',(-1.,-2.00183129229458E-14,-2.37218282461819E-14));
#48059=DIRECTION('center_axis',(2.76820162751153E-15,8.61946552381544E-15,
1.));
#48060=DIRECTION('ref_axis',(-6.76186946307289E-14,1.,-8.61946552381525E-15));
#48061=DIRECTION('center_axis',(2.76820162751153E-15,8.61946552381544E-15,
1.));
#48062=DIRECTION('ref_axis',(-6.76186946307289E-14,1.,-8.61946552381525E-15));
#48063=DIRECTION('',(2.76820162751153E-15,8.61946552381544E-15,1.));
#48064=DIRECTION('center_axis',(-2.76820162751153E-15,-8.61946552381544E-15,
-1.));
#48065=DIRECTION('ref_axis',(-0.581108581114972,0.813826036051037,-5.40611974012191E-15));
#48066=DIRECTION('center_axis',(2.99566356165988E-15,8.72176871572695E-15,
1.));
#48067=DIRECTION('ref_axis',(-6.76186946307289E-14,1.,-8.72176871572675E-15));
#48068=DIRECTION('',(2.99566356165988E-15,8.72176871572695E-15,1.));
#48069=DIRECTION('center_axis',(-2.76820162751153E-15,-8.61946552381544E-15,
-1.));
#48070=DIRECTION('ref_axis',(-0.581108581114972,0.813826036051037,-5.40611974012191E-15));
#48071=DIRECTION('center_axis',(2.71915890354096E-15,8.72176871572693E-15,
1.));
#48072=DIRECTION('ref_axis',(-6.76186946307289E-14,1.,-8.72176871572675E-15));
#48073=DIRECTION('',(2.71915890354096E-15,8.72176871572693E-15,1.));
#48074=DIRECTION('center_axis',(-2.76820162751153E-15,-8.61946552381544E-15,
-1.));
#48075=DIRECTION('ref_axis',(-0.581108581114971,0.813826036051038,-5.40611974012192E-15));
#48076=DIRECTION('center_axis',(-2.76820162751153E-15,-8.61946552381544E-15,
-1.));
#48077=DIRECTION('ref_axis',(0.715652996595046,0.698456003241816,-8.00138922975266E-15));
#48078=DIRECTION('center_axis',(1.20008912487007E-15,8.61946552381533E-15,
1.));
#48079=DIRECTION('ref_axis',(0.71856952465566,0.695455130282421,-6.85679899083214E-15));
#48080=DIRECTION('center_axis',(0.999390826289479,-5.82068180765387E-7,
-0.0348995175911332));
#48081=DIRECTION('ref_axis',(0.0348985180651857,-0.00755166584133485,0.999362329578154));
#48082=DIRECTION('center_axis',(1.21617314918329E-15,8.61946552381533E-15,
1.));
#48083=DIRECTION('ref_axis',(0.715652996595047,0.698456003241815,-6.89067539843613E-15));
#48084=DIRECTION('center_axis',(0.999390826289723,5.81873952209323E-7,-0.0348995175841439));
#48085=DIRECTION('ref_axis',(0.0348985217095042,0.00753783529609301,0.999362433865482));
#48086=DIRECTION('center_axis',(2.76820162751153E-15,8.61946552381544E-15,
1.));
#48087=DIRECTION('ref_axis',(-6.76186946307289E-14,1.,-8.61946552381525E-15));
#48088=DIRECTION('',(6.76186946307289E-14,-1.,8.61946552381525E-15));
#48089=DIRECTION('center_axis',(-2.76820162751153E-15,-8.61946552381544E-15,
-1.));
#48090=DIRECTION('ref_axis',(-0.338105122691879,0.941108349771433,-7.17590782412406E-15));
#48091=DIRECTION('center_axis',(2.76820162751206E-15,7.35344329979148E-16,
1.));
#48092=DIRECTION('ref_axis',(-0.329874263976707,0.944024877832055,2.18975133141604E-16));
#48093=DIRECTION('center_axis',(1.50207726725875E-6,0.999390821854869,-0.0348996445539642));
#48094=DIRECTION('ref_axis',(-0.995051211909553,0.00346924114795279,0.0993028199155812));
#48095=DIRECTION('center_axis',(2.76820162751153E-15,8.61946552381544E-15,
1.));
#48096=DIRECTION('ref_axis',(-0.338105122691878,0.941108349771433,-7.17590782412407E-15));
#48097=DIRECTION('center_axis',(-1.50215001892545E-6,0.999390821854616,
-0.0348996445611993));
#48098=DIRECTION('ref_axis',(0.995316427551229,0.00337526453063588,0.0966116796045264));
#48099=DIRECTION('center_axis',(2.76820162751153E-15,8.61946552381544E-15,
1.));
#48100=DIRECTION('ref_axis',(-6.76186946307289E-14,1.,-8.61946552381525E-15));
#48101=DIRECTION('',(1.,6.76186946307289E-14,-2.76820162751211E-15));
#48102=DIRECTION('center_axis',(-2.76820162751153E-15,-8.61946552381544E-15,
-1.));
#48103=DIRECTION('ref_axis',(-0.715652996595035,-0.698456003241827,8.00138922975273E-15));
#48104=DIRECTION('center_axis',(-0.999390826288683,-5.82701798186421E-7,
-0.0348995176139201));
#48105=DIRECTION('ref_axis',(-0.0348985190951373,-0.00754783375989079,0.999362358491903));
#48106=DIRECTION('center_axis',(4.33631413015298E-15,8.61946552381554E-15,
1.));
#48107=DIRECTION('ref_axis',(-0.718569524655658,-0.695455130282423,9.11039470209163E-15));
#48108=DIRECTION('center_axis',(-0.999390826289037,5.82420313152883E-7,
-0.0348995176037821));
#48109=DIRECTION('ref_axis',(-0.034898520434395,0.00754272883685878,0.999362396987791));
#48110=DIRECTION('center_axis',(2.76820162751153E-15,8.61946552381544E-15,
1.));
#48111=DIRECTION('ref_axis',(-0.715652996595031,-0.69845600324183,8.00138922975275E-15));
#48112=DIRECTION('center_axis',(2.76820162751153E-15,8.61946552381544E-15,
1.));
#48113=DIRECTION('ref_axis',(-6.76186946307289E-14,1.,-8.61946552381525E-15));
#48114=DIRECTION('',(-6.76186946307289E-14,1.,-8.61946552381525E-15));
#48115=DIRECTION('center_axis',(2.76820162751153E-15,8.61946552381544E-15,
1.));
#48116=DIRECTION('ref_axis',(-6.76186946307289E-14,1.,-8.61946552381525E-15));
#48117=DIRECTION('',(-1.,-6.76186946307289E-14,2.76820162751211E-15));
#48118=DIRECTION('',(6.76186946307289E-14,-1.,8.61946552381525E-15));
#48119=DIRECTION('center_axis',(-2.02835435550342E-15,3.82290954079985E-15,
1.));
#48120=DIRECTION('ref_axis',(-6.56318960898822E-14,1.,-3.82290954079999E-15));
#48121=DIRECTION('',(1.,6.6593023648202E-14,-2.7682016275121E-15));
#48122=DIRECTION('',(-6.76186946307289E-14,1.,-8.61946552381525E-15));
#48123=DIRECTION('center_axis',(-7.79286212482761E-15,-1.36441260211324E-14,
-1.));
#48124=DIRECTION('ref_axis',(-1.,-8.20575921431216E-14,7.79286212482873E-15));
#48125=DIRECTION('center_axis',(2.76820162751153E-15,8.61946552381544E-15,
1.));
#48126=DIRECTION('ref_axis',(-6.76186946307289E-14,1.,-8.61946552381525E-15));
#48127=DIRECTION('',(1.,6.76186946307289E-14,-2.76820162751211E-15));
#48128=DIRECTION('center_axis',(-2.76820162751153E-15,-8.61946552381544E-15,
-1.));
#48129=DIRECTION('ref_axis',(-5.72122820091847E-14,1.,-8.61946552381528E-15));
#48130=DIRECTION('',(-6.76186946307289E-14,1.,-8.61946552381525E-15));
#48131=DIRECTION('',(-1.,-6.76186946307289E-14,2.76820162751211E-15));
#48132=DIRECTION('center_axis',(2.76820162751153E-15,8.61946552381544E-15,
1.));
#48133=DIRECTION('ref_axis',(1.,6.96054931715756E-14,-2.76820162751213E-15));
#48134=DIRECTION('',(6.76186946307289E-14,-1.,8.61946552381525E-15));
#48135=DIRECTION('center_axis',(2.76820162751153E-15,8.61946552381544E-15,
1.));
#48136=DIRECTION('ref_axis',(-6.76186946307289E-14,1.,-8.61946552381525E-15));
#48137=DIRECTION('',(6.76186946307289E-14,-1.,8.61946552381525E-15));
#48138=DIRECTION('center_axis',(-2.76820162751153E-15,-8.61946552381544E-15,
-1.));
#48139=DIRECTION('ref_axis',(1.,5.72122820091843E-14,-2.76820162751202E-15));
#48140=DIRECTION('',(1.,6.76186946307289E-14,-2.76820162751211E-15));
#48141=DIRECTION('',(-6.76186946307289E-14,1.,-8.61946552381525E-15));
#48142=DIRECTION('center_axis',(7.56475761052649E-15,1.3416021506831E-14,
1.));
#48143=DIRECTION('ref_axis',(6.56318960898822E-14,-1.,1.34160215068305E-14));
#48144=DIRECTION('',(-1.,-6.76186946307289E-14,2.76820162751211E-15));
#48145=DIRECTION('center_axis',(3.16808364362118E-15,-7.7277101918449E-15,
-1.));
#48146=DIRECTION('ref_axis',(-0.581108581114974,0.813826036051036,-8.13001234417858E-15));
#48147=DIRECTION('center_axis',(2.99361242701923E-14,-6.76685568622446E-16,
1.));
#48148=DIRECTION('ref_axis',(0.581108581114944,-0.813826036051057,-1.7946843032697E-14));
#48149=DIRECTION('center_axis',(2.76820162751153E-15,8.61946552381544E-15,
1.));
#48150=DIRECTION('ref_axis',(6.57847267468704E-14,-1.,8.61946552381526E-15));
#48151=DIRECTION('',(0.0101417431417703,-0.0142032227503904,-0.999847695156392));
#48152=DIRECTION('center_axis',(2.76820162751153E-15,8.61946552381544E-15,
1.));
#48153=DIRECTION('ref_axis',(-6.39448049203062E-14,1.,-8.61946552381526E-15));
#48154=DIRECTION('center_axis',(2.76820162751153E-15,8.61946552381544E-15,
1.));
#48155=DIRECTION('ref_axis',(-6.39448049203062E-14,1.,-8.61946552381526E-15));
#48156=DIRECTION('center_axis',(-0.500000000000034,0.499999999999961,-0.707106781186551));
#48157=DIRECTION('ref_axis',(5.400078907659E-14,-0.81649658092773,-0.577350269189619));
#48158=DIRECTION('',(0.809436869760785,-0.0204932255811562,-0.586849198327085));
#48159=DIRECTION('',(-0.0204932255813507,0.809436869760778,0.586849198327087));
#48160=DIRECTION('',(0.707106781186508,0.707106781186587,-8.05229666459882E-15));
#48161=DIRECTION('center_axis',(0.499999999999975,0.500000000000019,-0.707106781186552));
#48162=DIRECTION('ref_axis',(5.34456775642777E-14,-0.816496580927735,-0.577350269189613));
#48163=DIRECTION('',(0.809436869760787,0.0204932255812656,0.586849198327078));
#48164=DIRECTION('',(0.707106781186619,-0.707106781186476,4.1374683795877E-15));
#48165=DIRECTION('',(-0.020493225581152,-0.809436869760773,-0.586849198327101));
#48166=DIRECTION('center_axis',(-0.499999999999967,-0.500000000000045,-0.707106781186539));
#48167=DIRECTION('ref_axis',(5.67531437763696E-14,-0.816496580927717,0.577350269189638));
#48168=DIRECTION('',(0.020493225581241,0.809436869760761,-0.586849198327114));
#48169=DIRECTION('',(-0.809436869760783,-0.0204932255812548,0.586849198327084));
#48170=DIRECTION('',(-0.707106781186604,0.707106781186491,-4.13746837958787E-15));
#48171=DIRECTION('center_axis',(0.500000000000041,-0.499999999999962,-0.707106781186545));
#48172=DIRECTION('ref_axis',(5.68364105032171E-14,-0.816496580927727,0.577350269189624));
#48173=DIRECTION('',(-0.809436869760727,0.0204932255811478,-0.586849198327164));
#48174=DIRECTION('',(0.0204932255812648,-0.809436869760761,0.586849198327114));
#48175=DIRECTION('',(-0.707106781186518,-0.707106781186577,8.05229666459876E-15));
#48176=DIRECTION('center_axis',(0.999390827019098,6.78783181575812E-14,
0.0348994967024421));
#48177=DIRECTION('ref_axis',(-6.76186946307289E-14,1.,-8.61946552381525E-15));
#48178=DIRECTION('',(6.76186946307289E-14,-1.,8.61946552381525E-15));
#48179=DIRECTION('',(6.76186946307289E-14,-1.,8.61946552381525E-15));
#48180=DIRECTION('',(-0.034899496702468,6.254356368018E-15,0.999390827019097));
#48181=DIRECTION('',(0.0348994967024809,-8.11584534007077E-15,-0.999390827019096));
#48182=DIRECTION('',(6.76186946307289E-14,-1.,8.61946552381525E-15));
#48183=DIRECTION('',(-0.0348994967024809,6.25435636801712E-15,0.999390827019096));
#48184=DIRECTION('',(-0.034899496702468,6.254356368018E-15,0.999390827019097));
#48185=DIRECTION('center_axis',(1.10105900386719E-14,4.42832088979503E-14,
1.));
#48186=DIRECTION('ref_axis',(-0.144919489023215,0.98944345048176,-4.22200819281441E-14));
#48187=DIRECTION('',(4.06656903582202E-16,0.0348994967025038,0.999390827019096));
#48188=DIRECTION('center_axis',(7.56475761052712E-15,3.82290954080049E-15,
1.));
#48189=DIRECTION('ref_axis',(-1.,-6.66252953603055E-14,7.56475761052737E-15));
#48190=DIRECTION('center_axis',(6.7674111992527E-14,-0.999390827019096,
0.0348994967025072));
#48191=DIRECTION('ref_axis',(4.06656903581971E-16,0.0348994967025072,0.999390827019096));
#48192=DIRECTION('',(-1.,-6.76186946307289E-14,2.76820162751211E-15));
#48193=DIRECTION('',(-1.,-6.76186946307289E-14,2.76820162751211E-15));
#48194=DIRECTION('',(-4.06656903581526E-16,-0.0348994967025138,-0.999390827019095));
#48195=DIRECTION('',(-1.,-6.76186946307289E-14,2.76820162751211E-15));
#48196=DIRECTION('',(4.06656903581526E-16,0.0348994967025138,0.999390827019095));
#48197=DIRECTION('',(4.06656903581634E-16,0.0348994967025122,0.999390827019095));
#48198=DIRECTION('center_axis',(3.34855224867282E-15,8.43325952165753E-15,
1.));
#48199=DIRECTION('ref_axis',(0.989443450481758,0.144919489023225,-4.53534675172414E-15));
#48200=DIRECTION('',(0.0348994967024996,1.09740731886008E-14,0.999390827019096));
#48201=DIRECTION('center_axis',(-2.02835435550348E-15,3.82290954079984E-15,
1.));
#48202=DIRECTION('ref_axis',(-6.16582990081887E-14,1.,-3.82290954079997E-15));
#48203=DIRECTION('center_axis',(-0.999390827019096,-6.72766881403301E-14,
0.0348994967025019));
#48204=DIRECTION('ref_axis',(6.76186946307289E-14,-1.,8.61946552381525E-15));
#48205=DIRECTION('',(-6.76186946307289E-14,1.,-8.61946552381525E-15));
#48206=DIRECTION('',(-6.76186946307289E-14,1.,-8.61946552381525E-15));
#48207=DIRECTION('',(-0.0348994967025063,-1.09740731886012E-14,-0.999390827019096));
#48208=DIRECTION('',(-6.76186946307289E-14,1.,-8.61946552381525E-15));
#48209=DIRECTION('',(0.0348994967025063,1.28355621606549E-14,0.999390827019096));
#48210=DIRECTION('',(6.76186946307289E-14,-1.,8.61946552381525E-15));
#48211=DIRECTION('',(0.0348994967025071,1.09740731886013E-14,0.999390827019096));
#48212=DIRECTION('center_axis',(4.9279827061289E-15,1.80927121643866E-14,
1.));
#48213=DIRECTION('ref_axis',(0.144919489023234,-0.989443450481757,1.71875548168164E-14));
#48214=DIRECTION('center_axis',(2.25645886980557E-15,-1.36441260211317E-14,
-1.));
#48215=DIRECTION('ref_axis',(7.80251072522735E-14,-1.,1.36441260211319E-14));
#48216=DIRECTION('',(5.12637372416654E-15,-0.034899496702487,0.999390827019096));
#48217=DIRECTION('center_axis',(7.56475761052717E-15,3.82290954080049E-15,
1.));
#48218=DIRECTION('ref_axis',(1.,7.34549153444662E-14,-7.56475761052745E-15));
#48219=DIRECTION('center_axis',(-6.74808943053846E-14,0.999390827019096,
0.0348994967024958));
#48220=DIRECTION('ref_axis',(-5.12637372416713E-15,0.0348994967024958,-0.999390827019096));
#48221=DIRECTION('',(1.,6.76186946307289E-14,-2.76820162751211E-15));
#48222=DIRECTION('center_axis',(3.48068716811668E-13,-0.999390827019095,
-0.0348994967025218));
#48223=DIRECTION('ref_axis',(-0.995316427483098,-0.00337375605847328,0.0966117329952275));
#48224=DIRECTION('',(-1.,-6.76186946307289E-14,2.76820162751211E-15));
#48225=DIRECTION('center_axis',(-2.01883415239548E-13,-0.999390827019095,
-0.0348994967025223));
#48226=DIRECTION('ref_axis',(0.995051211981761,-0.00346773269898284,0.0993028718797044));
#48227=DIRECTION('',(1.,6.76186946307289E-14,-2.76820162751211E-15));
#48228=DIRECTION('',(-1.,-6.76186946307289E-14,2.76820162751211E-15));
#48229=DIRECTION('',(-5.1263737241671E-15,0.0348994967024954,-0.999390827019096));
#48230=DIRECTION('',(1.,6.76186946307289E-14,-2.76820162751211E-15));
#48231=DIRECTION('',(5.1263737241671E-15,-0.0348994967024954,0.999390827019096));
#48232=DIRECTION('',(5.12637372416711E-15,-0.0348994967024956,0.999390827019096));
#48233=DIRECTION('center_axis',(3.8368846416151E-14,-1.48709733737763E-16,
1.));
#48234=DIRECTION('ref_axis',(-0.989443450481756,-0.144919489023242,3.7942252850375E-14));
#48235=DIRECTION('center_axis',(-2.02835435550344E-15,3.82290954079982E-15,
1.));
#48236=DIRECTION('ref_axis',(6.16582990081887E-14,-1.,3.82290954079995E-15));
#48237=DIRECTION('center_axis',(2.76820162751153E-15,8.61946552381544E-15,
1.));
#48238=DIRECTION('ref_axis',(-6.76186946307289E-14,1.,-8.61946552381525E-15));
#48239=DIRECTION('',(6.76186946307289E-14,-1.,8.61946552381525E-15));
#48240=DIRECTION('',(6.76186946307289E-14,-1.,8.61946552381525E-15));
#48241=DIRECTION('center_axis',(7.56475761052712E-15,3.8229095408005E-15,
1.));
#48242=DIRECTION('ref_axis',(-1.,-6.87362688099551E-14,7.56475761052739E-15));
#48243=DIRECTION('',(1.,6.76186946307289E-14,-2.76820162751211E-15));
#48244=DIRECTION('',(1.,6.76186946307289E-14,-2.76820162751211E-15));
#48245=DIRECTION('center_axis',(-2.02835435550342E-15,3.82290954079985E-15,
1.));
#48246=DIRECTION('ref_axis',(6.76186946307289E-14,-1.,3.82290954079999E-15));
#48247=DIRECTION('',(-6.76186946307289E-14,1.,-8.61946552381525E-15));
#48248=DIRECTION('',(-6.76186946307289E-14,1.,-8.61946552381525E-15));
#48249=DIRECTION('center_axis',(2.76820162751153E-15,8.61946552381544E-15,
1.));
#48250=DIRECTION('ref_axis',(1.,6.76186946307289E-14,-2.76820162751211E-15));
#48251=DIRECTION('',(-1.,-6.76186946307289E-14,2.76820162751211E-15));
#48252=DIRECTION('',(-1.,-6.76186946307289E-14,2.76820162751211E-15));
#48253=DIRECTION('center_axis',(-2.02835435550342E-15,3.82290954079985E-15,
1.));
#48254=DIRECTION('ref_axis',(-6.56318960898822E-14,1.,-3.82290954079999E-15));
#48255=DIRECTION('center_axis',(-1.,-6.76186946307289E-14,2.76820162751211E-15));
#48256=DIRECTION('ref_axis',(6.76186946307289E-14,-1.,8.61946552381525E-15));
#48257=DIRECTION('',(-6.76186946307289E-14,1.,-8.61946552381525E-15));
#48258=DIRECTION('',(-2.76820162751153E-15,-8.61946552381544E-15,-1.));
#48259=DIRECTION('center_axis',(4.40730523866621E-15,1.04820891558594E-14,
1.));
#48260=DIRECTION('ref_axis',(-6.56318960898822E-14,1.,-1.04820891558591E-14));
#48261=DIRECTION('center_axis',(7.56475761052712E-15,3.8229095408005E-15,
1.));
#48262=DIRECTION('ref_axis',(-1.,-6.87362688099551E-14,7.56475761052739E-15));
#48263=DIRECTION('',(-2.76820162751153E-15,-8.61946552381544E-15,-1.));
#48264=DIRECTION('center_axis',(-6.76186946307289E-14,1.,-8.61946552381525E-15));
#48265=DIRECTION('ref_axis',(-2.76820162751153E-15,-8.61946552381544E-15,
-1.));
#48266=DIRECTION('',(1.,6.76186946307289E-14,-2.76820162751211E-15));
#48267=DIRECTION('center_axis',(6.76186946307289E-14,-1.,8.61946552381525E-15));
#48268=DIRECTION('ref_axis',(2.76820162751153E-15,8.61946552381544E-15,
1.));
#48269=DIRECTION('',(-2.76820162751153E-15,-8.61946552381544E-15,-1.));
#48270=DIRECTION('center_axis',(2.76820162751153E-15,8.61946552381544E-15,
1.));
#48271=DIRECTION('ref_axis',(-1.,-6.86120939011522E-14,2.76820162751212E-15));
#48272=DIRECTION('',(-2.76820162751153E-15,-8.61946552381544E-15,-1.));
#48273=DIRECTION('center_axis',(-1.,-6.76186946307289E-14,2.76820162751211E-15));
#48274=DIRECTION('ref_axis',(6.76186946307289E-14,-1.,8.61946552381525E-15));
#48275=DIRECTION('center_axis',(1.,6.76186946307289E-14,-2.76820162751211E-15));
#48276=DIRECTION('ref_axis',(-6.76186946307289E-14,1.,-8.61946552381525E-15));
#48277=DIRECTION('',(-2.76820162751153E-15,-8.61946552381544E-15,-1.));
#48278=DIRECTION('center_axis',(2.76820162751153E-15,8.61946552381544E-15,
1.));
#48279=DIRECTION('ref_axis',(6.76186946307289E-14,-1.,8.61946552381525E-15));
#48280=DIRECTION('',(-2.76820162751153E-15,-8.61946552381544E-15,-1.));
#48281=DIRECTION('center_axis',(6.76186946307289E-14,-1.,8.61946552381525E-15));
#48282=DIRECTION('ref_axis',(2.76820162751153E-15,8.61946552381544E-15,
1.));
#48283=DIRECTION('center_axis',(-6.65967751777163E-14,1.,-8.61946552381525E-15));
#48284=DIRECTION('ref_axis',(-2.76820162751153E-15,-8.61946552381544E-15,
-1.));
#48285=DIRECTION('',(-2.76820162751153E-15,-8.61946552381544E-15,-1.));
#48286=DIRECTION('center_axis',(2.76820162751152E-15,8.84298554470447E-15,
1.));
#48287=DIRECTION('ref_axis',(1.,6.83637440835464E-14,-2.76820162751212E-15));
#48288=DIRECTION('',(-2.76820162751153E-15,-8.61946552381544E-15,-1.));
#48289=DIRECTION('center_axis',(1.,6.76186946307289E-14,-2.76820162751211E-15));
#48290=DIRECTION('ref_axis',(-6.76186946307289E-14,1.,-8.61946552381525E-15));
#48291=DIRECTION('center_axis',(2.76820162751153E-15,8.61946552381544E-15,
1.));
#48292=DIRECTION('ref_axis',(-6.76186946307289E-14,1.,-8.61946552381525E-15));
#48293=DIRECTION('center_axis',(-2.76820162751153E-15,-8.61946552381544E-15,
-1.));
#48294=DIRECTION('ref_axis',(0.338105122691878,-0.941108349771433,7.17590782412407E-15));
#48295=DIRECTION('center_axis',(2.76820162751206E-15,7.35344329979309E-16,
1.));
#48296=DIRECTION('ref_axis',(0.329874263976713,-0.944024877832053,-2.18975133141472E-16));
#48297=DIRECTION('center_axis',(2.76820162751153E-15,8.61946552381544E-15,
1.));
#48298=DIRECTION('ref_axis',(0.338105122691879,-0.941108349771433,7.17590782412406E-15));
#48299=DIRECTION('center_axis',(2.76820162751153E-15,8.61946552381544E-15,
1.));
#48300=DIRECTION('ref_axis',(-6.76186946307289E-14,1.,-8.61946552381525E-15));
#48301=DIRECTION('center_axis',(-2.76820162751153E-15,-8.61946552381544E-15,
-1.));
#48302=DIRECTION('ref_axis',(6.76186946307289E-14,-1.,8.61946552381525E-15));
#48303=DIRECTION('center_axis',(2.76820162751153E-15,8.61946552381544E-15,
1.));
#48304=DIRECTION('ref_axis',(1.83515276180121E-13,-1.,8.61946552381493E-15));
#48305=DIRECTION('',(2.76820162751153E-15,8.61946552381544E-15,1.));
#48306=DIRECTION('center_axis',(2.76820162751153E-15,8.61946552381544E-15,
1.));
#48307=DIRECTION('ref_axis',(1.17288658151894E-13,-1.,8.61946552381511E-15));
#48308=DIRECTION('',(2.76820162751153E-15,8.61946552381544E-15,1.));
#48309=DIRECTION('center_axis',(-6.76186946307289E-14,1.,-8.61946552381525E-15));
#48310=DIRECTION('ref_axis',(-2.76820162751153E-15,-8.61946552381544E-15,
-1.));
#48311=DIRECTION('',(1.,6.76186946307289E-14,-2.76820162751211E-15));
#48312=DIRECTION('',(2.76820162751153E-15,8.61946552381544E-15,1.));
#48313=DIRECTION('',(1.,6.76186946307289E-14,-2.76820162751211E-15));
#48314=DIRECTION('center_axis',(-2.76820162751153E-15,-8.61946552381544E-15,
-1.));
#48315=DIRECTION('ref_axis',(0.981901184295549,-0.189393939393524,-1.08562592540037E-15));
#48316=DIRECTION('center_axis',(-2.02627523364964E-14,3.65172596209946E-14,
1.));
#48317=DIRECTION('ref_axis',(0.981901184295513,-0.189393939393713,2.68121681717756E-14));
#48318=DIRECTION('',(2.76820162751153E-15,8.61946552381544E-15,1.));
#48319=DIRECTION('center_axis',(-2.02627523364964E-14,3.65172596209946E-14,
1.));
#48320=DIRECTION('ref_axis',(0.981901184295513,-0.189393939393713,2.68121681717756E-14));
#48321=DIRECTION('center_axis',(-2.76820162751153E-15,-8.61946552381544E-15,
-1.));
#48322=DIRECTION('ref_axis',(-0.981901184295477,0.1893939393939,1.08562592539693E-15));
#48323=DIRECTION('center_axis',(2.76820162751153E-15,8.61946552381544E-15,
1.));
#48324=DIRECTION('ref_axis',(-0.981901184295475,0.189393939393907,1.08562592539687E-15));
#48325=DIRECTION('',(2.76820162751153E-15,8.61946552381544E-15,1.));
#48326=DIRECTION('center_axis',(-1.51165366653243E-14,1.60275666842004E-14,
1.));
#48327=DIRECTION('ref_axis',(-0.981901184295476,0.189393939393906,-1.78784692473471E-14));
#48328=DIRECTION('center_axis',(-2.76820162751153E-15,-8.61946552381544E-15,
-1.));
#48329=DIRECTION('ref_axis',(0.707106781186593,0.707106781186502,-8.05229666459833E-15));
#48330=DIRECTION('center_axis',(3.87802647389425E-14,1.20608411849333E-14,
1.));
#48331=DIRECTION('ref_axis',(0.707106781186678,0.707106781186417,-3.59500907617996E-14));
#48332=DIRECTION('',(2.76820162751153E-15,8.61946552381544E-15,1.));
#48333=DIRECTION('center_axis',(2.76820162751153E-15,8.61946552381544E-15,
1.));
#48334=DIRECTION('ref_axis',(0.707106781186678,0.707106781186417,-8.05229666459783E-15));
#48335=DIRECTION('center_axis',(-0.707106781186549,-0.707106781186546,8.05229666459858E-15));
#48336=DIRECTION('ref_axis',(2.76820162751153E-15,8.61946552381544E-15,
1.));
#48337=DIRECTION('',(-0.707106781186631,0.707106781186464,-4.13746837958756E-15));
#48338=DIRECTION('',(2.76820162751153E-15,8.61946552381544E-15,1.));
#48339=DIRECTION('',(-0.707106781186631,0.707106781186464,-4.13746837958756E-15));
#48340=DIRECTION('center_axis',(-2.76820162751153E-15,-8.61946552381544E-15,
-1.));
#48341=DIRECTION('ref_axis',(-0.815724561786088,0.578440523562185,-2.72775809088462E-15));
#48342=DIRECTION('center_axis',(2.76820162751153E-15,8.61946552381544E-15,
1.));
#48343=DIRECTION('ref_axis',(-0.815724561786174,0.578440523562064,-2.72775809088334E-15));
#48344=DIRECTION('',(2.76820162751153E-15,8.61946552381544E-15,1.));
#48345=DIRECTION('center_axis',(2.76820162751153E-15,8.61946552381544E-15,
1.));
#48346=DIRECTION('ref_axis',(-0.815724561786174,0.578440523562064,-2.72775809088334E-15));
#48347=DIRECTION('center_axis',(-2.76820162751153E-15,-8.61946552381544E-15,
-1.));
#48348=DIRECTION('ref_axis',(-0.985823571918317,0.167785234899295,1.28273936860376E-15));
#48349=DIRECTION('center_axis',(1.4606207662274E-14,3.71600285032521E-15,
1.));
#48350=DIRECTION('ref_axis',(-0.985823571918316,0.167785234899296,1.37756533986753E-14));
#48351=DIRECTION('center_axis',(2.76820162751153E-15,8.61946552381544E-15,
1.));
#48352=DIRECTION('ref_axis',(-0.985823571918316,0.167785234899296,1.28273936860375E-15));
#48353=DIRECTION('center_axis',(2.76820162751153E-15,8.61946552381544E-15,
1.));
#48354=DIRECTION('ref_axis',(-6.76186946307289E-14,1.,-8.61946552381525E-15));
#48355=DIRECTION('center_axis',(0.70710678118645,0.707106781186645,-8.05229666459916E-15));
#48356=DIRECTION('ref_axis',(-2.76820162751153E-15,-8.61946552381544E-15,
-1.));
#48357=DIRECTION('',(0.707106781186554,-0.707106781186541,4.13746837958844E-15));
#48358=DIRECTION('',(2.76820162751153E-15,8.61946552381544E-15,1.));
#48359=DIRECTION('',(0.707106781186554,-0.707106781186541,4.13746837958844E-15));
#48360=DIRECTION('',(2.76820162751153E-15,8.61946552381544E-15,1.));
#48361=DIRECTION('center_axis',(-2.76820162751153E-15,-8.61946552381544E-15,
-1.));
#48362=DIRECTION('ref_axis',(0.560387247009387,-0.828230724731485,5.58764128837962E-15));
#48363=DIRECTION('center_axis',(-6.73174033601705E-16,-2.73925975876096E-14,
1.));
#48364=DIRECTION('ref_axis',(0.560387247009324,-0.828230724731527,-2.23101528088168E-14));
#48365=DIRECTION('',(2.76820162751153E-15,8.61946552381544E-15,1.));
#48366=DIRECTION('center_axis',(2.76820162751153E-15,8.61946552381544E-15,
1.));
#48367=DIRECTION('ref_axis',(0.560387247009278,-0.828230724731558,5.58764128838055E-15));
#48368=DIRECTION('center_axis',(-2.76820162751153E-15,-8.61946552381544E-15,
-1.));
#48369=DIRECTION('ref_axis',(-0.560387247009416,0.828230724731465,-5.58764128837936E-15));
#48370=DIRECTION('center_axis',(-3.46342042556553E-15,2.43000874453061E-14,
1.));
#48371=DIRECTION('ref_axis',(-0.560387247009403,0.828230724731474,-2.20669356733829E-14));
#48372=DIRECTION('',(2.76820162751153E-15,8.61946552381544E-15,1.));
#48373=DIRECTION('center_axis',(2.76820162751153E-15,8.61946552381544E-15,
1.));
#48374=DIRECTION('ref_axis',(-0.560387247009409,0.82823072473147,-5.58764128837942E-15));
#48375=DIRECTION('center_axis',(-2.76820162751153E-15,-8.61946552381544E-15,
-1.));
#48376=DIRECTION('ref_axis',(1.,6.76186946307289E-14,-2.76820162751211E-15));
#48377=DIRECTION('center_axis',(-2.37218282461811E-14,3.11387233849611E-14,
1.));
#48378=DIRECTION('ref_axis',(1.,3.86445492433809E-14,2.37218282461799E-14));
#48379=DIRECTION('',(2.76820162751153E-15,8.61946552381544E-15,1.));
#48380=DIRECTION('center_axis',(-2.37218282461811E-14,3.11387233849611E-14,
1.));
#48381=DIRECTION('ref_axis',(1.,3.86445492433809E-14,2.37218282461799E-14));
#48382=DIRECTION('center_axis',(-1.,-6.76186946307289E-14,2.76820162751211E-15));
#48383=DIRECTION('ref_axis',(6.76186946307289E-14,-1.,8.61946552381525E-15));
#48384=DIRECTION('',(-6.76186946307289E-14,1.,-8.61946552381525E-15));
#48385=DIRECTION('',(2.76820162751153E-15,8.61946552381544E-15,1.));
#48386=DIRECTION('',(-6.76186946307289E-14,1.,-8.61946552381525E-15));
#48387=DIRECTION('center_axis',(-2.76820162751153E-15,-8.61946552381544E-15,
-1.));
#48388=DIRECTION('ref_axis',(-0.14261736693024,0.989777897636579,-8.13656283766531E-15));
#48389=DIRECTION('center_axis',(-1.293091612144E-14,-9.50387773154572E-15,
1.));
#48390=DIRECTION('ref_axis',(-0.142617366930127,0.989777897636595,7.56255491129047E-15));
#48391=DIRECTION('',(2.76820162751153E-15,8.61946552381544E-15,1.));
#48392=DIRECTION('center_axis',(-1.293091612144E-14,-9.50387773154572E-15,
1.));
#48393=DIRECTION('ref_axis',(-0.142617366930127,0.989777897636595,7.56255491129047E-15));
#48394=DIRECTION('center_axis',(-2.76820162751153E-15,-8.61946552381544E-15,
-1.));
#48395=DIRECTION('ref_axis',(-0.578440455376734,0.815724610137243,-5.42987034401337E-15));
#48396=DIRECTION('center_axis',(2.76820162751153E-15,8.61946552381544E-15,
1.));
#48397=DIRECTION('ref_axis',(-0.578440455376735,0.815724610137242,-5.42987034401336E-15));
#48398=DIRECTION('',(2.76820162751153E-15,8.61946552381544E-15,1.));
#48399=DIRECTION('center_axis',(2.76820162751153E-15,8.61946552381544E-15,
1.));
#48400=DIRECTION('ref_axis',(-0.578440455376735,0.815724610137242,-5.42987034401336E-15));
#48401=DIRECTION('center_axis',(-2.76820162751153E-15,-8.61946552381544E-15,
-1.));
#48402=DIRECTION('ref_axis',(-0.707106781186599,-0.707106781186496,8.05229666459829E-15));
#48403=DIRECTION('center_axis',(2.76820162751153E-15,8.61946552381544E-15,
1.));
#48404=DIRECTION('ref_axis',(-0.707106781186148,-0.707106781186947,8.05229666460093E-15));
#48405=DIRECTION('center_axis',(2.76820162751153E-15,8.61946552381544E-15,
1.));
#48406=DIRECTION('ref_axis',(-0.707106781186148,-0.707106781186947,8.05229666460093E-15));
#48407=DIRECTION('center_axis',(2.76820162751153E-15,8.61946552381544E-15,
1.));
#48408=DIRECTION('ref_axis',(-6.76186946307289E-14,1.,-8.61946552381525E-15));
#48409=DIRECTION('center_axis',(-2.76820162751153E-15,-8.61946552381544E-15,
-1.));
#48410=DIRECTION('ref_axis',(-0.815724610137212,-0.578440455376777,7.24393775608327E-15));
#48411=DIRECTION('center_axis',(-9.06980458537594E-15,3.71600279897938E-15,
1.));
#48412=DIRECTION('ref_axis',(-0.815724610137216,-0.578440455376772,-5.24897645820353E-15));
#48413=DIRECTION('',(2.76820162751153E-15,8.61946552381544E-15,1.));
#48414=DIRECTION('center_axis',(-9.06980458537584E-15,3.7160027989794E-15,
1.));
#48415=DIRECTION('ref_axis',(-0.815724610137217,-0.578440455376771,-5.24897645820345E-15));
#48416=DIRECTION('',(2.76820162751153E-15,8.61946552381544E-15,1.));
#48417=DIRECTION('center_axis',(-2.76820162751153E-15,-8.61946552381544E-15,
-1.));
#48418=DIRECTION('ref_axis',(0.707106781186686,-0.707106781186409,4.13746837958694E-15));
#48419=DIRECTION('center_axis',(8.04566559262691E-16,-1.46211539950285E-14,
1.));
#48420=DIRECTION('ref_axis',(0.707106781186663,-0.707106781186432,-1.09076316086264E-14));
#48421=DIRECTION('',(2.76820162751153E-15,8.61946552381544E-15,1.));
#48422=DIRECTION('center_axis',(4.73183669576037E-15,3.18600850426594E-14,
1.));
#48423=DIRECTION('ref_axis',(0.707106781186663,-0.707106781186432,1.91825683678008E-14));
#48424=DIRECTION('center_axis',(-0.707106781186641,0.707106781186454,-4.13746837958745E-15));
#48425=DIRECTION('ref_axis',(-2.76820162751153E-15,-8.61946552381544E-15,
-1.));
#48426=DIRECTION('',(0.707106781186536,0.707106781186559,-8.05229666459866E-15));
#48427=DIRECTION('',(2.76820162751153E-15,8.61946552381544E-15,1.));
#48428=DIRECTION('',(0.707106781186536,0.707106781186559,-8.05229666459866E-15));
#48429=DIRECTION('center_axis',(-2.76820162751153E-15,-8.61946552381544E-15,
-1.));
#48430=DIRECTION('ref_axis',(0.82823072473152,0.560387247009334,-7.12294819573965E-15));
#48431=DIRECTION('center_axis',(3.87802647389429E-14,5.17808986270238E-15,
1.));
#48432=DIRECTION('ref_axis',(0.828230724731499,0.560387247009366,-3.50207422929409E-14));
#48433=DIRECTION('',(2.76820162751153E-15,8.61946552381544E-15,1.));
#48434=DIRECTION('center_axis',(7.47923278503742E-14,1.73671420158932E-15,
1.));
#48435=DIRECTION('ref_axis',(0.828230724731499,0.560387247009366,-6.2918536390142E-14));
#48436=DIRECTION('center_axis',(-2.76820162751153E-15,-8.61946552381544E-15,
-1.));
#48437=DIRECTION('ref_axis',(-0.828230724731476,-0.560387247009399,7.12294819574009E-15));
#48438=DIRECTION('center_axis',(2.76820162751153E-15,8.61946552381544E-15,
1.));
#48439=DIRECTION('ref_axis',(-0.828230724731477,-0.560387247009398,7.12294819574008E-15));
#48440=DIRECTION('',(2.76820162751153E-15,8.61946552381544E-15,1.));
#48441=DIRECTION('center_axis',(2.06529399203462E-14,1.60275666842028E-14,
1.));
#48442=DIRECTION('ref_axis',(-0.828230724731477,-0.560387247009398,2.6087043368484E-14));
#48443=DIRECTION('center_axis',(-2.76820162751153E-15,-8.61946552381544E-15,
-1.));
#48444=DIRECTION('ref_axis',(-6.76186946307289E-14,1.,-8.61946552381525E-15));
#48445=DIRECTION('center_axis',(2.57991555915155E-14,3.6517259620996E-14,
1.));
#48446=DIRECTION('ref_axis',(-3.32525166743677E-13,1.,-3.65172596209874E-14));
#48447=DIRECTION('',(2.76820162751153E-15,8.61946552381544E-15,1.));
#48448=DIRECTION('center_axis',(2.76820162751153E-15,8.61946552381544E-15,
1.));
#48449=DIRECTION('ref_axis',(-3.32525166743677E-13,1.,-8.61946552381452E-15));
#48450=DIRECTION('center_axis',(6.76186946307289E-14,-1.,8.61946552381525E-15));
#48451=DIRECTION('ref_axis',(2.76820162751153E-15,8.61946552381544E-15,
1.));
#48452=DIRECTION('',(-1.,-6.76186946307289E-14,2.76820162751211E-15));
#48453=DIRECTION('',(2.76820162751153E-15,8.61946552381544E-15,1.));
#48454=DIRECTION('',(-1.,-6.76186946307289E-14,2.76820162751211E-15));
#48455=DIRECTION('center_axis',(-2.76820162751153E-15,-8.61946552381544E-15,
-1.));
#48456=DIRECTION('ref_axis',(-0.985823571918217,-0.167785234899881,4.17517746384804E-15));
#48457=DIRECTION('center_axis',(2.0590300960797E-14,-6.42563446439966E-15,
1.));
#48458=DIRECTION('ref_axis',(-0.98582357191831,-0.167785234899333,1.92202774520594E-14));
#48459=DIRECTION('center_axis',(2.76820162751153E-15,8.61946552381544E-15,
1.));
#48460=DIRECTION('ref_axis',(-0.985823571918306,-0.167785234899355,4.17517746384375E-15));
#48461=DIRECTION('center_axis',(2.76820162751153E-15,8.61946552381544E-15,
1.));
#48462=DIRECTION('ref_axis',(-6.76186946307289E-14,1.,-8.61946552381525E-15));
#48463=DIRECTION('center_axis',(-2.76820162751153E-15,-8.61946552381544E-15,
-1.));
#48464=DIRECTION('ref_axis',(-0.142617449664351,-0.989777885715394,8.92615021843118E-15));
#48465=DIRECTION('center_axis',(7.02512529519804E-15,1.92786459487573E-14,
1.));
#48466=DIRECTION('ref_axis',(-0.142617449664345,-0.989777885715395,2.00834828797903E-14));
#48467=DIRECTION('',(2.76820162751153E-15,8.61946552381544E-15,1.));
#48468=DIRECTION('center_axis',(7.02512529519795E-15,1.92786459487572E-14,
1.));
#48469=DIRECTION('ref_axis',(-0.142617449664338,-0.989777885715396,2.00834828797902E-14));
#48470=DIRECTION('',(2.76820162751153E-15,8.61946552381544E-15,1.));
#48471=DIRECTION('center_axis',(-2.76820162751153E-15,-8.61946552381544E-15,
-1.));
#48472=DIRECTION('ref_axis',(1.,4.27837128701397E-14,-2.7682016275119E-15));
#48473=DIRECTION('center_axis',(2.76820162751153E-15,8.61946552381544E-15,
1.));
#48474=DIRECTION('ref_axis',(1.,-1.04156595879955E-13,-2.76820162751063E-15));
#48475=DIRECTION('',(2.76820162751153E-15,8.61946552381544E-15,1.));
#48476=DIRECTION('center_axis',(2.76820162751153E-15,8.61946552381544E-15,
1.));
#48477=DIRECTION('ref_axis',(1.,-1.04156595879955E-13,-2.76820162751063E-15));
#48478=DIRECTION('center_axis',(-1.,-6.76186946307289E-14,2.76820162751211E-15));
#48479=DIRECTION('ref_axis',(6.76186946307289E-14,-1.,8.61946552381525E-15));
#48480=DIRECTION('',(-6.76186946307289E-14,1.,-8.61946552381525E-15));
#48481=DIRECTION('',(2.76820162751153E-15,8.61946552381544E-15,1.));
#48482=DIRECTION('',(-6.76186946307289E-14,1.,-8.61946552381525E-15));
#48483=DIRECTION('center_axis',(-2.76820162751153E-15,-8.61946552381544E-15,
-1.));
#48484=DIRECTION('ref_axis',(0.160984739080998,0.986956895605387,-8.95267915189108E-15));
#48485=DIRECTION('center_axis',(2.76820162751153E-15,8.61946552381544E-15,
1.));
#48486=DIRECTION('ref_axis',(0.160984739081009,0.986956895605385,-8.9526791518911E-15));
#48487=DIRECTION('',(2.76820162751153E-15,8.61946552381544E-15,1.));
#48488=DIRECTION('center_axis',(2.76820162751153E-15,8.61946552381544E-15,
1.));
#48489=DIRECTION('ref_axis',(0.160984739080975,0.986956895605391,-8.95267915189105E-15));
#48490=DIRECTION('center_axis',(-2.76820162751153E-15,-8.61946552381544E-15,
-1.));
#48491=DIRECTION('ref_axis',(-0.160984853694478,-0.98695687691052,8.95267930802455E-15));
#48492=DIRECTION('center_axis',(2.76820162751153E-15,8.61946552381544E-15,
1.));
#48493=DIRECTION('ref_axis',(-0.160984853694478,-0.98695687691052,8.95267930802455E-15));
#48494=DIRECTION('',(2.76820162751153E-15,8.61946552381544E-15,1.));
#48495=DIRECTION('center_axis',(2.76820162751153E-15,8.61946552381544E-15,
1.));
#48496=DIRECTION('ref_axis',(-0.16098485369447,-0.986956876910521,8.95267930802453E-15));
#48497=DIRECTION('center_axis',(-2.76820162751153E-15,-8.61946552381544E-15,
-1.));
#48498=DIRECTION('ref_axis',(-0.707106781186625,0.70710678118647,-4.13746837958763E-15));
#48499=DIRECTION('center_axis',(2.76820162751153E-15,8.61946552381544E-15,
1.));
#48500=DIRECTION('ref_axis',(-0.707106781186618,0.707106781186477,-4.13746837958771E-15));
#48501=DIRECTION('',(2.76820162751153E-15,8.61946552381544E-15,1.));
#48502=DIRECTION('center_axis',(-6.73183838288935E-16,4.46315494435653E-14,
1.));
#48503=DIRECTION('ref_axis',(-0.707106781186618,0.707106781186477,-3.20352841234439E-14));
#48504=DIRECTION('center_axis',(0.707106781186635,-0.70710678118646,4.13746837958752E-15));
#48505=DIRECTION('ref_axis',(2.76820162751153E-15,8.61946552381544E-15,
1.));
#48506=DIRECTION('',(-0.707106781186539,-0.707106781186556,8.05229666459864E-15));
#48507=DIRECTION('',(2.76820162751153E-15,8.61946552381544E-15,1.));
#48508=DIRECTION('',(-0.707106781186539,-0.707106781186556,8.05229666459864E-15));
#48509=DIRECTION('center_axis',(-2.76820162751153E-15,-8.61946552381544E-15,
-1.));
#48510=DIRECTION('ref_axis',(-0.578440455376605,-0.815724610137334,8.63234996399857E-15));
#48511=DIRECTION('center_axis',(2.76820162751153E-15,8.61946552381544E-15,
1.));
#48512=DIRECTION('ref_axis',(-0.57844045537632,-0.815724610137536,8.63234996399952E-15));
#48513=DIRECTION('center_axis',(2.76820162751153E-15,8.61946552381544E-15,
1.));
#48514=DIRECTION('ref_axis',(-0.57844045537632,-0.815724610137536,8.63234996399952E-15));
#48515=DIRECTION('center_axis',(2.76820162751153E-15,8.61946552381544E-15,
1.));
#48516=DIRECTION('ref_axis',(-6.76186946307289E-14,1.,-8.61946552381525E-15));
#48517=DIRECTION('center_axis',(-2.76820162751153E-15,-8.61946552381544E-15,
-1.));
#48518=DIRECTION('ref_axis',(0.160984848484789,0.986956877760285,-8.95267930092759E-15));
#48519=DIRECTION('center_axis',(2.76820162751153E-15,8.61946552381544E-15,
1.));
#48520=DIRECTION('ref_axis',(0.160984848484786,0.986956877760285,-8.95267930092759E-15));
#48521=DIRECTION('',(2.76820162751153E-15,8.61946552381544E-15,1.));
#48522=DIRECTION('',(2.76820162751153E-15,8.61946552381544E-15,1.));
#48523=DIRECTION('center_axis',(-2.76820162751153E-15,-8.61946552381544E-15,
-1.));
#48524=DIRECTION('ref_axis',(-0.160984848484817,-0.98695687776028,8.95267930092763E-15));
#48525=DIRECTION('center_axis',(2.76820162751153E-15,8.61946552381544E-15,
1.));
#48526=DIRECTION('ref_axis',(-0.160984848484789,-0.986956877760285,8.95267930092759E-15));
#48527=DIRECTION('',(2.76820162751153E-15,8.61946552381544E-15,1.));
#48528=DIRECTION('center_axis',(1.,6.76186946307289E-14,-2.76820162751211E-15));
#48529=DIRECTION('ref_axis',(-6.76186946307289E-14,1.,-8.61946552381525E-15));
#48530=DIRECTION('',(6.76186946307289E-14,-1.,8.61946552381525E-15));
#48531=DIRECTION('',(2.76820162751153E-15,8.61946552381544E-15,1.));
#48532=DIRECTION('center_axis',(-2.76820162751153E-15,-8.61946552381544E-15,
-1.));
#48533=DIRECTION('ref_axis',(-1.,-5.93403673771998E-14,2.76820162751204E-15));
#48534=DIRECTION('center_axis',(-1.29309139275491E-14,2.67428077770537E-14,
1.));
#48535=DIRECTION('ref_axis',(-1.,3.5860396038368E-14,-1.29309139275501E-14));
#48536=DIRECTION('',(2.76820162751153E-15,8.61946552381544E-15,1.));
#48537=DIRECTION('center_axis',(-2.76820162751153E-15,-8.61946552381544E-15,
-1.));
#48538=DIRECTION('ref_axis',(0.142617449664357,0.989777885715393,-8.92615021843119E-15));
#48539=DIRECTION('center_axis',(7.02512538336182E-15,1.92786462781398E-14,
1.));
#48540=DIRECTION('ref_axis',(0.142617449664349,0.989777885715395,-2.00834832183795E-14));
#48541=DIRECTION('',(2.76820162751153E-15,8.61946552381544E-15,1.));
#48542=DIRECTION('center_axis',(-2.76820162751153E-15,-8.61946552381544E-15,
-1.));
#48543=DIRECTION('ref_axis',(0.578440307445746,0.815724715036924,-8.63235045867452E-15));
#48544=DIRECTION('center_axis',(-2.04724131764889E-14,6.65582873155238E-15,
1.));
#48545=DIRECTION('ref_axis',(0.578440307445796,0.815724715036889,6.41274497658572E-15));
#48546=DIRECTION('',(2.76820162751153E-15,8.61946552381544E-15,1.));
#48547=DIRECTION('center_axis',(-2.76820162751153E-15,-8.61946552381544E-15,
-1.));
#48548=DIRECTION('ref_axis',(0.7071067811866,-0.707106781186495,4.13746837958792E-15));
#48549=DIRECTION('center_axis',(-6.73174033609845E-16,4.46315286352391E-14,
1.));
#48550=DIRECTION('ref_axis',(0.7071067811866,-0.707106781186495,3.20352624767811E-14));
#48551=DIRECTION('',(2.76820162751153E-15,8.61946552381544E-15,1.));
#48552=DIRECTION('center_axis',(-0.707106781186595,0.7071067811865,-4.13746837958797E-15));
#48553=DIRECTION('ref_axis',(-2.76820162751153E-15,-8.61946552381544E-15,
-1.));
#48554=DIRECTION('',(0.7071067811865,0.707106781186595,-8.05229666459887E-15));
#48555=DIRECTION('center_axis',(3.77043884608029E-15,9.11212513897563E-15,
1.));
#48556=DIRECTION('ref_axis',(-6.75992533669751E-14,1.,-9.79699324159059E-15));
#48557=DIRECTION('center_axis',(1.,6.79666406135347E-14,-3.77043884608091E-15));
#48558=DIRECTION('ref_axis',(6.79666406135348E-14,-1.,8.57236908639177E-15));
#48559=DIRECTION('center_axis',(2.76820162751153E-15,8.61946552381544E-15,
1.));
#48560=DIRECTION('ref_axis',(-6.54074540654431E-14,1.,-8.61946552381526E-15));
#48561=DIRECTION('center_axis',(-2.76820162751153E-15,-8.61946552381544E-15,
-1.));
#48562=DIRECTION('ref_axis',(6.76186946307289E-14,-1.,8.61946552381525E-15));
#48563=DIRECTION('',(6.76186946307289E-14,-1.,8.61946552381525E-15));
#48564=DIRECTION('',(0.707106781186591,-0.707106781186504,4.13746837958802E-15));
#48565=DIRECTION('',(1.,6.76186946307289E-14,-2.76820162751211E-15));
#48566=DIRECTION('',(0.707106781186484,0.707106781186611,-8.05229666459896E-15));
#48567=DIRECTION('',(-6.76186946307289E-14,1.,-8.61946552381525E-15));
#48568=DIRECTION('',(-0.707106781186581,0.707106781186514,-4.13746837958813E-15));
#48569=DIRECTION('',(-1.,-6.76186946307289E-14,2.76820162751211E-15));
#48570=DIRECTION('',(-0.707106781186495,-0.7071067811866,8.0522966645989E-15));
#48571=DIRECTION('center_axis',(-0.706676030840845,0.706676030840825,-0.03489949670248));
#48572=DIRECTION('ref_axis',(6.53747871958143E-16,-0.0493253122022489,-0.99878276595872));
#48573=DIRECTION('',(0.0348958507746445,-0.0144543346614283,-0.999286421306829));
#48574=DIRECTION('',(0.0144543346614127,-0.0348958507746925,-0.999286421306828));
#48575=DIRECTION('center_axis',(0.706676030840779,0.706676030840889,-0.0348994967025111));
#48576=DIRECTION('ref_axis',(4.83744971315161E-16,-0.0493253122022894,-0.998782765958718));
#48577=DIRECTION('',(-0.0144543346614135,-0.0348958507747033,-0.999286421306827));
#48578=DIRECTION('',(-0.0348958507746963,-0.0144543346614329,-0.999286421306827));
#48579=DIRECTION('center_axis',(-6.7674111992527E-14,0.999390827019095,
-0.0348994967025096));
#48580=DIRECTION('ref_axis',(-4.0665690358181E-16,-0.0348994967025096,-0.999390827019096));
#48581=DIRECTION('center_axis',(6.74808943053847E-14,-0.999390827019096,
-0.0348994967024927));
#48582=DIRECTION('ref_axis',(5.12637372416692E-15,-0.0348994967024927,0.999390827019096));
#48583=DIRECTION('',(-0.0144543346614183,0.0348958507746843,-0.999286421306828));
#48584=DIRECTION('',(0.0144543346614081,0.0348958507746774,-0.999286421306828));
#48585=DIRECTION('center_axis',(-0.706676030840789,-0.70667603084088,-0.0348994967024987));
#48586=DIRECTION('ref_axis',(6.04463415039793E-15,-0.0493253122022781,0.998782765958718));
#48587=DIRECTION('',(0.0348958507746425,0.0144543346614176,-0.999286421306829));
#48588=DIRECTION('center_axis',(2.76820162751153E-15,8.61946552381544E-15,
1.));
#48589=DIRECTION('ref_axis',(-6.76186946307289E-14,1.,-8.61946552381525E-15));
#48590=DIRECTION('center_axis',(0.999390827019096,6.72766881403301E-14,
-0.034899496702505));
#48591=DIRECTION('ref_axis',(-6.76186946307289E-14,1.,-8.61946552381525E-15));
#48592=DIRECTION('',(-0.0348958507746983,0.0144543346614128,-0.999286421306827));
#48593=DIRECTION('center_axis',(-0.999390827019097,-6.78783181575814E-14,
-0.034899496702471));
#48594=DIRECTION('ref_axis',(6.76186946307289E-14,-1.,8.61946552381525E-15));
#48595=DIRECTION('center_axis',(0.706676030840878,-0.706676030840792,-0.0348994967024981));
#48596=DIRECTION('ref_axis',(6.10708419553262E-15,-0.0493253122022712,0.998782765958719));
#48597=DIRECTION('center_axis',(-2.76820162751153E-15,-8.61946552381544E-15,
-1.));
#48598=DIRECTION('ref_axis',(6.76186946307289E-14,-1.,8.61946552381525E-15));
#48599=DIRECTION('center_axis',(-1.57236108655672E-14,-6.56288797468043E-14,
-1.));
#48600=DIRECTION('ref_axis',(-0.581108581114844,-0.813826036051129,6.25476162549096E-14));
#48601=DIRECTION('center_axis',(-6.30343034787932E-15,-8.61946552381568E-15,
-1.));
#48602=DIRECTION('ref_axis',(4.99425510288896E-14,-1.,8.61946552381536E-15));
#48603=DIRECTION('center_axis',(-6.30343034787932E-15,-8.61946552381568E-15,
-1.));
#48604=DIRECTION('ref_axis',(4.99425510288896E-14,-1.,8.61946552381536E-15));
#48605=DIRECTION('',(-0.410905818311989,-0.575461908797876,0.707106781186589));
#48606=DIRECTION('center_axis',(-2.76820162751153E-15,-8.61946552381544E-15,
-1.));
#48607=DIRECTION('ref_axis',(-7.14991605308202E-14,1.,-8.61946552381524E-15));
#48608=DIRECTION('center_axis',(2.76820162751153E-15,8.61946552381544E-15,
1.));
#48609=DIRECTION('ref_axis',(6.76186946307289E-14,-1.,8.61946552381525E-15));
#48610=DIRECTION('',(-2.76820162751153E-15,-8.61946552381544E-15,-1.));
#48611=DIRECTION('center_axis',(-9.83865906824712E-15,-8.61946552381592E-15,
-1.));
#48612=DIRECTION('ref_axis',(4.99425510288896E-14,-1.,8.61946552381543E-15));
#48613=DIRECTION('center_axis',(-9.83865906824712E-15,-8.61946552381592E-15,
-1.));
#48614=DIRECTION('ref_axis',(4.99425510288896E-14,-1.,8.61946552381543E-15));
#48615=DIRECTION('center_axis',(-3.19797012705699E-14,2.80182790159477E-14,
1.));
#48616=DIRECTION('ref_axis',(-0.581108581114993,0.813826036051022,-4.13856837783424E-14));
#48617=DIRECTION('',(-0.410905818312099,0.575461908797849,-0.707106781186548));
#48618=DIRECTION('center_axis',(1.,6.76186946307289E-14,-2.76820162751211E-15));
#48619=DIRECTION('ref_axis',(-6.76186946307289E-14,1.,-8.61946552381525E-15));
#48620=DIRECTION('',(6.76186946307289E-14,-1.,8.61946552381525E-15));
#48621=DIRECTION('',(2.76820162751153E-15,8.61946552381544E-15,1.));
#48622=DIRECTION('',(6.76186946307289E-14,-1.,8.61946552381525E-15));
#48623=DIRECTION('',(2.76820162751153E-15,8.61946552381544E-15,1.));
#48624=DIRECTION('center_axis',(0.500000000000024,0.866025403784425,-8.84877692442402E-15));
#48625=DIRECTION('ref_axis',(-2.76820162751153E-15,-8.61946552381544E-15,
-1.));
#48626=DIRECTION('',(0.866025403784471,-0.499999999999943,1.91239982968473E-15));
#48627=DIRECTION('',(2.76820162751153E-15,8.61946552381544E-15,1.));
#48628=DIRECTION('',(0.866025403784471,-0.499999999999943,1.91239982968473E-15));
#48629=DIRECTION('center_axis',(-0.500000000000142,0.866025403784357,1.33116358653071E-14));
#48630=DIRECTION('ref_axis',(-2.61873825433902E-15,1.38590238642998E-14,
-1.));
#48631=DIRECTION('',(0.866025403784404,0.500000000000061,-6.70706569413056E-15));
#48632=DIRECTION('',(2.76820162751153E-15,8.61946552381544E-15,1.));
#48633=DIRECTION('',(0.866025403784404,0.500000000000061,-6.70706569413056E-15));
#48634=DIRECTION('center_axis',(-1.,-6.76186946307289E-14,2.76820162751211E-15));
#48635=DIRECTION('ref_axis',(6.76186946307289E-14,-1.,8.61946552381525E-15));
#48636=DIRECTION('',(6.76186946307289E-14,-1.,8.61946552381525E-15));
#48637=DIRECTION('',(2.76820162751153E-15,8.61946552381544E-15,1.));
#48638=DIRECTION('',(-6.76186946307289E-14,1.,-8.61946552381525E-15));
#48639=DIRECTION('center_axis',(-0.500000000000026,-0.866025403784423,8.84877692442402E-15));
#48640=DIRECTION('ref_axis',(2.76820162751153E-15,8.61946552381544E-15,
1.));
#48641=DIRECTION('',(-0.866025403784473,0.499999999999941,-1.9123998296847E-15));
#48642=DIRECTION('',(2.76820162751153E-15,8.61946552381544E-15,1.));
#48643=DIRECTION('',(-0.866025403784473,0.499999999999941,-1.9123998296847E-15));
#48644=DIRECTION('center_axis',(2.76820162751153E-15,8.61946552381544E-15,
1.));
#48645=DIRECTION('ref_axis',(-6.76186946307289E-14,1.,-8.61946552381525E-15));
#48646=DIRECTION('',(-0.866025403784405,-0.500000000000058,6.70706569413054E-15));
#48647=DIRECTION('center_axis',(0.500000000000166,-0.866025403784343,6.08057529691127E-15));
#48648=DIRECTION('ref_axis',(2.76820162751153E-15,8.61946552381544E-15,
1.));
#48649=DIRECTION('',(-0.866025403784405,-0.500000000000058,6.70706569413054E-15));
#48650=DIRECTION('center_axis',(2.76820162751153E-15,8.61946552381544E-15,
1.));
#48651=DIRECTION('ref_axis',(-6.76186946307289E-14,1.,-8.61946552381525E-15));
#58607=CARTESIAN_POINT('',(0.,0.,0.));
#58608=CARTESIAN_POINT('Origin',(322.566620000606,298.539939847208,392.450702781549));
#58609=CARTESIAN_POINT('',(322.566620000606,298.546824263208,395.671178941549));
#58610=CARTESIAN_POINT('',(320.695173668754,298.546824263208,389.829795434059));
#58611=CARTESIAN_POINT('Origin',(322.566620000606,298.546824263208,392.450702781549));
#58612=CARTESIAN_POINT('Origin',(322.566620000606,298.546824263208,392.450702781549));
#58613=CARTESIAN_POINT('',(320.73517960089,298.477980103208,389.885822603897));
#58614=CARTESIAN_POINT('',(320.699174261967,298.539939847208,389.835398151043));
#58615=CARTESIAN_POINT('Origin',(322.566620000606,298.477980103208,392.450702781549));
#58616=CARTESIAN_POINT('Origin',(325.736133600606,298.477980103208,392.450702781549));
#58617=CARTESIAN_POINT('Origin',(322.566620000606,291.082459603103,392.450702781549));
#58618=CARTESIAN_POINT('',(322.566620000606,290.896525325314,392.450702781549));
#58619=CARTESIAN_POINT('',(320.695173668754,292.755868103209,389.829795434059));
#58620=CARTESIAN_POINT('',(322.379475367421,291.082459603103,392.1886120468));
#58621=CARTESIAN_POINT('',(322.566620000606,292.755868103209,395.671178941549));
#58622=CARTESIAN_POINT('Origin',(322.566620000606,292.755868103209,392.450702781549));
#58623=CARTESIAN_POINT('Origin',(322.566620000606,292.755868103209,392.450702781549));
#58624=CARTESIAN_POINT('Origin',(322.566620000606,295.651346183209,392.450702781549));
#58625=CARTESIAN_POINT('',(322.566620000606,295.651346183209,395.671178941549));
#58626=CARTESIAN_POINT('Origin',(322.566620000605,317.432476103209,392.450702781549));
#58627=CARTESIAN_POINT('',(322.566620000604,320.829980103208,396.362302781548));
#58628=CARTESIAN_POINT('Origin',(322.566620000604,320.829980103208,392.450702781549));
#58629=CARTESIAN_POINT('',(322.566620000605,314.034972103209,396.362302781549));
#58630=CARTESIAN_POINT('',(322.566620000605,317.432476103209,396.362302781548));
#58631=CARTESIAN_POINT('Origin',(322.566620000605,314.034972103209,392.450702781549));
#58632=CARTESIAN_POINT('Origin',(326.775501600604,320.829980103209,392.450702781549));
#58633=CARTESIAN_POINT('',(322.566620000604,320.829980103208,388.259702781549));
#58634=CARTESIAN_POINT('Origin',(322.566620000604,320.829980103208,392.450702781549));
#58635=CARTESIAN_POINT('Origin',(326.775501600605,314.034972103209,392.450702781549));
#58636=CARTESIAN_POINT('',(322.566620000605,314.034972103209,388.259702781549));
#58637=CARTESIAN_POINT('Origin',(322.566620000605,314.034972103209,392.450702781549));
#58638=CARTESIAN_POINT('Origin',(322.566620000605,317.432476103209,392.450702781549));
#58639=CARTESIAN_POINT('',(322.566620000605,317.432476103209,388.259702781549));
#58640=CARTESIAN_POINT('Origin',(427.66521554129,298.539939847217,497.549298322233));
#58641=CARTESIAN_POINT('',(427.66521554129,298.546824263216,500.769774482233));
#58642=CARTESIAN_POINT('',(425.793769209438,298.546824263216,494.928390974743));
#58643=CARTESIAN_POINT('Origin',(427.66521554129,298.546824263216,497.549298322233));
#58644=CARTESIAN_POINT('Origin',(427.66521554129,298.546824263216,497.549298322233));
#58645=CARTESIAN_POINT('',(425.833775141574,298.477980103216,494.984418144581));
#58646=CARTESIAN_POINT('',(425.797769802652,298.539939847217,494.933993691727));
#58647=CARTESIAN_POINT('Origin',(427.66521554129,298.477980103217,497.549298322233));
#58648=CARTESIAN_POINT('Origin',(430.83472914129,298.477980103217,497.549298322233));
#58649=CARTESIAN_POINT('Origin',(427.665215541291,291.082459603111,497.549298322233));
#58650=CARTESIAN_POINT('',(427.665215541291,290.896525325322,497.549298322233));
#58651=CARTESIAN_POINT('',(425.793769209439,292.755868103217,494.928390974743));
#58652=CARTESIAN_POINT('',(427.478070908106,291.082459603111,497.287207587484));
#58653=CARTESIAN_POINT('',(427.665215541291,292.755868103217,500.769774482233));
#58654=CARTESIAN_POINT('Origin',(427.665215541291,292.755868103217,497.549298322233));
#58655=CARTESIAN_POINT('Origin',(427.665215541291,292.755868103217,497.549298322233));
#58656=CARTESIAN_POINT('Origin',(427.66521554129,295.651346183217,497.549298322233));
#58657=CARTESIAN_POINT('',(427.66521554129,295.651346183217,500.769774482233));
#58658=CARTESIAN_POINT('Origin',(427.665215541289,317.432476103217,497.549298322232));
#58659=CARTESIAN_POINT('',(427.665215541289,320.829980103216,501.460898322232));
#58660=CARTESIAN_POINT('Origin',(427.665215541289,320.829980103217,497.549298322232));
#58661=CARTESIAN_POINT('',(427.665215541289,314.034972103217,501.460898322232));
#58662=CARTESIAN_POINT('',(427.665215541289,317.432476103217,501.460898322232));
#58663=CARTESIAN_POINT('Origin',(427.665215541289,314.034972103217,497.549298322232));
#58664=CARTESIAN_POINT('Origin',(431.874097141289,320.829980103217,497.549298322232));
#58665=CARTESIAN_POINT('',(427.665215541289,320.829980103216,493.358298322232));
#58666=CARTESIAN_POINT('Origin',(427.665215541289,320.829980103216,497.549298322232));
#58667=CARTESIAN_POINT('Origin',(431.874097141289,314.034972103217,497.549298322232));
#58668=CARTESIAN_POINT('',(427.665215541289,314.034972103217,493.358298322232));
#58669=CARTESIAN_POINT('Origin',(427.665215541289,314.034972103217,497.549298322232));
#58670=CARTESIAN_POINT('Origin',(427.665215541289,317.432476103217,497.549298322232));
#58671=CARTESIAN_POINT('',(427.665215541289,317.432476103217,493.358298322232));
#58672=CARTESIAN_POINT('Origin',(319.69547489095,274.10535930321,526.415998247891));
#58673=CARTESIAN_POINT('',(321.292075273455,271.869365888763,526.422077991891));
#58674=CARTESIAN_POINT('',(319.69547489095,271.35785146321,526.422077991891));
#58675=CARTESIAN_POINT('Origin',(319.69547489095,274.10535930321,526.422077991891));
#58676=CARTESIAN_POINT('',(321.256745359361,271.918844428361,526.361280551891));
#58677=CARTESIAN_POINT('',(321.288542282045,271.874313742723,526.415998247891));
#58678=CARTESIAN_POINT('Origin',(319.69547489095,274.10535930321,526.361280551891));
#58679=CARTESIAN_POINT('Origin',(319.69547489095,274.10535930321,526.422077991891));
#58680=CARTESIAN_POINT('Origin',(316.99088289095,274.105359303209,526.361280551891));
#58681=CARTESIAN_POINT('Origin',(319.69547489095,274.10535930321,523.709439271891));
#58682=CARTESIAN_POINT('',(319.69547489095,271.35785146321,520.996800551891));
#58683=CARTESIAN_POINT('',(318.098874508445,276.341352717656,520.996800551891));
#58684=CARTESIAN_POINT('Origin',(319.69547489095,274.10535930321,520.996800551891));
#58685=CARTESIAN_POINT('Origin',(319.69547489095,274.10535930321,520.996800551891));
#58686=CARTESIAN_POINT('',(319.69547489095,271.35785146321,523.709439271891));
#58687=CARTESIAN_POINT('Origin',(319.69547489095,274.10535930321,519.569153599969));
#58688=CARTESIAN_POINT('',(319.69547489095,274.10535930321,519.410526160866));
#58689=CARTESIAN_POINT('',(319.535814852699,274.328958644654,519.569153599969));
#58690=CARTESIAN_POINT('Origin',(319.69547489095,274.10535930321,543.795840551891));
#58691=CARTESIAN_POINT('',(319.69547489095,277.45815930321,548.713280551891));
#58692=CARTESIAN_POINT('Origin',(319.69547489095,274.10535930321,548.713280551891));
#58693=CARTESIAN_POINT('',(319.69547489095,277.45815930321,538.878400551891));
#58694=CARTESIAN_POINT('',(319.69547489095,277.45815930321,543.795840551891));
#58695=CARTESIAN_POINT('Origin',(319.69547489095,274.10535930321,538.878400551891));
#58696=CARTESIAN_POINT('Origin',(316.04539329095,274.10535930321,548.713280551891));
#58697=CARTESIAN_POINT('',(319.69547489095,270.47315930321,548.713280551891));
#58698=CARTESIAN_POINT('Origin',(319.69547489095,274.10535930321,548.713280551891));
#58699=CARTESIAN_POINT('Origin',(319.69547489095,274.10535930321,543.795840551891));
#58700=CARTESIAN_POINT('',(319.69547489095,270.47315930321,538.878400551891));
#58701=CARTESIAN_POINT('Origin',(319.69547489095,274.10535930321,538.878400551891));
#58702=CARTESIAN_POINT('',(319.69547489095,270.47315930321,543.795840551891));
#58703=CARTESIAN_POINT('Origin',(323.34555649095,274.10535930321,538.878400551891));
#58704=CARTESIAN_POINT('Origin',(427.665215541289,317.432476103216,392.450702781548));
#58705=CARTESIAN_POINT('',(427.665215541289,320.829980103215,396.362302781548));
#58706=CARTESIAN_POINT('Origin',(427.665215541289,320.829980103215,392.450702781548));
#58707=CARTESIAN_POINT('',(427.665215541289,314.034972103216,396.362302781548));
#58708=CARTESIAN_POINT('',(427.665215541289,317.432476103216,396.362302781548));
#58709=CARTESIAN_POINT('Origin',(427.665215541289,314.034972103216,392.450702781548));
#58710=CARTESIAN_POINT('Origin',(431.874097141288,320.829980103216,392.450702781548));
#58711=CARTESIAN_POINT('',(427.665215541288,320.829980103216,388.259702781548));
#58712=CARTESIAN_POINT('Origin',(427.665215541288,320.829980103216,392.450702781548));
#58713=CARTESIAN_POINT('Origin',(427.665215541289,317.432476103216,392.450702781548));
#58714=CARTESIAN_POINT('',(427.665215541289,314.034972103216,388.259702781548));
#58715=CARTESIAN_POINT('',(427.665215541289,317.432476103216,388.259702781548));
#58716=CARTESIAN_POINT('Origin',(427.665215541289,314.034972103216,392.450702781548));
#58717=CARTESIAN_POINT('Origin',(431.874097141289,314.034972103216,392.450702781548));
#58718=CARTESIAN_POINT('Origin',(427.66521554129,298.539939847216,392.450702781548));
#58719=CARTESIAN_POINT('',(427.66521554129,298.546824263215,395.671178941548));
#58720=CARTESIAN_POINT('',(425.793769209438,298.546824263215,389.829795434059));
#58721=CARTESIAN_POINT('Origin',(427.66521554129,298.546824263215,392.450702781548));
#58722=CARTESIAN_POINT('Origin',(427.66521554129,298.546824263215,392.450702781548));
#58723=CARTESIAN_POINT('',(425.833775141574,298.477980103215,389.885822603897));
#58724=CARTESIAN_POINT('',(425.797769802652,298.539939847215,389.835398151042));
#58725=CARTESIAN_POINT('Origin',(427.66521554129,298.477980103215,392.450702781548));
#58726=CARTESIAN_POINT('Origin',(430.83472914129,298.477980103216,392.450702781548));
#58727=CARTESIAN_POINT('Origin',(427.66521554129,295.651346183216,392.450702781548));
#58728=CARTESIAN_POINT('',(427.66521554129,292.755868103216,395.671178941548));
#58729=CARTESIAN_POINT('',(425.793769209438,292.755868103216,389.829795434059));
#58730=CARTESIAN_POINT('Origin',(427.66521554129,292.755868103216,392.450702781548));
#58731=CARTESIAN_POINT('Origin',(427.66521554129,292.755868103216,392.450702781548));
#58732=CARTESIAN_POINT('',(427.66521554129,295.651346183216,395.671178941548));
#58733=CARTESIAN_POINT('Origin',(427.66521554129,291.082459603111,392.450702781548));
#58734=CARTESIAN_POINT('',(427.66521554129,290.896525325321,392.450702781548));
#58735=CARTESIAN_POINT('',(427.478070908105,291.082459603111,392.188612046799));
#58736=CARTESIAN_POINT('Origin',(322.566620000605,317.43247610321,497.549298322233));
#58737=CARTESIAN_POINT('',(322.566620000605,320.829980103209,501.460898322233));
#58738=CARTESIAN_POINT('Origin',(322.566620000605,320.829980103209,497.549298322233));
#58739=CARTESIAN_POINT('',(322.566620000605,314.03497210321,501.460898322233));
#58740=CARTESIAN_POINT('',(322.566620000605,317.43247610321,501.460898322233));
#58741=CARTESIAN_POINT('Origin',(322.566620000605,314.03497210321,497.549298322233));
#58742=CARTESIAN_POINT('Origin',(326.775501600605,320.82998010321,497.549298322233));
#58743=CARTESIAN_POINT('',(322.566620000605,320.829980103209,493.358298322233));
#58744=CARTESIAN_POINT('Origin',(322.566620000605,320.829980103209,497.549298322233));
#58745=CARTESIAN_POINT('Origin',(322.566620000605,317.43247610321,497.549298322233));
#58746=CARTESIAN_POINT('',(322.566620000605,314.03497210321,493.358298322233));
#58747=CARTESIAN_POINT('',(322.566620000605,317.432476103209,493.358298322233));
#58748=CARTESIAN_POINT('Origin',(322.566620000605,314.03497210321,497.549298322233));
#58749=CARTESIAN_POINT('Origin',(326.775501600605,314.03497210321,497.549298322233));
#58750=CARTESIAN_POINT('Origin',(322.566620000606,298.539939847209,497.549298322233));
#58751=CARTESIAN_POINT('',(322.566620000606,298.546824263209,500.769774482233));
#58752=CARTESIAN_POINT('',(320.695173668754,298.546824263209,494.928390974743));
#58753=CARTESIAN_POINT('Origin',(322.566620000606,298.546824263209,497.549298322233));
#58754=CARTESIAN_POINT('Origin',(322.566620000606,298.546824263209,497.549298322233));
#58755=CARTESIAN_POINT('',(320.73517960089,298.477980103209,494.984418144581));
#58756=CARTESIAN_POINT('',(320.699174261968,298.539939847209,494.933993691727));
#58757=CARTESIAN_POINT('Origin',(322.566620000606,298.477980103209,497.549298322233));
#58758=CARTESIAN_POINT('Origin',(325.736133600606,298.47798010321,497.549298322233));
#58759=CARTESIAN_POINT('Origin',(322.566620000606,295.65134618321,497.549298322233));
#58760=CARTESIAN_POINT('',(322.566620000607,292.75586810321,500.769774482233));
#58761=CARTESIAN_POINT('',(320.695173668754,292.75586810321,494.928390974743));
#58762=CARTESIAN_POINT('Origin',(322.566620000607,292.75586810321,497.549298322233));
#58763=CARTESIAN_POINT('Origin',(322.566620000607,292.75586810321,497.549298322233));
#58764=CARTESIAN_POINT('',(322.566620000606,295.65134618321,500.769774482233));
#58765=CARTESIAN_POINT('Origin',(322.566620000607,291.082459603104,497.549298322233));
#58766=CARTESIAN_POINT('',(322.566620000607,290.896525325315,497.549298322233));
#58767=CARTESIAN_POINT('',(322.379475367421,291.082459603104,497.287207587484));
#58768=CARTESIAN_POINT('Origin',(464.492340170948,302.000655303219,445.000000551888));
#58769=CARTESIAN_POINT('',(271.071258570948,302.000655303206,530.262016502755));
#58770=CARTESIAN_POINT('',(271.071258570948,302.000655303205,359.737984601026));
#58771=CARTESIAN_POINT('',(271.071258570948,302.000655303206,530.262016502755));
#58772=CARTESIAN_POINT('',(464.474458570948,302.00065530322,530.262016502755));
#58773=CARTESIAN_POINT('',(271.071258570948,302.000655303206,530.262016502755));
#58774=CARTESIAN_POINT('',(464.474458570947,302.000655303218,359.737984601026));
#58775=CARTESIAN_POINT('',(464.474458570948,302.00065530322,530.262016502755));
#58776=CARTESIAN_POINT('',(407.733894628553,302.000655303214,359.737984601026));
#58777=CARTESIAN_POINT('',(407.733894628553,302.000655303214,359.737984601026));
#58778=CARTESIAN_POINT('',(404.706788582958,302.000655303214,373.473600551891));
#58779=CARTESIAN_POINT('Ctrl Pts',(404.706788582958,302.000655303214,373.473600551891));
#58780=CARTESIAN_POINT('Ctrl Pts',(406.157952436569,302.000655303214,368.402118484692));
#58781=CARTESIAN_POINT('Ctrl Pts',(407.733894628554,302.000655303214,359.737984601022));
#58782=CARTESIAN_POINT('',(426.614925770948,302.000655303216,373.47360055189));
#58783=CARTESIAN_POINT('',(426.614925770948,302.000655303216,373.47360055189));
#58784=CARTESIAN_POINT('',(446.642317770948,302.000655303217,393.50099255189));
#58785=CARTESIAN_POINT('',(446.642317770948,302.000655303217,393.50099255189));
#58786=CARTESIAN_POINT('',(446.642317770948,302.000655303218,496.49900855189));
#58787=CARTESIAN_POINT('',(446.642317770948,302.000655303218,496.499008551891));
#58788=CARTESIAN_POINT('',(426.614925770948,302.000655303217,516.52640055189));
#58789=CARTESIAN_POINT('',(426.614925770948,302.000655303217,516.52640055189));
#58790=CARTESIAN_POINT('',(323.616909770948,302.00065530321,516.526400551891));
#58791=CARTESIAN_POINT('',(323.616909770948,302.00065530321,516.526400551891));
#58792=CARTESIAN_POINT('',(303.589517770948,302.000655303208,496.499008551891));
#58793=CARTESIAN_POINT('',(303.589517770948,302.000655303208,496.499008551891));
#58794=CARTESIAN_POINT('',(303.589517770948,302.000655303208,393.500992551891));
#58795=CARTESIAN_POINT('',(303.589517770948,302.000655303208,393.500992551891));
#58796=CARTESIAN_POINT('',(316.405264128415,302.000655303208,380.685246194424));
#58797=CARTESIAN_POINT('',(316.405264128415,302.000655303208,380.685246194424));
#58798=CARTESIAN_POINT('',(315.741199156673,302.000655303208,379.6288809737));
#58799=CARTESIAN_POINT('',(315.741199156673,302.000655303208,379.6288809737));
#58800=CARTESIAN_POINT('',(310.311060913343,302.000655303208,359.737984601026));
#58801=CARTESIAN_POINT('Ctrl Pts',(310.311060913342,302.000655303208,359.737984601022));
#58802=CARTESIAN_POINT('Ctrl Pts',(313.19124860752,302.000655303208,375.572532288989));
#58803=CARTESIAN_POINT('Ctrl Pts',(315.741199156672,302.000655303208,379.628880973699));
#58804=CARTESIAN_POINT('',(271.071258570948,302.000655303205,359.737984601026));
#58805=CARTESIAN_POINT('Origin',(359.02247777095,249.071311553972,331.655798731546));
#58806=CARTESIAN_POINT('',(367.706500485028,311.19711150173,330.571673357733));
#58807=CARTESIAN_POINT('',(350.338455056865,311.197111501729,330.571673357734));
#58808=CARTESIAN_POINT('Origin',(359.022477770949,249.407877716595,330.571673357734));
#58809=CARTESIAN_POINT('',(350.556449206845,307.437429180769,373.473600551891));
#58810=CARTESIAN_POINT('',(350.338455056865,311.197111501729,330.571673357734));
#58811=CARTESIAN_POINT('',(367.488506335048,307.43742918077,373.473600551891));
#58812=CARTESIAN_POINT('Origin',(359.02247777095,247.199284325311,373.473600551891));
#58813=CARTESIAN_POINT('',(367.488506335048,307.43742918077,373.473600551891));
#58814=CARTESIAN_POINT('Origin',(385.304007296866,308.72551700596,330.55385980262));
#58815=CARTESIAN_POINT('',(402.378703501902,302.533931748012,373.473600551891));
#58816=CARTESIAN_POINT('',(367.488506335048,307.43742918077,373.473600551891));
#58817=CARTESIAN_POINT('',(402.901080310565,306.250835876051,330.571673357733));
#58818=CARTESIAN_POINT('',(402.378703501902,302.533931748012,373.473600551891));
#58819=CARTESIAN_POINT('',(402.901080310565,306.250835876051,330.571673357733));
#58820=CARTESIAN_POINT('Origin',(359.022477770951,245.494607052455,331.655798731566));
#58821=CARTESIAN_POINT('',(350.338455056874,183.368807104691,330.571673357735));
#58822=CARTESIAN_POINT('',(367.706500485037,183.368807104693,330.571673357735));
#58823=CARTESIAN_POINT('Origin',(359.022477770951,245.158040889847,330.571673357734));
#58824=CARTESIAN_POINT('',(367.488506335057,187.128489425653,373.473600551892));
#58825=CARTESIAN_POINT('',(367.706500485037,183.368807104693,330.571673357735));
#58826=CARTESIAN_POINT('',(350.556449206854,187.128489425652,373.473600551892));
#58827=CARTESIAN_POINT('Origin',(359.022477770951,247.366634281122,373.473600551892));
#58828=CARTESIAN_POINT('',(350.556449206854,187.128489425652,373.473600551892));
#58829=CARTESIAN_POINT('Origin',(332.740948245037,185.840401600462,330.553859802622));
#58830=CARTESIAN_POINT('',(323.616909770955,190.91459478447,373.473600551892));
#58831=CARTESIAN_POINT('',(350.556449206854,187.128489425652,373.473600551892));
#58832=CARTESIAN_POINT('',(316.405264128422,192.565263303208,380.685246194425));
#58833=CARTESIAN_POINT('',(323.616909770955,190.91459478447,373.473600551892));
#58834=CARTESIAN_POINT('',(315.74119915668,192.565263303208,379.628880973701));
#58835=CARTESIAN_POINT('',(316.405264128422,192.565263303208,380.685246194425));
#58836=CARTESIAN_POINT('',(315.143875231337,188.31508273037,330.571673357735));
#58837=CARTESIAN_POINT('',(315.74119915668,192.565263303208,379.628880973701));
#58838=CARTESIAN_POINT('',(315.143875231337,188.31508273037,330.571673357735));
#58839=CARTESIAN_POINT('Origin',(332.740948245028,308.725517005956,330.553859802621));
#58840=CARTESIAN_POINT('',(315.143875231329,306.250835876046,330.571673357734));
#58841=CARTESIAN_POINT('',(350.338455056865,311.197111501729,330.571673357734));
#58842=CARTESIAN_POINT('',(315.741199156673,302.000655303208,379.6288809737));
#58843=CARTESIAN_POINT('',(323.616909770947,303.651323821948,373.473600551891));
#58844=CARTESIAN_POINT('',(316.405264128415,302.000655303208,380.685246194424));
#58845=CARTESIAN_POINT('',(323.616909770947,303.651323821948,373.473600551891));
#58846=CARTESIAN_POINT('Origin',(426.632807370947,311.415317703215,373.47360055189));
#58847=CARTESIAN_POINT('',(323.616909770946,320.829980103208,373.473600551891));
#58848=CARTESIAN_POINT('',(323.616909770947,303.651323821948,373.473600551891));
#58849=CARTESIAN_POINT('',(426.614925770946,320.829980103215,373.47360055189));
#58850=CARTESIAN_POINT('',(323.616909770946,320.829980103208,373.473600551891));
#58851=CARTESIAN_POINT('',(426.614925770948,302.000655303215,373.47360055189));
#58852=CARTESIAN_POINT('Origin',(400.433645843278,288.694127375541,373.473600551888));
#58853=CARTESIAN_POINT('Origin',(426.632807370956,183.088015303216,373.473600551891));
#58854=CARTESIAN_POINT('',(402.378703501909,192.031986858416,373.473600551891));
#58855=CARTESIAN_POINT('',(402.378703501909,192.031986858416,373.473600551891));
#58856=CARTESIAN_POINT('',(404.706788582966,192.565263303214,373.473600551891));
#58857=CARTESIAN_POINT('Origin',(400.433645843284,205.871791230884,373.473600551894));
#58858=CARTESIAN_POINT('',(426.614925770955,192.565263303216,373.473600551891));
#58859=CARTESIAN_POINT('',(404.706788582966,192.565263303214,373.473600551891));
#58860=CARTESIAN_POINT('',(426.614925770956,173.610767303216,373.473600551892));
#58861=CARTESIAN_POINT('',(426.614925770956,173.610767303216,373.473600551892));
#58862=CARTESIAN_POINT('',(323.616909770956,173.610767303209,373.473600551892));
#58863=CARTESIAN_POINT('',(323.616909770956,173.610767303209,373.473600551892));
#58864=CARTESIAN_POINT('',(323.616909770956,173.610767303209,373.473600551892));
#58865=CARTESIAN_POINT('Origin',(385.304007296874,185.840401600465,330.553859802621));
#58866=CARTESIAN_POINT('',(402.901080310573,188.315082730376,330.571673357734));
#58867=CARTESIAN_POINT('',(367.706500485037,183.368807104693,330.571673357735));
#58868=CARTESIAN_POINT('',(402.378703501909,192.031986858416,373.473600551891));
#58869=CARTESIAN_POINT('Origin',(367.772858570951,182.141307303882,330.571673357735));
#58870=CARTESIAN_POINT('',(410.104986828528,273.835075933065,330.571673357763));
#58871=CARTESIAN_POINT('Origin',(400.433645843278,288.694127375543,330.571673357734));
#58872=CARTESIAN_POINT('',(464.474458570949,273.835075933041,330.571673357734));
#58873=CARTESIAN_POINT('',(464.474458570949,273.835075933041,330.571673357734));
#58874=CARTESIAN_POINT('',(464.474458570953,220.730842673395,330.571673357734));
#58875=CARTESIAN_POINT('',(464.474458570953,220.730842673395,330.571673357734));
#58876=CARTESIAN_POINT('',(410.104986828532,220.730842673363,330.571673357763));
#58877=CARTESIAN_POINT('',(410.104986828532,220.730842673391,330.571673357734));
#58878=CARTESIAN_POINT('Origin',(400.433645843284,205.871791230884,330.571673357734));
#58879=CARTESIAN_POINT('',(307.939968713374,220.730842673356,330.571673357763));
#58880=CARTESIAN_POINT('Origin',(317.611309698625,205.871791230878,330.571673357734));
#58881=CARTESIAN_POINT('',(271.071258570953,220.730842673381,330.571673357734));
#58882=CARTESIAN_POINT('',(271.071258570953,220.730842673381,330.571673357734));
#58883=CARTESIAN_POINT('',(271.071258570949,273.835075933028,330.571673357734));
#58884=CARTESIAN_POINT('',(271.071258570949,273.835075933028,330.571673357734));
#58885=CARTESIAN_POINT('',(307.93996871337,273.835075933058,330.571673357763));
#58886=CARTESIAN_POINT('',(307.93996871337,273.83507593303,330.571673357734));
#58887=CARTESIAN_POINT('Origin',(317.611309698619,288.694127375538,330.571673357734));
#58888=CARTESIAN_POINT('',(359.022477770953,217.089877703211,330.571673357734));
#58889=CARTESIAN_POINT('Origin',(359.022477770951,247.282959303211,330.571673357734));
#58890=CARTESIAN_POINT('Origin',(447.762010570948,291.986959303217,369.00320055189));
#58891=CARTESIAN_POINT('',(464.474458570948,296.695184583218,369.00320055189));
#58892=CARTESIAN_POINT('Origin',(464.474458570948,291.986959303218,369.00320055189));
#58893=CARTESIAN_POINT('',(431.049562570948,296.695184583216,369.00320055189));
#58894=CARTESIAN_POINT('',(447.762010570948,296.695184583217,369.00320055189));
#58895=CARTESIAN_POINT('',(431.049562570947,295.818635619674,371.739190663921));
#58896=CARTESIAN_POINT('Origin',(431.049562570948,291.986959303216,369.003200551891));
#58897=CARTESIAN_POINT('Origin',(431.049562570948,291.986959303216,369.003200551891));
#58898=CARTESIAN_POINT('Origin',(464.492340170949,287.917865618129,345.15482897938));
#58899=CARTESIAN_POINT('Origin',(400.433645843277,287.197585189467,344.408956761074));
#58900=CARTESIAN_POINT('',(464.474458570949,273.835075933041,330.571673357734));
#58901=CARTESIAN_POINT('Origin',(464.474458570951,247.282959303218,330.553791757734));
#58902=CARTESIAN_POINT('',(464.474458570948,297.532978550114,534.888431212814));
#58903=CARTESIAN_POINT('',(464.474458570948,302.00065530322,530.262016502755));
#58904=CARTESIAN_POINT('',(464.474458570952,247.28295930322,536.643200551891));
#58905=CARTESIAN_POINT('',(464.474458570952,247.28295930322,536.643200551891));
#58906=CARTESIAN_POINT('',(464.474458570955,197.032940056326,534.888431212815));
#58907=CARTESIAN_POINT('',(464.474458570955,197.032940056326,534.888431212815));
#58908=CARTESIAN_POINT('',(464.474458570955,192.56526330322,530.262016502756));
#58909=CARTESIAN_POINT('',(464.474458570955,197.032940056326,534.888431212815));
#58910=CARTESIAN_POINT('',(464.474458570955,192.565263303218,359.737984601027));
#58911=CARTESIAN_POINT('',(464.474458570955,192.565263303218,359.737984601027));
#58912=CARTESIAN_POINT('',(464.474458570953,220.730842673395,330.571673357734));
#58913=CARTESIAN_POINT('',(464.474458570954,207.287184583218,369.003200551891));
#58914=CARTESIAN_POINT('Origin',(464.474458570954,202.578959303218,369.003200551891));
#58915=CARTESIAN_POINT('',(464.474458570949,296.695184583219,520.99680055189));
#58916=CARTESIAN_POINT('Origin',(464.474458570949,291.98695930322,520.99680055189));
#58917=CARTESIAN_POINT('',(464.474458570955,207.287184583219,520.996800551891));
#58918=CARTESIAN_POINT('Origin',(464.474458570955,202.578959303219,520.996800551891));
#58919=CARTESIAN_POINT('Origin',(447.762010570954,202.578959303217,369.003200551891));
#58920=CARTESIAN_POINT('',(431.049562570954,207.287184583216,369.003200551891));
#58921=CARTESIAN_POINT('',(447.762010570954,207.287184583217,369.003200551891));
#58922=CARTESIAN_POINT('',(431.049562570953,206.410635619674,371.739190663922));
#58923=CARTESIAN_POINT('Origin',(431.049562570954,202.578959303216,369.003200551891));
#58924=CARTESIAN_POINT('Origin',(431.049562570954,202.578959303216,369.003200551891));
#58925=CARTESIAN_POINT('Origin',(464.492340170954,206.648052988306,345.15482897938));
#58926=CARTESIAN_POINT('',(407.73389462856,192.565263303214,359.737984601027));
#58927=CARTESIAN_POINT('',(407.73389462856,192.565263303214,359.737984601027));
#58928=CARTESIAN_POINT('Origin',(400.433645843283,207.36833341696,344.408956761074));
#58929=CARTESIAN_POINT('Origin',(464.492340170953,222.157949679773,535.765815882353));
#58930=CARTESIAN_POINT('',(271.071258570955,197.032940056313,534.888431212815));
#58931=CARTESIAN_POINT('',(271.071258570955,197.032940056313,534.888431212815));
#58932=CARTESIAN_POINT('',(445.915945087977,247.282959303218,536.643200551891));
#58933=CARTESIAN_POINT('',(445.915945087977,247.282959303218,536.643200551891));
#58934=CARTESIAN_POINT('',(438.427890453927,247.282959303217,536.643200551891));
#58935=CARTESIAN_POINT('Origin',(442.171917770952,250.687930181368,536.762104755053));
#58936=CARTESIAN_POINT('',(367.594537087977,247.282959303213,536.643200551891));
#58937=CARTESIAN_POINT('',(367.594537087977,247.282959303213,536.643200551891));
#58938=CARTESIAN_POINT('',(360.106482453926,247.282959303212,536.643200551891));
#58939=CARTESIAN_POINT('Origin',(363.850509770952,243.527086301937,536.512042576573));
#58940=CARTESIAN_POINT('',(333.509010890952,247.282959303211,536.643200551891));
#58941=CARTESIAN_POINT('',(333.509010890952,247.282959303211,536.643200551891));
#58942=CARTESIAN_POINT('',(332.869141902422,210.624889501466,535.363072546332));
#58943=CARTESIAN_POINT('',(332.869141902422,210.624889501466,535.363072546333));
#58944=CARTESIAN_POINT('',(327.592975586647,205.44001530321,535.182012749611));
#58945=CARTESIAN_POINT('',(327.592975586647,205.44001530321,535.182012749612));
#58946=CARTESIAN_POINT('',(271.071258570955,205.440015303207,535.182012749612));
#58947=CARTESIAN_POINT('',(271.071258570955,205.440015303207,535.182012749612));
#58948=CARTESIAN_POINT('',(271.071258570955,197.032940056313,534.888431212815));
#58949=CARTESIAN_POINT('Origin',(447.762010570955,202.578959303218,520.996800551891));
#58950=CARTESIAN_POINT('',(431.049562570954,207.287184583217,520.996800551891));
#58951=CARTESIAN_POINT('',(447.762010570954,207.287184583218,520.996800551891));
#58952=CARTESIAN_POINT('',(431.049562570954,206.410635619676,523.732790663922));
#58953=CARTESIAN_POINT('Origin',(431.049562570955,202.578959303217,520.996800551891));
#58954=CARTESIAN_POINT('Origin',(431.049562570955,202.578959303217,520.996800551891));
#58955=CARTESIAN_POINT('Origin',(464.492340170955,194.799101679773,532.575223857785));
#58956=CARTESIAN_POINT('',(271.071258570955,192.565263303206,530.262016502756));
#58957=CARTESIAN_POINT('',(271.071258570955,192.565263303207,530.262016502756));
#58958=CARTESIAN_POINT('',(271.071258570955,192.565263303207,530.262016502756));
#58959=CARTESIAN_POINT('Origin',(464.492340170948,299.766816926667,532.575223857784));
#58960=CARTESIAN_POINT('',(271.071258570948,297.5329785501,534.888431212814));
#58961=CARTESIAN_POINT('',(271.071258570948,297.5329785501,534.888431212814));
#58962=CARTESIAN_POINT('',(271.071258570948,297.5329785501,534.888431212814));
#58963=CARTESIAN_POINT('Origin',(447.762010570949,291.986959303218,520.99680055189));
#58964=CARTESIAN_POINT('',(431.049562570948,296.695184583217,520.99680055189));
#58965=CARTESIAN_POINT('',(447.762010570948,296.695184583218,520.99680055189));
#58966=CARTESIAN_POINT('',(431.049562570948,295.818635619675,523.732790663921));
#58967=CARTESIAN_POINT('Origin',(431.049562570949,291.986959303217,520.996800551891));
#58968=CARTESIAN_POINT('Origin',(431.049562570949,291.986959303217,520.996800551891));
#58969=CARTESIAN_POINT('Origin',(464.49234017095,272.407968926666,535.765815882352));
#58970=CARTESIAN_POINT('',(271.071258570949,289.125903303207,535.182012749611));
#58971=CARTESIAN_POINT('',(271.071258570949,289.125903303207,535.182012749611));
#58972=CARTESIAN_POINT('',(327.592975586641,289.12590330321,535.182012749611));
#58973=CARTESIAN_POINT('',(327.592975586641,289.12590330321,535.182012749611));
#58974=CARTESIAN_POINT('',(332.869141902417,283.941029104955,535.363072546332));
#58975=CARTESIAN_POINT('',(332.869141902417,283.941029104955,535.363072546332));
#58976=CARTESIAN_POINT('',(333.509010890952,247.282959303211,536.643200551891));
#58977=CARTESIAN_POINT('Origin',(363.850509770952,243.877988425064,536.762104755053));
#58978=CARTESIAN_POINT('Origin',(442.171917770952,251.038832304494,536.512042576573));
#58979=CARTESIAN_POINT('Origin',(464.492340170955,192.565263303219,445.000000551889));
#58980=CARTESIAN_POINT('',(271.071258570955,192.565263303205,413.628947618471));
#58981=CARTESIAN_POINT('',(271.071258570955,192.565263303205,413.628947618471));
#58982=CARTESIAN_POINT('',(271.071258570955,192.565263303205,404.844653485312));
#58983=CARTESIAN_POINT('Origin',(267.168274890955,192.565263303205,409.236800551892));
#58984=CARTESIAN_POINT('',(271.071258570955,192.565263303205,359.737984601027));
#58985=CARTESIAN_POINT('',(271.071258570955,192.565263303205,359.737984601027));
#58986=CARTESIAN_POINT('',(310.31106091335,192.565263303208,359.737984601027));
#58987=CARTESIAN_POINT('',(271.071258570955,192.565263303205,359.737984601027));
#58988=CARTESIAN_POINT('Ctrl Pts',(315.741199156679,192.565263303208,379.6288809737));
#58989=CARTESIAN_POINT('Ctrl Pts',(313.191248607527,192.565263303208,375.57253228899));
#58990=CARTESIAN_POINT('Ctrl Pts',(310.311060913349,192.565263303208,359.737984601023));
#58991=CARTESIAN_POINT('',(303.589517770955,192.565263303208,393.500992551892));
#58992=CARTESIAN_POINT('',(303.589517770955,192.565263303208,393.500992551892));
#58993=CARTESIAN_POINT('',(303.589517770955,192.565263303208,496.499008551892));
#58994=CARTESIAN_POINT('',(303.589517770955,192.565263303208,496.499008551892));
#58995=CARTESIAN_POINT('',(323.616909770955,192.56526330321,516.526400551892));
#58996=CARTESIAN_POINT('',(323.616909770955,192.56526330321,516.526400551892));
#58997=CARTESIAN_POINT('',(426.614925770955,192.565263303217,516.526400551891));
#58998=CARTESIAN_POINT('',(426.614925770955,192.565263303217,516.526400551891));
#58999=CARTESIAN_POINT('',(446.642317770955,192.565263303218,496.499008551891));
#59000=CARTESIAN_POINT('',(446.642317770955,192.565263303218,496.499008551891));
#59001=CARTESIAN_POINT('',(446.642317770955,192.565263303217,393.500992551891));
#59002=CARTESIAN_POINT('',(446.642317770955,192.565263303217,393.500992551891));
#59003=CARTESIAN_POINT('',(426.614925770955,192.565263303216,373.473600551891));
#59004=CARTESIAN_POINT('Ctrl Pts',(407.733894628561,192.565263303214,359.737984601023));
#59005=CARTESIAN_POINT('Ctrl Pts',(406.157952436577,192.565263303214,368.402118484693));
#59006=CARTESIAN_POINT('Ctrl Pts',(404.706788582965,192.565263303214,373.473600551892));
#59007=CARTESIAN_POINT('Origin',(298.461074890952,247.282959303208,530.301894951891));
#59008=CARTESIAN_POINT('',(271.071258570951,256.407969349735,522.619469351891));
#59009=CARTESIAN_POINT('',(298.461074890954,218.413116103208,522.619469351891));
#59010=CARTESIAN_POINT('Origin',(298.461074890952,247.282959303208,522.619469351891));
#59011=CARTESIAN_POINT('',(298.461074890954,218.413116103208,537.984320551892));
#59012=CARTESIAN_POINT('',(298.461074890954,218.413116103208,530.301894951892));
#59013=CARTESIAN_POINT('',(281.684561271989,270.777989356079,537.984320551891));
#59014=CARTESIAN_POINT('Origin',(298.461074890952,247.282959303208,537.984320551891));
#59015=CARTESIAN_POINT('Origin',(298.461074890952,247.282959303208,537.984320551891));
#59016=CARTESIAN_POINT('',(271.071258570952,238.157949256678,522.619469351891));
#59017=CARTESIAN_POINT('Origin',(298.461074890952,247.282959303208,522.619469351891));
#59018=CARTESIAN_POINT('',(271.071258570952,238.157949256678,536.324548179447));
#59019=CARTESIAN_POINT('',(271.071258570952,238.157949256678,536.324548179447));
#59020=CARTESIAN_POINT('',(269.591231690952,247.282959303206,536.643200551891));
#59021=CARTESIAN_POINT('Origin',(298.461074890952,247.282959303208,536.643200551891));
#59022=CARTESIAN_POINT('',(271.071258570951,256.407969349735,536.324548179447));
#59023=CARTESIAN_POINT('Origin',(298.461074890952,247.282959303208,536.643200551891));
#59024=CARTESIAN_POINT('',(271.071258570951,256.407969349735,522.619469351891));
#59025=CARTESIAN_POINT('Origin',(298.461074890952,247.282959303208,536.911424551891));
#59026=CARTESIAN_POINT('',(271.071258570952,238.214682172211,534.944448551891));
#59027=CARTESIAN_POINT('',(298.46107489095,276.134920903208,534.944448551891));
#59028=CARTESIAN_POINT('Origin',(298.461074890952,247.282959303208,534.944448551891));
#59029=CARTESIAN_POINT('',(298.46107489095,276.134920903208,538.878400551891));
#59030=CARTESIAN_POINT('',(298.46107489095,276.134920903208,536.911424551891));
#59031=CARTESIAN_POINT('Origin',(298.461074890952,247.282959303208,538.878400551891));
#59032=CARTESIAN_POINT('',(271.071258570951,256.351236434202,534.944448551891));
#59033=CARTESIAN_POINT('Origin',(298.461074890952,247.282959303208,534.944448551891));
#59034=CARTESIAN_POINT('',(271.071258570951,256.351236434202,536.326529336513));
#59035=CARTESIAN_POINT('',(271.071258570951,256.351236434202,536.326529336513));
#59036=CARTESIAN_POINT('',(269.609113290952,247.282959303206,536.643200551891));
#59037=CARTESIAN_POINT('Origin',(298.461074890952,247.282959303208,536.643200551891));
#59038=CARTESIAN_POINT('',(271.071258570952,238.214682172211,536.326529336513));
#59039=CARTESIAN_POINT('Origin',(298.461074890952,247.282959303208,536.643200551891));
#59040=CARTESIAN_POINT('',(271.071258570952,238.214682172211,534.944448551891));
#59041=CARTESIAN_POINT('Origin',(271.089140170951,251.817097868704,536.484864944202));
#59042=CARTESIAN_POINT('',(271.071258570952,247.282959303207,536.643200551891));
#59043=CARTESIAN_POINT('',(271.071258570952,247.282959303207,536.643200551891));
#59044=CARTESIAN_POINT('',(271.071258570952,247.282959303207,536.643200551891));
#59045=CARTESIAN_POINT('Origin',(271.089140170952,242.748820737708,536.484864944202));
#59046=CARTESIAN_POINT('',(271.071258570952,238.214682172211,536.326529336513));
#59047=CARTESIAN_POINT('Origin',(265.827154890955,192.583144903205,406.913912572845));
#59048=CARTESIAN_POINT('',(264.486034890955,192.565263303205,407.688208565861));
#59049=CARTESIAN_POINT('',(267.168274890955,192.565263303205,406.139616579829));
#59050=CARTESIAN_POINT('',(264.486034890955,192.565263303205,407.688208565861));
#59051=CARTESIAN_POINT('',(264.486034890955,192.118223303205,407.688208565861));
#59052=CARTESIAN_POINT('',(264.486034890955,192.565263303205,407.688208565861));
#59053=CARTESIAN_POINT('',(267.168274890955,192.118223303205,406.139616579829));
#59054=CARTESIAN_POINT('',(264.486034890955,192.118223303205,407.688208565861));
#59055=CARTESIAN_POINT('',(267.168274890955,192.565263303205,406.139616579829));
#59056=CARTESIAN_POINT('Origin',(264.486034890955,192.341743303205,407.670326965861));
#59057=CARTESIAN_POINT('',(264.486034890955,192.565263303205,410.785392537923));
#59058=CARTESIAN_POINT('',(264.486034890955,192.565263303205,410.785392537923));
#59059=CARTESIAN_POINT('',(264.486034890955,192.118223303205,410.785392537923));
#59060=CARTESIAN_POINT('',(264.486034890955,192.565263303205,410.785392537923));
#59061=CARTESIAN_POINT('',(264.486034890955,192.118223303205,410.785392537923));
#59062=CARTESIAN_POINT('Origin',(265.827154890955,192.583144903205,411.559688530939));
#59063=CARTESIAN_POINT('',(267.168274890955,192.565263303205,412.333984523954));
#59064=CARTESIAN_POINT('',(267.168274890955,192.565263303205,412.333984523954));
#59065=CARTESIAN_POINT('',(267.168274890955,192.118223303205,412.333984523954));
#59066=CARTESIAN_POINT('',(267.168274890955,192.565263303205,412.333984523954));
#59067=CARTESIAN_POINT('',(267.168274890955,192.118223303205,412.333984523954));
#59068=CARTESIAN_POINT('Origin',(329.95734926431,244.855096103656,522.619469351891));
#59069=CARTESIAN_POINT('',(271.071258570952,238.157949256678,522.619469351891));
#59070=CARTESIAN_POINT('Origin',(298.46107489095,247.282959303208,534.85504055189));
#59071=CARTESIAN_POINT('',(271.071258570952,241.675722415372,534.050368551892));
#59072=CARTESIAN_POINT('Ctrl Pts',(271.071258570952,241.675722415372,534.050368551892));
#59073=CARTESIAN_POINT('Ctrl Pts',(271.071258570952,239.972437423184,534.391979643008));
#59074=CARTESIAN_POINT('Ctrl Pts',(271.071258570952,238.214682172211,534.944448551891));
#59075=CARTESIAN_POINT('',(271.071258570951,252.89019619104,534.050368551891));
#59076=CARTESIAN_POINT('Origin',(298.461074890952,247.282959303208,534.050368551891));
#59077=CARTESIAN_POINT('Ctrl Pts',(271.071258570951,256.351236434202,534.944448551891));
#59078=CARTESIAN_POINT('Ctrl Pts',(271.071258570951,254.593481183229,534.391979643008));
#59079=CARTESIAN_POINT('Ctrl Pts',(271.071258570951,252.89019619104,534.050368551891));
#59080=CARTESIAN_POINT('Origin',(326.436838090951,247.28295930321,534.050368551891));
#59081=CARTESIAN_POINT('',(271.071258570951,252.89019619104,534.050368551891));
#59082=CARTESIAN_POINT('',(298.46107489095,269.108793223208,534.050368551891));
#59083=CARTESIAN_POINT('Origin',(298.461074890952,247.282959303208,534.050368551891));
#59084=CARTESIAN_POINT('Origin',(272.783706570949,291.986959303207,520.996800551891));
#59085=CARTESIAN_POINT('',(274.496154570948,296.695184583207,520.996800551891));
#59086=CARTESIAN_POINT('',(274.496154570949,288.155282986749,523.732790663921));
#59087=CARTESIAN_POINT('Origin',(274.496154570949,291.986959303207,520.996800551891));
#59088=CARTESIAN_POINT('Origin',(274.496154570949,291.986959303207,520.996800551891));
#59089=CARTESIAN_POINT('',(271.071258570948,296.695184583206,520.996800551891));
#59090=CARTESIAN_POINT('',(272.783706570948,296.695184583207,520.996800551891));
#59091=CARTESIAN_POINT('Origin',(271.071258570949,291.986959303206,520.996800551891));
#59092=CARTESIAN_POINT('Origin',(272.783706570948,291.986959303205,369.003200551891));
#59093=CARTESIAN_POINT('',(274.496154570948,296.695184583205,369.003200551891));
#59094=CARTESIAN_POINT('',(274.496154570949,288.155282986747,371.739190663921));
#59095=CARTESIAN_POINT('Origin',(274.496154570948,291.986959303205,369.003200551891));
#59096=CARTESIAN_POINT('Origin',(274.496154570948,291.986959303205,369.003200551891));
#59097=CARTESIAN_POINT('',(271.071258570948,296.695184583205,369.003200551891));
#59098=CARTESIAN_POINT('',(272.783706570948,296.695184583205,369.003200551891));
#59099=CARTESIAN_POINT('Origin',(271.071258570948,291.986959303205,369.003200551891));
#59100=CARTESIAN_POINT('Origin',(272.783706570954,202.578959303205,369.003200551892));
#59101=CARTESIAN_POINT('',(274.496154570954,207.287184583205,369.003200551892));
#59102=CARTESIAN_POINT('',(274.496154570955,198.747282986747,371.739190663922));
#59103=CARTESIAN_POINT('Origin',(274.496154570954,202.578959303205,369.003200551892));
#59104=CARTESIAN_POINT('Origin',(274.496154570954,202.578959303205,369.003200551892));
#59105=CARTESIAN_POINT('',(271.071258570954,207.287184583205,369.003200551892));
#59106=CARTESIAN_POINT('',(272.783706570954,207.287184583205,369.003200551892));
#59107=CARTESIAN_POINT('Origin',(271.071258570954,202.578959303205,369.003200551892));
#59108=CARTESIAN_POINT('Origin',(272.783706570955,202.578959303207,520.996800551892));
#59109=CARTESIAN_POINT('',(274.496154570954,207.287184583207,520.996800551892));
#59110=CARTESIAN_POINT('',(274.496154570955,198.747282986749,523.732790663922));
#59111=CARTESIAN_POINT('Origin',(274.496154570955,202.578959303207,520.996800551892));
#59112=CARTESIAN_POINT('Origin',(274.496154570955,202.578959303207,520.996800551892));
#59113=CARTESIAN_POINT('',(271.071258570954,207.287184583206,520.996800551892));
#59114=CARTESIAN_POINT('',(272.783706570954,207.287184583207,520.996800551892));
#59115=CARTESIAN_POINT('Origin',(271.071258570955,202.578959303206,520.996800551892));
#59116=CARTESIAN_POINT('Origin',(271.071258570952,247.282959303206,534.032486951892));
#59117=CARTESIAN_POINT('Origin',(271.08914017095,268.204431303207,535.912606650751));
#59118=CARTESIAN_POINT('',(263.413138890952,247.282959303206,536.643200551891));
#59119=CARTESIAN_POINT('',(269.591231690952,247.282959303206,536.643200551891));
#59120=CARTESIAN_POINT('',(264.053007879482,283.941029104951,535.363072546332));
#59121=CARTESIAN_POINT('',(264.053007879482,283.941029104951,535.363072546332));
#59122=CARTESIAN_POINT('',(269.329174195257,289.125903303206,535.182012749611));
#59123=CARTESIAN_POINT('',(269.329174195257,289.125903303206,535.182012749611));
#59124=CARTESIAN_POINT('',(271.071258570949,289.125903303207,535.182012749611));
#59125=CARTESIAN_POINT('',(271.071258570951,256.407969349735,536.324548179447));
#59126=CARTESIAN_POINT('Origin',(271.089140170953,226.361487303207,535.912606650752));
#59127=CARTESIAN_POINT('',(271.071258570955,205.440015303207,535.182012749612));
#59128=CARTESIAN_POINT('',(269.329174195263,205.440015303206,535.182012749612));
#59129=CARTESIAN_POINT('',(269.329174195263,205.440015303206,535.182012749612));
#59130=CARTESIAN_POINT('',(264.053007879487,210.624889501461,535.363072546333));
#59131=CARTESIAN_POINT('',(264.053007879487,210.624889501461,535.363072546333));
#59132=CARTESIAN_POINT('',(263.413138890952,247.282959303206,536.643200551891));
#59133=CARTESIAN_POINT('Origin',(271.089140170955,192.565263303205,409.236800551892));
#59134=CARTESIAN_POINT('',(271.071258570955,192.565263303205,404.844653485312));
#59135=CARTESIAN_POINT('',(263.753836065183,192.565263303205,404.454976112844));
#59136=CARTESIAN_POINT('Origin',(267.168274890955,192.565263303205,409.236800551892));
#59137=CARTESIAN_POINT('Origin',(267.168274890955,192.565263303205,409.236800551892));
#59138=CARTESIAN_POINT('',(269.850514890955,192.565263303205,407.688208565861));
#59139=CARTESIAN_POINT('',(267.168274890955,192.565263303205,406.139616579829));
#59140=CARTESIAN_POINT('',(269.850514890955,192.565263303205,410.785392537923));
#59141=CARTESIAN_POINT('',(269.850514890955,192.565263303205,407.688208565861));
#59142=CARTESIAN_POINT('',(269.850514890955,192.565263303205,410.785392537923));
#59143=CARTESIAN_POINT('Origin',(376.045474576545,162.345359303212,428.915241806248));
#59144=CARTESIAN_POINT('',(391.640751370957,162.345359303214,448.361741351892));
#59145=CARTESIAN_POINT('',(391.640751370957,162.345359303214,441.638259751892));
#59146=CARTESIAN_POINT('',(391.640751370957,162.345359303214,448.361741351892));
#59147=CARTESIAN_POINT('',(389.391142518198,162.345359303214,441.638259751892));
#59148=CARTESIAN_POINT('',(391.640751370957,162.345359303214,441.638259751892));
#59149=CARTESIAN_POINT('',(389.391142518198,162.345359303214,448.361741351892));
#59150=CARTESIAN_POINT('Origin',(375.115917770957,162.345359303213,445.000000551892));
#59151=CARTESIAN_POINT('',(389.391142518198,162.345359303214,448.361741351892));
#59152=CARTESIAN_POINT('Origin',(375.11591777096,114.845359303212,445.000000551892));
#59153=CARTESIAN_POINT('',(397.615917770963,82.3453593032132,445.000000551892));
#59154=CARTESIAN_POINT('Origin',(375.115917770963,82.3453593032118,445.000000551893));
#59155=CARTESIAN_POINT('',(397.615917770958,147.345359303214,445.000000551892));
#59156=CARTESIAN_POINT('',(397.61591777096,114.845359303213,445.000000551892));
#59157=CARTESIAN_POINT('Origin',(375.115917770958,147.345359303212,445.000000551892));
#59158=CARTESIAN_POINT('Origin',(375.115917770963,82.3453593032116,422.490000551892));
#59159=CARTESIAN_POINT('Origin',(432.504565497636,326.498447303217,494.755298322232));
#59160=CARTESIAN_POINT('',(430.89144884552,326.016308993801,491.961298322232));
#59161=CARTESIAN_POINT('',(432.09282582224,326.480565703217,494.042144284955));
#59162=CARTESIAN_POINT('Ctrl Pts',(430.891448845508,326.016308993793,491.96129832221));
#59163=CARTESIAN_POINT('Ctrl Pts',(431.532053923755,326.386162508166,493.070858865322));
#59164=CARTESIAN_POINT('Ctrl Pts',(432.092825822243,326.480565703217,494.042144284959));
#59165=CARTESIAN_POINT('',(432.916305173032,326.480565703217,495.46845235951));
#59166=CARTESIAN_POINT('',(432.09282582224,326.480565703217,494.042144284955));
#59167=CARTESIAN_POINT('',(434.117682149752,326.016308993801,497.549298322232));
#59168=CARTESIAN_POINT('Ctrl Pts',(432.916305173029,326.480565703217,495.468452359506));
#59169=CARTESIAN_POINT('Ctrl Pts',(433.477077071517,326.386162508166,496.439737779143));
#59170=CARTESIAN_POINT('Ctrl Pts',(434.117682149765,326.016308993793,497.549298322255));
#59171=CARTESIAN_POINT('',(434.117682149752,320.829980103217,497.549298322232));
#59172=CARTESIAN_POINT('',(434.117682149752,326.016308993801,497.549298322232));
#59173=CARTESIAN_POINT('',(430.891448845521,320.829980103217,491.961298322232));
#59174=CARTESIAN_POINT('',(430.891448845521,320.829980103217,491.961298322232));
#59175=CARTESIAN_POINT('',(430.89144884552,326.016308993801,491.961298322232));
#59176=CARTESIAN_POINT('Origin',(430.909330445546,323.655272903217,491.961298322232));
#59177=CARTESIAN_POINT('',(424.438982237057,326.016308993801,491.961298322232));
#59178=CARTESIAN_POINT('',(426.841736190497,326.480565703217,491.961298322232));
#59179=CARTESIAN_POINT('Ctrl Pts',(424.438982237031,326.016308993793,491.961298322232));
#59180=CARTESIAN_POINT('Ctrl Pts',(425.720192393527,326.386162508166,491.961298322232));
#59181=CARTESIAN_POINT('Ctrl Pts',(426.841736190502,326.480565703217,491.961298322232));
#59182=CARTESIAN_POINT('',(428.48869489208,326.480565703217,491.961298322232));
#59183=CARTESIAN_POINT('',(426.841736190497,326.480565703217,491.961298322232));
#59184=CARTESIAN_POINT('Ctrl Pts',(428.488694892075,326.480565703217,491.961298322232));
#59185=CARTESIAN_POINT('Ctrl Pts',(429.61023868905,326.386162508166,491.961298322232));
#59186=CARTESIAN_POINT('Ctrl Pts',(430.891448845546,326.016308993793,491.961298322232));
#59187=CARTESIAN_POINT('',(424.438982237057,320.829980103216,491.961298322232));
#59188=CARTESIAN_POINT('',(424.438982237057,320.829980103216,491.961298322232));
#59189=CARTESIAN_POINT('',(424.438982237057,326.016308993801,491.961298322232));
#59190=CARTESIAN_POINT('Origin',(422.825865584941,326.498447303216,494.755298322232));
#59191=CARTESIAN_POINT('',(421.212748932825,326.0163089938,497.549298322232));
#59192=CARTESIAN_POINT('',(422.414125909545,326.480565703216,495.46845235951));
#59193=CARTESIAN_POINT('Ctrl Pts',(421.212748932813,326.016308993792,497.549298322255));
#59194=CARTESIAN_POINT('Ctrl Pts',(421.85335401106,326.386162508165,496.439737779143));
#59195=CARTESIAN_POINT('Ctrl Pts',(422.414125909548,326.480565703216,495.468452359506));
#59196=CARTESIAN_POINT('',(423.237605260337,326.480565703216,494.042144284955));
#59197=CARTESIAN_POINT('',(422.414125909545,326.480565703216,495.46845235951));
#59198=CARTESIAN_POINT('Ctrl Pts',(423.237605260335,326.480565703216,494.042144284959));
#59199=CARTESIAN_POINT('Ctrl Pts',(423.798377158822,326.386162508166,493.070858865322));
#59200=CARTESIAN_POINT('Ctrl Pts',(424.43898223707,326.016308993793,491.96129832221));
#59201=CARTESIAN_POINT('',(421.212748932826,320.829980103216,497.549298322232));
#59202=CARTESIAN_POINT('',(421.212748932826,320.829980103216,497.549298322232));
#59203=CARTESIAN_POINT('',(421.212748932825,326.0163089938,497.549298322232));
#59204=CARTESIAN_POINT('Origin',(422.825865584941,326.498447303216,500.343298322232));
#59205=CARTESIAN_POINT('',(424.438982237057,326.016308993801,503.137298322232));
#59206=CARTESIAN_POINT('',(423.237605260337,326.480565703217,501.05645235951));
#59207=CARTESIAN_POINT('Ctrl Pts',(424.43898223707,326.016308993793,503.137298322254));
#59208=CARTESIAN_POINT('Ctrl Pts',(423.798377158822,326.386162508166,502.027737779143));
#59209=CARTESIAN_POINT('Ctrl Pts',(423.237605260335,326.480565703217,501.056452359506));
#59210=CARTESIAN_POINT('',(422.414125909545,326.480565703216,499.630144284955));
#59211=CARTESIAN_POINT('',(423.237605260337,326.480565703217,501.05645235951));
#59212=CARTESIAN_POINT('Ctrl Pts',(422.414125909548,326.480565703216,499.630144284959));
#59213=CARTESIAN_POINT('Ctrl Pts',(421.85335401106,326.386162508165,498.658858865322));
#59214=CARTESIAN_POINT('Ctrl Pts',(421.212748932813,326.016308993792,497.54929832221));
#59215=CARTESIAN_POINT('',(424.438982237057,320.829980103216,503.137298322232));
#59216=CARTESIAN_POINT('',(424.438982237057,320.829980103216,503.137298322232));
#59217=CARTESIAN_POINT('',(424.438982237057,326.016308993801,503.137298322232));
#59218=CARTESIAN_POINT('Origin',(427.665215541289,326.062734664735,497.549298322232));
#59219=CARTESIAN_POINT('',(426.841736190497,326.480565703217,503.137298322232));
#59220=CARTESIAN_POINT('Ctrl Pts',(426.841736190502,326.480565703217,503.137298322232));
#59221=CARTESIAN_POINT('Ctrl Pts',(425.720192393527,326.386162508166,503.137298322232));
#59222=CARTESIAN_POINT('Ctrl Pts',(424.438982237031,326.016308993793,503.137298322232));
#59223=CARTESIAN_POINT('Origin',(427.665215541289,326.480565703217,497.549298322233));
#59224=CARTESIAN_POINT('Origin',(427.665215541288,326.062734664736,497.549298322232));
#59225=CARTESIAN_POINT('Origin',(427.665215541289,326.480565703217,497.549298322232));
#59226=CARTESIAN_POINT('Origin',(427.665215541288,326.062734664735,497.549298322232));
#59227=CARTESIAN_POINT('',(430.89144884552,326.016308993801,503.137298322232));
#59228=CARTESIAN_POINT('',(428.48869489208,326.480565703217,503.137298322232));
#59229=CARTESIAN_POINT('Ctrl Pts',(430.891448845546,326.016308993793,503.137298322232));
#59230=CARTESIAN_POINT('Ctrl Pts',(429.61023868905,326.386162508166,503.137298322232));
#59231=CARTESIAN_POINT('Ctrl Pts',(428.488694892075,326.480565703217,503.137298322232));
#59232=CARTESIAN_POINT('',(432.09282582224,326.480565703217,501.05645235951));
#59233=CARTESIAN_POINT('Ctrl Pts',(432.092825822243,326.480565703217,501.056452359506));
#59234=CARTESIAN_POINT('Ctrl Pts',(431.532053923755,326.386162508166,502.027737779143));
#59235=CARTESIAN_POINT('Ctrl Pts',(430.891448845508,326.016308993793,503.137298322254));
#59236=CARTESIAN_POINT('Origin',(427.665215541289,326.480565703217,497.549298322233));
#59237=CARTESIAN_POINT('Origin',(427.66521554129,326.062734664736,497.549298322232));
#59238=CARTESIAN_POINT('',(432.916305173032,326.480565703217,499.630144284955));
#59239=CARTESIAN_POINT('Ctrl Pts',(434.117682149765,326.016308993793,497.54929832221));
#59240=CARTESIAN_POINT('Ctrl Pts',(433.477077071517,326.386162508166,498.658858865322));
#59241=CARTESIAN_POINT('Ctrl Pts',(432.916305173029,326.480565703217,499.630144284959));
#59242=CARTESIAN_POINT('Origin',(427.665215541289,326.480565703217,497.549298322232));
#59243=CARTESIAN_POINT('Origin',(427.66521554129,326.062734664736,497.549298322231));
#59244=CARTESIAN_POINT('Origin',(427.665215541289,326.480565703217,497.549298322232));
#59245=CARTESIAN_POINT('Origin',(432.504565497636,326.498447303217,500.343298322232));
#59246=CARTESIAN_POINT('',(432.916305173032,326.480565703217,499.630144284955));
#59247=CARTESIAN_POINT('',(430.891448845521,320.829980103217,503.137298322232));
#59248=CARTESIAN_POINT('',(430.89144884552,326.016308993801,503.137298322232));
#59249=CARTESIAN_POINT('',(434.117682149752,320.829980103217,497.549298322232));
#59250=CARTESIAN_POINT('Origin',(430.909330445546,323.655272903217,503.137298322232));
#59251=CARTESIAN_POINT('',(428.48869489208,326.480565703217,503.137298322232));
#59252=CARTESIAN_POINT('',(430.891448845521,320.829980103217,503.137298322232));
#59253=CARTESIAN_POINT('Origin',(427.665215541289,326.062734664735,497.549298322233));
#59254=CARTESIAN_POINT('Origin',(427.665215541288,326.480565703217,497.549298322232));
#59255=CARTESIAN_POINT('Origin',(433.758762284827,326.480565703217,497.549298322232));
#59256=CARTESIAN_POINT('Origin',(327.405969956951,326.498447303209,389.656702781548));
#59257=CARTESIAN_POINT('',(325.792853304836,326.016308993793,386.862702781548));
#59258=CARTESIAN_POINT('',(326.994230281556,326.480565703209,388.943548744271));
#59259=CARTESIAN_POINT('Ctrl Pts',(325.792853304823,326.016308993785,386.862702781526));
#59260=CARTESIAN_POINT('Ctrl Pts',(326.433458383071,326.386162508158,387.972263324638));
#59261=CARTESIAN_POINT('Ctrl Pts',(326.994230281558,326.480565703209,388.943548744275));
#59262=CARTESIAN_POINT('',(327.817709632347,326.480565703209,390.369856818826));
#59263=CARTESIAN_POINT('',(326.994230281556,326.480565703209,388.943548744271));
#59264=CARTESIAN_POINT('',(329.019086609067,326.016308993793,392.450702781548));
#59265=CARTESIAN_POINT('Ctrl Pts',(327.817709632345,326.480565703209,390.369856818822));
#59266=CARTESIAN_POINT('Ctrl Pts',(328.378481530832,326.386162508158,391.341142238459));
#59267=CARTESIAN_POINT('Ctrl Pts',(329.01908660908,326.016308993785,392.450702781571));
#59268=CARTESIAN_POINT('',(329.019086609068,320.829980103209,392.450702781549));
#59269=CARTESIAN_POINT('',(329.019086609067,326.016308993792,392.450702781548));
#59270=CARTESIAN_POINT('',(325.792853304836,320.829980103209,386.862702781548));
#59271=CARTESIAN_POINT('',(325.792853304836,320.829980103209,386.862702781548));
#59272=CARTESIAN_POINT('',(325.792853304836,326.016308993792,386.862702781548));
#59273=CARTESIAN_POINT('Origin',(325.810734904861,323.655272903209,386.862702781548));
#59274=CARTESIAN_POINT('',(319.340386696372,326.016308993792,386.862702781548));
#59275=CARTESIAN_POINT('',(321.743140649812,326.480565703209,386.862702781548));
#59276=CARTESIAN_POINT('Ctrl Pts',(319.340386696347,326.016308993784,386.862702781548));
#59277=CARTESIAN_POINT('Ctrl Pts',(320.621596852842,326.386162508158,386.862702781548));
#59278=CARTESIAN_POINT('Ctrl Pts',(321.743140649817,326.480565703209,386.862702781548));
#59279=CARTESIAN_POINT('',(323.390099351396,326.480565703209,386.862702781548));
#59280=CARTESIAN_POINT('',(321.743140649812,326.480565703209,386.862702781548));
#59281=CARTESIAN_POINT('Ctrl Pts',(323.390099351391,326.480565703209,386.862702781548));
#59282=CARTESIAN_POINT('Ctrl Pts',(324.511643148366,326.386162508158,386.862702781548));
#59283=CARTESIAN_POINT('Ctrl Pts',(325.792853304861,326.016308993785,386.862702781548));
#59284=CARTESIAN_POINT('',(319.340386696372,320.829980103208,386.862702781548));
#59285=CARTESIAN_POINT('',(319.340386696372,320.829980103208,386.862702781548));
#59286=CARTESIAN_POINT('',(319.340386696372,326.016308993792,386.862702781548));
#59287=CARTESIAN_POINT('Origin',(317.727270044256,326.498447303208,389.656702781548));
#59288=CARTESIAN_POINT('',(316.114153392141,326.016308993792,392.450702781548));
#59289=CARTESIAN_POINT('',(317.315530368861,326.480565703208,390.369856818826));
#59290=CARTESIAN_POINT('Ctrl Pts',(316.114153392128,326.016308993784,392.450702781571));
#59291=CARTESIAN_POINT('Ctrl Pts',(316.754758470376,326.386162508157,391.341142238459));
#59292=CARTESIAN_POINT('Ctrl Pts',(317.315530368863,326.480565703209,390.369856818822));
#59293=CARTESIAN_POINT('',(318.139009719652,326.480565703208,388.943548744271));
#59294=CARTESIAN_POINT('',(317.315530368861,326.480565703208,390.369856818826));
#59295=CARTESIAN_POINT('Ctrl Pts',(318.13900971965,326.480565703209,388.943548744275));
#59296=CARTESIAN_POINT('Ctrl Pts',(318.699781618137,326.386162508157,387.972263324638));
#59297=CARTESIAN_POINT('Ctrl Pts',(319.340386696385,326.016308993784,386.862702781526));
#59298=CARTESIAN_POINT('',(316.114153392141,320.829980103208,392.450702781549));
#59299=CARTESIAN_POINT('',(316.114153392141,320.829980103208,392.450702781549));
#59300=CARTESIAN_POINT('',(316.114153392141,326.016308993791,392.450702781548));
#59301=CARTESIAN_POINT('Origin',(317.727270044256,326.498447303209,395.244702781548));
#59302=CARTESIAN_POINT('',(319.340386696372,326.016308993792,398.038702781548));
#59303=CARTESIAN_POINT('',(318.139009719652,326.480565703209,395.957856818826));
#59304=CARTESIAN_POINT('Ctrl Pts',(319.340386696385,326.016308993785,398.038702781571));
#59305=CARTESIAN_POINT('Ctrl Pts',(318.699781618137,326.386162508158,396.929142238459));
#59306=CARTESIAN_POINT('Ctrl Pts',(318.13900971965,326.480565703209,395.957856818822));
#59307=CARTESIAN_POINT('',(317.315530368861,326.480565703208,394.531548744271));
#59308=CARTESIAN_POINT('',(318.139009719652,326.480565703209,395.957856818826));
#59309=CARTESIAN_POINT('Ctrl Pts',(317.315530368863,326.480565703209,394.531548744275));
#59310=CARTESIAN_POINT('Ctrl Pts',(316.754758470376,326.386162508157,393.560263324638));
#59311=CARTESIAN_POINT('Ctrl Pts',(316.114153392128,326.016308993784,392.450702781526));
#59312=CARTESIAN_POINT('',(319.340386696372,320.829980103208,398.038702781548));
#59313=CARTESIAN_POINT('',(319.340386696372,320.829980103208,398.038702781548));
#59314=CARTESIAN_POINT('',(319.340386696372,326.016308993792,398.038702781548));
#59315=CARTESIAN_POINT('Origin',(322.566620000605,326.06273466473,392.450702781554));
#59316=CARTESIAN_POINT('',(321.743140649812,326.480565703209,398.038702781548));
#59317=CARTESIAN_POINT('Ctrl Pts',(321.743140649817,326.480565703209,398.038702781548));
#59318=CARTESIAN_POINT('Ctrl Pts',(320.621596852842,326.386162508158,398.038702781548));
#59319=CARTESIAN_POINT('Ctrl Pts',(319.340386696347,326.016308993785,398.038702781549));
#59320=CARTESIAN_POINT('Origin',(322.566620000605,326.480565703209,392.450702781546));
#59321=CARTESIAN_POINT('Origin',(322.5666200006,326.062734664731,392.450702781548));
#59322=CARTESIAN_POINT('Origin',(322.566620000601,326.480565703209,392.450702781548));
#59323=CARTESIAN_POINT('Origin',(322.566620000602,326.062734664725,392.450702781546));
#59324=CARTESIAN_POINT('',(325.792853304836,326.016308993793,398.038702781548));
#59325=CARTESIAN_POINT('',(323.390099351396,326.480565703209,398.038702781548));
#59326=CARTESIAN_POINT('Ctrl Pts',(325.792853304861,326.016308993785,398.038702781548));
#59327=CARTESIAN_POINT('Ctrl Pts',(324.511643148366,326.386162508158,398.038702781548));
#59328=CARTESIAN_POINT('Ctrl Pts',(323.390099351391,326.480565703209,398.038702781548));
#59329=CARTESIAN_POINT('',(326.994230281556,326.480565703209,395.957856818826));
#59330=CARTESIAN_POINT('Ctrl Pts',(326.994230281558,326.480565703209,395.957856818822));
#59331=CARTESIAN_POINT('Ctrl Pts',(326.433458383071,326.386162508158,396.929142238459));
#59332=CARTESIAN_POINT('Ctrl Pts',(325.792853304823,326.016308993785,398.03870278157));
#59333=CARTESIAN_POINT('Origin',(322.566620000604,326.480565703209,392.450702781548));
#59334=CARTESIAN_POINT('Origin',(322.566620000608,326.06273466473,392.450702781548));
#59335=CARTESIAN_POINT('',(327.817709632347,326.480565703209,394.531548744271));
#59336=CARTESIAN_POINT('Ctrl Pts',(329.01908660908,326.016308993785,392.450702781526));
#59337=CARTESIAN_POINT('Ctrl Pts',(328.378481530832,326.386162508158,393.560263324638));
#59338=CARTESIAN_POINT('Ctrl Pts',(327.817709632345,326.480565703209,394.531548744275));
#59339=CARTESIAN_POINT('Origin',(322.566620000604,326.480565703209,392.450702781548));
#59340=CARTESIAN_POINT('Origin',(322.566620000604,326.062734664727,392.450702781548));
#59341=CARTESIAN_POINT('Origin',(322.566620000604,326.480565703209,392.450702781549));
#59342=CARTESIAN_POINT('Origin',(327.405969956951,326.498447303209,395.244702781548));
#59343=CARTESIAN_POINT('',(327.817709632347,326.480565703209,394.531548744271));
#59344=CARTESIAN_POINT('',(325.792853304836,320.829980103209,398.038702781548));
#59345=CARTESIAN_POINT('',(325.792853304836,326.016308993792,398.038702781548));
#59346=CARTESIAN_POINT('',(329.019086609068,320.829980103209,392.450702781549));
#59347=CARTESIAN_POINT('Origin',(325.810734904861,323.655272903209,398.038702781548));
#59348=CARTESIAN_POINT('',(323.390099351396,326.480565703209,398.038702781548));
#59349=CARTESIAN_POINT('',(325.792853304836,320.829980103209,398.038702781548));
#59350=CARTESIAN_POINT('Origin',(322.56662000061,326.062734664723,392.450702781552));
#59351=CARTESIAN_POINT('Origin',(322.566620000605,326.480565703209,392.450702781551));
#59352=CARTESIAN_POINT('Origin',(328.660166744143,326.480565703209,392.450702781548));
#59353=CARTESIAN_POINT('Origin',(313.603213770955,192.583144903208,383.487296551892));
#59354=CARTESIAN_POINT('',(303.589517770956,173.610767303207,393.500992551892));
#59355=CARTESIAN_POINT('',(303.589517770956,173.610767303207,393.500992551892));
#59356=CARTESIAN_POINT('',(303.589517770956,173.610767303207,393.500992551892));
#59357=CARTESIAN_POINT('Origin',(303.589517770947,311.415317703207,393.483110951891));
#59358=CARTESIAN_POINT('',(303.589517770946,320.829980103207,393.500992551891));
#59359=CARTESIAN_POINT('',(303.589517770948,302.000655303207,393.500992551891));
#59360=CARTESIAN_POINT('',(303.589517770947,320.829980103208,496.499008551891));
#59361=CARTESIAN_POINT('',(303.589517770948,302.000655303208,496.499008551891));
#59362=CARTESIAN_POINT('',(303.589517770947,320.829980103208,496.499008551891));
#59363=CARTESIAN_POINT('Origin',(313.603213770947,320.847861703209,506.512704551891));
#59364=CARTESIAN_POINT('',(323.616909770947,320.82998010321,516.526400551891));
#59365=CARTESIAN_POINT('',(323.616909770948,302.000655303209,516.526400551891));
#59366=CARTESIAN_POINT('',(323.616909770947,320.82998010321,516.526400551891));
#59367=CARTESIAN_POINT('Origin',(426.632807370947,311.415317703216,516.52640055189));
#59368=CARTESIAN_POINT('',(426.614925770947,320.829980103217,516.52640055189));
#59369=CARTESIAN_POINT('',(426.614925770948,302.000655303216,516.52640055189));
#59370=CARTESIAN_POINT('',(426.614925770947,320.829980103217,516.52640055189));
#59371=CARTESIAN_POINT('Origin',(436.628621770947,320.847861703217,506.51270455189));
#59372=CARTESIAN_POINT('',(446.642317770947,320.829980103218,496.49900855189));
#59373=CARTESIAN_POINT('',(446.642317770948,302.000655303218,496.49900855189));
#59374=CARTESIAN_POINT('',(446.642317770947,320.829980103218,496.49900855189));
#59375=CARTESIAN_POINT('Origin',(446.642317770947,311.415317703217,393.48311095189));
#59376=CARTESIAN_POINT('',(446.642317770946,320.829980103217,393.50099255189));
#59377=CARTESIAN_POINT('',(446.642317770948,302.000655303217,393.50099255189));
#59378=CARTESIAN_POINT('',(446.642317770946,320.829980103217,393.50099255189));
#59379=CARTESIAN_POINT('Origin',(436.628621770946,320.847861703216,383.48729655189));
#59380=CARTESIAN_POINT('',(426.614925770946,320.829980103215,373.47360055189));
#59381=CARTESIAN_POINT('Origin',(310.328942513349,206.648052988296,345.154828979381));
#59382=CARTESIAN_POINT('Origin',(317.611309698626,207.368333416955,344.408956761074));
#59383=CARTESIAN_POINT('',(271.071258570953,220.730842673381,330.571673357734));
#59384=CARTESIAN_POINT('Origin',(310.328942513343,287.917865618119,345.15482897938));
#59385=CARTESIAN_POINT('',(271.071258570948,302.000655303205,359.737984601026));
#59386=CARTESIAN_POINT('Origin',(317.611309698621,287.197585189461,344.408956761074));
#59387=CARTESIAN_POINT('Origin',(317.611309698618,288.694127375538,335.477394119331));
#59388=CARTESIAN_POINT('Origin',(442.171917770952,250.859279303218,536.344095603207));
#59389=CARTESIAN_POINT('Origin',(442.171917770952,250.859279303218,536.643200551891));
#59390=CARTESIAN_POINT('Origin',(363.850509770952,243.706639303217,536.577811187259));
#59391=CARTESIAN_POINT('Origin',(363.850509770952,243.706639303213,536.643200551891));
#59392=CARTESIAN_POINT('Origin',(444.872039370952,250.859279303218,534.855040551891));
#59393=CARTESIAN_POINT('',(439.489677770952,252.407871289249,534.855040551891));
#59394=CARTESIAN_POINT('',(439.489677770952,249.310687317187,534.855040551891));
#59395=CARTESIAN_POINT('',(439.489677770952,252.407871289249,534.855040551891));
#59396=CARTESIAN_POINT('',(442.171917770952,247.762095331156,534.855040551891));
#59397=CARTESIAN_POINT('',(439.489677770952,249.310687317187,534.855040551891));
#59398=CARTESIAN_POINT('',(444.854157770952,249.310687317187,534.855040551891));
#59399=CARTESIAN_POINT('',(442.171917770952,247.762095331156,534.855040551891));
#59400=CARTESIAN_POINT('',(444.854157770951,252.407871289249,534.855040551891));
#59401=CARTESIAN_POINT('',(444.854157770952,249.310687317187,534.855040551891));
#59402=CARTESIAN_POINT('',(442.171917770951,253.95646327528,534.855040551891));
#59403=CARTESIAN_POINT('',(444.854157770951,252.407871289249,534.855040551891));
#59404=CARTESIAN_POINT('',(442.171917770951,253.95646327528,534.855040551891));
#59405=CARTESIAN_POINT('Origin',(440.830797770951,253.182167282265,534.837158951891));
#59406=CARTESIAN_POINT('',(442.171917770951,253.95646327528,536.643200551891));
#59407=CARTESIAN_POINT('',(439.489677770952,252.407871289249,536.643200551891));
#59408=CARTESIAN_POINT('',(442.171917770951,253.95646327528,536.643200551891));
#59409=CARTESIAN_POINT('',(439.489677770952,252.407871289249,534.855040551891));
#59410=CARTESIAN_POINT('',(442.171917770951,253.95646327528,534.855040551891));
#59411=CARTESIAN_POINT('Origin',(443.513037770951,253.182167282265,534.837158951891));
#59412=CARTESIAN_POINT('',(444.854157770951,252.407871289249,536.643200551891));
#59413=CARTESIAN_POINT('',(444.854157770951,252.407871289249,536.643200551891));
#59414=CARTESIAN_POINT('',(444.854157770951,252.407871289249,534.855040551891));
#59415=CARTESIAN_POINT('Origin',(444.854157770952,250.859279303218,534.837158951891));
#59416=CARTESIAN_POINT('',(444.854157770952,249.310687317187,536.643200551891));
#59417=CARTESIAN_POINT('',(444.854157770952,249.310687317187,534.855040551891));
#59418=CARTESIAN_POINT('',(444.854157770951,252.407871289249,536.643200551891));
#59419=CARTESIAN_POINT('Origin',(443.513037770952,248.536391324171,534.837158951891));
#59420=CARTESIAN_POINT('',(442.171917770952,247.762095331156,536.643200551891));
#59421=CARTESIAN_POINT('',(442.171917770952,247.762095331156,536.643200551891));
#59422=CARTESIAN_POINT('',(442.171917770952,247.762095331156,534.855040551891));
#59423=CARTESIAN_POINT('Origin',(440.830797770952,248.536391324171,534.837158951891));
#59424=CARTESIAN_POINT('',(439.489677770952,249.310687317187,536.643200551891));
#59425=CARTESIAN_POINT('',(439.489677770952,249.310687317187,536.643200551891));
#59426=CARTESIAN_POINT('',(439.489677770952,249.310687317187,534.855040551891));
#59427=CARTESIAN_POINT('Origin',(439.489677770952,250.859279303218,534.837158951891));
#59428=CARTESIAN_POINT('',(439.489677770952,252.407871289249,536.643200551891));
#59429=CARTESIAN_POINT('Origin',(442.17191777095,250.859279303222,536.577811187251));
#59430=CARTESIAN_POINT('Origin',(442.171917770952,250.859279303218,536.643200551891));
#59431=CARTESIAN_POINT('Origin',(449.455947285591,251.903964171691,536.643200551891));
#59432=CARTESIAN_POINT('Origin',(366.550631370952,243.706639303213,534.855040551891));
#59433=CARTESIAN_POINT('',(361.168269770952,245.255231289244,534.855040551891));
#59434=CARTESIAN_POINT('',(361.168269770952,242.158047317181,534.855040551891));
#59435=CARTESIAN_POINT('',(361.168269770952,245.255231289244,534.855040551891));
#59436=CARTESIAN_POINT('',(363.850509770952,240.60945533115,534.855040551891));
#59437=CARTESIAN_POINT('',(361.168269770952,242.158047317181,534.855040551891));
#59438=CARTESIAN_POINT('',(366.532749770952,242.158047317182,534.855040551891));
#59439=CARTESIAN_POINT('',(363.850509770952,240.60945533115,534.855040551891));
#59440=CARTESIAN_POINT('',(366.532749770952,245.255231289244,534.855040551891));
#59441=CARTESIAN_POINT('',(366.532749770952,242.158047317182,534.855040551891));
#59442=CARTESIAN_POINT('',(363.850509770952,246.803823275275,534.855040551891));
#59443=CARTESIAN_POINT('',(366.532749770952,245.255231289244,534.855040551891));
#59444=CARTESIAN_POINT('',(363.850509770952,246.803823275275,534.855040551891));
#59445=CARTESIAN_POINT('Origin',(362.509389770952,246.029527282259,534.837158951891));
#59446=CARTESIAN_POINT('',(363.850509770952,246.803823275275,536.643200551891));
#59447=CARTESIAN_POINT('',(361.168269770952,245.255231289244,536.643200551891));
#59448=CARTESIAN_POINT('',(363.850509770952,246.803823275275,536.643200551891));
#59449=CARTESIAN_POINT('',(361.168269770952,245.255231289244,534.855040551891));
#59450=CARTESIAN_POINT('',(363.850509770952,246.803823275275,534.855040551891));
#59451=CARTESIAN_POINT('Origin',(365.191629770952,246.02952728226,534.837158951891));
#59452=CARTESIAN_POINT('',(366.532749770952,245.255231289244,536.643200551891));
#59453=CARTESIAN_POINT('',(366.532749770952,245.255231289244,536.643200551891));
#59454=CARTESIAN_POINT('',(366.532749770952,245.255231289244,534.855040551891));
#59455=CARTESIAN_POINT('Origin',(366.532749770952,243.706639303213,534.837158951891));
#59456=CARTESIAN_POINT('',(366.532749770952,242.158047317182,536.643200551891));
#59457=CARTESIAN_POINT('',(366.532749770952,242.158047317182,534.855040551891));
#59458=CARTESIAN_POINT('',(366.532749770952,245.255231289244,536.643200551891));
#59459=CARTESIAN_POINT('Origin',(365.191629770952,241.383751324166,534.837158951891));
#59460=CARTESIAN_POINT('',(363.850509770952,240.60945533115,536.643200551891));
#59461=CARTESIAN_POINT('',(363.850509770952,240.60945533115,536.643200551891));
#59462=CARTESIAN_POINT('',(363.850509770952,240.60945533115,534.855040551891));
#59463=CARTESIAN_POINT('Origin',(362.509389770952,241.383751324166,534.837158951891));
#59464=CARTESIAN_POINT('',(361.168269770952,242.158047317181,536.643200551891));
#59465=CARTESIAN_POINT('',(361.168269770952,242.158047317181,536.643200551891));
#59466=CARTESIAN_POINT('',(361.168269770952,242.158047317181,534.855040551891));
#59467=CARTESIAN_POINT('Origin',(361.168269770952,243.706639303213,534.837158951891));
#59468=CARTESIAN_POINT('',(361.168269770952,245.255231289244,536.643200551891));
#59469=CARTESIAN_POINT('Origin',(363.850509770952,243.706639303213,536.344095603207));
#59470=CARTESIAN_POINT('Origin',(363.850509770952,243.706639303213,536.643200551891));
#59471=CARTESIAN_POINT('Origin',(371.134539285592,242.661954434742,536.643200551891));
#59472=CARTESIAN_POINT('Origin',(268.509394890955,192.583144903205,411.559688530939));
#59473=CARTESIAN_POINT('',(269.850514890955,192.118223303205,410.785392537923));
#59474=CARTESIAN_POINT('',(269.850514890955,192.565263303205,410.785392537923));
#59475=CARTESIAN_POINT('',(269.850514890955,192.118223303205,410.785392537923));
#59476=CARTESIAN_POINT('Origin',(269.850514890955,192.341743303205,407.670326965861));
#59477=CARTESIAN_POINT('',(269.850514890955,192.118223303205,407.688208565861));
#59478=CARTESIAN_POINT('',(269.850514890955,192.565263303205,407.688208565861));
#59479=CARTESIAN_POINT('',(269.850514890955,192.118223303205,410.785392537923));
#59480=CARTESIAN_POINT('Origin',(268.509394890955,192.583144903205,406.913912572845));
#59481=CARTESIAN_POINT('',(267.168274890955,192.118223303205,406.139616579829));
#59482=CARTESIAN_POINT('Origin',(272.628588001728,192.118223303206,409.236800551892));
#59483=CARTESIAN_POINT('',(264.005631237915,192.118223303203,404.807608089002));
#59484=CARTESIAN_POINT('Origin',(267.168274890955,192.118223303205,409.236800551892));
#59485=CARTESIAN_POINT('Origin',(267.168274890955,192.520559303204,409.236800551893));
#59486=CARTESIAN_POINT('',(263.779015582457,192.520559303203,404.490239310461));
#59487=CARTESIAN_POINT('Origin',(277.22667489095,274.105359303207,519.569153599969));
#59488=CARTESIAN_POINT('',(277.22667489095,274.105359303207,519.410526160866));
#59489=CARTESIAN_POINT('',(275.630074508445,276.341352717653,520.996800551891));
#59490=CARTESIAN_POINT('',(277.067014852699,274.328958644651,519.569153599969));
#59491=CARTESIAN_POINT('',(277.22667489095,271.357851463207,520.996800551891));
#59492=CARTESIAN_POINT('Origin',(277.22667489095,274.105359303207,520.996800551891));
#59493=CARTESIAN_POINT('Origin',(277.22667489095,274.105359303207,520.996800551891));
#59494=CARTESIAN_POINT('Origin',(277.22667489095,274.105359303207,529.634954471891));
#59495=CARTESIAN_POINT('',(277.22667489095,271.357851463207,538.273108391891));
#59496=CARTESIAN_POINT('',(277.22667489095,271.357851463207,529.634954471891));
#59497=CARTESIAN_POINT('',(275.630074508445,276.341352717653,538.273108391891));
#59498=CARTESIAN_POINT('Origin',(277.22667489095,274.105359303207,538.273108391891));
#59499=CARTESIAN_POINT('Origin',(277.22667489095,274.105359303207,538.273108391891));
#59500=CARTESIAN_POINT('Origin',(277.22667489095,274.105359303207,538.333637607891));
#59501=CARTESIAN_POINT('',(275.278334040188,276.833955236879,538.878400551891));
#59502=CARTESIAN_POINT('',(275.594900461619,276.390612969576,538.333637607891));
#59503=CARTESIAN_POINT('Origin',(277.22667489095,274.105359303207,538.878400551891));
#59504=CARTESIAN_POINT('Origin',(319.695474890954,220.46055930321,519.569153599969));
#59505=CARTESIAN_POINT('',(319.695474890954,220.46055930321,519.410526160867));
#59506=CARTESIAN_POINT('',(318.098874508449,222.696552717656,520.996800551892));
#59507=CARTESIAN_POINT('',(319.535814852703,220.684158644654,519.569153599969));
#59508=CARTESIAN_POINT('',(319.695474890954,217.71305146321,520.996800551892));
#59509=CARTESIAN_POINT('Origin',(319.695474890954,220.46055930321,520.996800551892));
#59510=CARTESIAN_POINT('Origin',(319.695474890954,220.46055930321,520.996800551892));
#59511=CARTESIAN_POINT('Origin',(319.695474890954,220.46055930321,529.634954471891));
#59512=CARTESIAN_POINT('',(319.695474890954,217.71305146321,538.273108391892));
#59513=CARTESIAN_POINT('',(319.695474890954,217.71305146321,529.634954471891));
#59514=CARTESIAN_POINT('',(318.098874508449,222.696552717656,538.273108391891));
#59515=CARTESIAN_POINT('Origin',(319.695474890954,220.46055930321,538.273108391891));
#59516=CARTESIAN_POINT('Origin',(319.695474890954,220.46055930321,538.273108391891));
#59517=CARTESIAN_POINT('Origin',(319.695474890954,220.46055930321,538.333637607891));
#59518=CARTESIAN_POINT('',(317.747134040191,223.189155236882,538.878400551892));
#59519=CARTESIAN_POINT('',(318.063700461623,222.745812969579,538.333637607891));
#59520=CARTESIAN_POINT('Origin',(319.695474890954,220.46055930321,538.878400551891));
#59521=CARTESIAN_POINT('Origin',(277.226674890954,220.460559303207,519.569153599969));
#59522=CARTESIAN_POINT('',(277.226674890954,220.460559303207,519.410526160867));
#59523=CARTESIAN_POINT('',(275.630074508449,222.696552717653,520.996800551892));
#59524=CARTESIAN_POINT('',(277.067014852703,220.684158644651,519.569153599969));
#59525=CARTESIAN_POINT('',(277.226674890954,217.713051463207,520.996800551892));
#59526=CARTESIAN_POINT('Origin',(277.226674890954,220.460559303207,520.996800551892));
#59527=CARTESIAN_POINT('Origin',(277.226674890954,220.460559303207,520.996800551892));
#59528=CARTESIAN_POINT('Origin',(277.226674890954,220.460559303207,529.634954471892));
#59529=CARTESIAN_POINT('',(277.226674890954,217.713051463207,538.273108391892));
#59530=CARTESIAN_POINT('',(277.226674890954,217.713051463207,529.634954471892));
#59531=CARTESIAN_POINT('',(275.630074508449,222.696552717653,538.273108391892));
#59532=CARTESIAN_POINT('Origin',(277.226674890954,220.460559303207,538.273108391892));
#59533=CARTESIAN_POINT('Origin',(277.226674890954,220.460559303207,538.273108391892));
#59534=CARTESIAN_POINT('Origin',(277.226674890954,220.460559303207,538.333637607892));
#59535=CARTESIAN_POINT('',(275.278334040191,223.189155236879,538.878400551892));
#59536=CARTESIAN_POINT('',(275.594900461623,222.745812969576,538.333637607892));
#59537=CARTESIAN_POINT('Origin',(277.226674890954,220.460559303207,538.878400551892));
#59538=CARTESIAN_POINT('Origin',(322.566620000615,174.23277875921,497.549298322234));
#59539=CARTESIAN_POINT('',(322.566620000615,174.30189114321,500.769774482234));
#59540=CARTESIAN_POINT('',(320.695173668762,174.30189114321,500.170205669723));
#59541=CARTESIAN_POINT('Origin',(322.566620000615,174.30189114321,497.549298322234));
#59542=CARTESIAN_POINT('Origin',(322.566620000615,174.30189114321,497.549298322234));
#59543=CARTESIAN_POINT('',(320.293555674725,173.610767303209,500.732660244851));
#59544=CARTESIAN_POINT('',(320.655011869359,174.23277875921,500.226451127236));
#59545=CARTESIAN_POINT('Origin',(322.566620000615,173.61076730321,497.549298322234));
#59546=CARTESIAN_POINT('Origin',(322.566620000614,184.59588122321,497.549298322234));
#59547=CARTESIAN_POINT('',(322.566620000613,194.88987130321,500.769774482234));
#59548=CARTESIAN_POINT('',(322.566620000614,184.59588122321,500.769774482234));
#59549=CARTESIAN_POINT('',(320.69517366876,194.889871303211,500.170205669724));
#59550=CARTESIAN_POINT('Origin',(322.566620000613,194.88987130321,497.549298322234));
#59551=CARTESIAN_POINT('Origin',(322.566620000613,194.88987130321,497.549298322234));
#59552=CARTESIAN_POINT('Origin',(322.566620000613,196.563279803317,497.549298322234));
#59553=CARTESIAN_POINT('',(322.566620000613,196.749214081107,497.549298322234));
#59554=CARTESIAN_POINT('',(322.379475367428,196.563279803317,497.811389056983));
#59555=CARTESIAN_POINT('Origin',(427.665215541298,174.232778759216,392.450702781549));
#59556=CARTESIAN_POINT('',(427.665215541298,174.301891143216,395.671178941549));
#59557=CARTESIAN_POINT('',(425.793769209446,174.301891143216,395.071610129039));
#59558=CARTESIAN_POINT('Origin',(427.665215541298,174.301891143216,392.450702781549));
#59559=CARTESIAN_POINT('Origin',(427.665215541298,174.301891143216,392.450702781549));
#59560=CARTESIAN_POINT('',(425.392151215409,173.610767303216,395.634064704167));
#59561=CARTESIAN_POINT('',(425.753607410043,174.232778759216,395.127855586552));
#59562=CARTESIAN_POINT('Origin',(427.665215541298,173.610767303216,392.450702781549));
#59563=CARTESIAN_POINT('Origin',(427.665215541298,184.595881223216,392.450702781549));
#59564=CARTESIAN_POINT('',(427.665215541297,194.889871303216,395.671178941549));
#59565=CARTESIAN_POINT('',(427.665215541298,184.595881223216,395.671178941549));
#59566=CARTESIAN_POINT('',(425.793769209445,194.889871303216,395.071610129039));
#59567=CARTESIAN_POINT('Origin',(427.665215541297,194.889871303216,392.450702781549));
#59568=CARTESIAN_POINT('Origin',(427.665215541297,194.889871303216,392.450702781549));
#59569=CARTESIAN_POINT('Origin',(427.665215541297,196.563279803322,392.450702781549));
#59570=CARTESIAN_POINT('',(427.665215541297,196.749214081111,392.450702781549));
#59571=CARTESIAN_POINT('',(427.478070908112,196.563279803322,392.712793516298));
#59572=CARTESIAN_POINT('Origin',(427.665215541299,174.232778759217,497.549298322234));
#59573=CARTESIAN_POINT('',(427.665215541299,174.301891143217,500.769774482234));
#59574=CARTESIAN_POINT('',(425.793769209447,174.301891143217,500.170205669723));
#59575=CARTESIAN_POINT('Origin',(427.665215541299,174.301891143217,497.549298322234));
#59576=CARTESIAN_POINT('Origin',(427.665215541299,174.301891143217,497.549298322234));
#59577=CARTESIAN_POINT('',(425.392151215409,173.610767303217,500.732660244851));
#59578=CARTESIAN_POINT('',(425.753607410043,174.232778759217,500.226451127236));
#59579=CARTESIAN_POINT('Origin',(427.665215541299,173.610767303217,497.549298322234));
#59580=CARTESIAN_POINT('Origin',(427.665215541298,184.595881223217,497.549298322234));
#59581=CARTESIAN_POINT('',(427.665215541297,194.889871303217,500.769774482233));
#59582=CARTESIAN_POINT('',(427.665215541298,184.595881223217,500.769774482234));
#59583=CARTESIAN_POINT('',(425.793769209445,194.889871303218,500.170205669724));
#59584=CARTESIAN_POINT('Origin',(427.665215541297,194.889871303217,497.549298322233));
#59585=CARTESIAN_POINT('Origin',(427.665215541297,194.889871303217,497.549298322233));
#59586=CARTESIAN_POINT('Origin',(427.665215541297,196.563279803324,497.549298322233));
#59587=CARTESIAN_POINT('',(427.665215541297,196.749214081114,497.549298322233));
#59588=CARTESIAN_POINT('',(427.478070908112,196.563279803324,497.811389056982));
#59589=CARTESIAN_POINT('Origin',(322.566620000614,174.232778759209,392.45070278155));
#59590=CARTESIAN_POINT('',(322.566620000614,174.301891143209,395.67117894155));
#59591=CARTESIAN_POINT('',(320.695173668762,174.301891143209,395.071610129039));
#59592=CARTESIAN_POINT('Origin',(322.566620000614,174.301891143209,392.45070278155));
#59593=CARTESIAN_POINT('Origin',(322.566620000614,174.301891143209,392.45070278155));
#59594=CARTESIAN_POINT('',(320.293555674725,173.610767303209,395.634064704167));
#59595=CARTESIAN_POINT('',(320.655011869358,174.232778759209,395.127855586552));
#59596=CARTESIAN_POINT('Origin',(322.566620000614,173.610767303209,392.45070278155));
#59597=CARTESIAN_POINT('Origin',(322.566620000614,184.595881223209,392.45070278155));
#59598=CARTESIAN_POINT('',(322.566620000613,194.889871303209,395.67117894155));
#59599=CARTESIAN_POINT('',(322.566620000614,184.595881223209,395.67117894155));
#59600=CARTESIAN_POINT('',(320.695173668761,194.889871303209,395.071610129039));
#59601=CARTESIAN_POINT('Origin',(322.566620000613,194.889871303209,392.45070278155));
#59602=CARTESIAN_POINT('Origin',(322.566620000613,194.889871303209,392.45070278155));
#59603=CARTESIAN_POINT('Origin',(322.566620000613,196.563279803315,392.45070278155));
#59604=CARTESIAN_POINT('',(322.566620000613,196.749214081104,392.45070278155));
#59605=CARTESIAN_POINT('',(322.379475367428,196.563279803315,392.712793516299));
#59606=CARTESIAN_POINT('Origin',(428.603096951416,291.986959303217,520.996800551891));
#59607=CARTESIAN_POINT('',(428.331267438134,291.986959303217,520.996800551891));
#59608=CARTESIAN_POINT('',(428.603096951416,292.370126934863,521.270399563094));
#59609=CARTESIAN_POINT('Origin',(428.603096951415,291.986959303216,369.003200551891));
#59610=CARTESIAN_POINT('',(428.331267438134,291.986959303216,369.003200551891));
#59611=CARTESIAN_POINT('',(428.603096951415,292.370126934862,369.276799563094));
#59612=CARTESIAN_POINT('Origin',(276.942620190481,291.986959303207,520.996800551891));
#59613=CARTESIAN_POINT('',(277.214449703762,291.986959303207,520.996800551891));
#59614=CARTESIAN_POINT('',(276.942620190481,291.603791671561,521.270399563094));
#59615=CARTESIAN_POINT('Origin',(276.94262019048,291.986959303205,369.003200551891));
#59616=CARTESIAN_POINT('',(277.214449703761,291.986959303206,369.003200551891));
#59617=CARTESIAN_POINT('',(276.94262019048,291.60379167156,369.276799563094));
#59618=CARTESIAN_POINT('Origin',(276.942620190486,202.578959303206,369.003200551892));
#59619=CARTESIAN_POINT('',(277.214449703768,202.578959303206,369.003200551892));
#59620=CARTESIAN_POINT('',(276.942620190486,202.19579167156,369.276799563095));
#59621=CARTESIAN_POINT('Origin',(276.942620190487,202.578959303207,520.996800551892));
#59622=CARTESIAN_POINT('',(277.214449703768,202.578959303207,520.996800551892));
#59623=CARTESIAN_POINT('',(276.942620190487,202.195791671561,521.270399563095));
#59624=CARTESIAN_POINT('Origin',(428.603096951421,202.578959303216,369.003200551891));
#59625=CARTESIAN_POINT('',(428.33126743814,202.578959303216,369.003200551891));
#59626=CARTESIAN_POINT('',(428.603096951421,202.962126934862,369.276799563094));
#59627=CARTESIAN_POINT('Origin',(428.603096951422,202.578959303217,520.996800551891));
#59628=CARTESIAN_POINT('',(428.33126743814,202.578959303217,520.996800551891));
#59629=CARTESIAN_POINT('',(428.603096951422,202.962126934863,521.270399563094));
#59630=CARTESIAN_POINT('Origin',(330.231058744534,208.032452402338,535.164131149611));
#59631=CARTESIAN_POINT('',(327.592975586647,205.44001530321,538.878400551892));
#59632=CARTESIAN_POINT('',(327.592975586647,205.44001530321,538.878400551892));
#59633=CARTESIAN_POINT('',(332.869141902422,210.624889501466,538.878400551892));
#59634=CARTESIAN_POINT('',(332.869141902422,210.624889501466,538.878400551892));
#59635=CARTESIAN_POINT('',(327.592975586647,205.44001530321,538.878400551892));
#59636=CARTESIAN_POINT('Origin',(333.189076396687,228.953924402338,535.345190946332));
#59637=CARTESIAN_POINT('',(333.509010890952,247.282959303211,538.878400551891));
#59638=CARTESIAN_POINT('',(333.509010890952,247.282959303211,538.878400551891));
#59639=CARTESIAN_POINT('',(332.869141902422,210.624889501466,538.878400551892));
#59640=CARTESIAN_POINT('Origin',(263.733073385219,228.953924402334,535.345190946332));
#59641=CARTESIAN_POINT('',(263.413138890952,247.282959303206,538.878400551891));
#59642=CARTESIAN_POINT('',(263.413138890952,247.282959303206,538.878400551891));
#59643=CARTESIAN_POINT('',(264.053007879487,210.624889501461,538.878400551892));
#59644=CARTESIAN_POINT('',(264.053007879487,210.624889501461,538.878400551892));
#59645=CARTESIAN_POINT('',(263.413138890952,247.282959303206,538.878400551891));
#59646=CARTESIAN_POINT('Origin',(333.189076396684,265.611994204083,535.345190946332));
#59647=CARTESIAN_POINT('',(332.869141902417,283.941029104955,538.878400551891));
#59648=CARTESIAN_POINT('',(332.869141902417,283.941029104955,538.878400551891));
#59649=CARTESIAN_POINT('',(333.509010890952,247.282959303211,538.878400551891));
#59650=CARTESIAN_POINT('Origin',(330.231058744529,286.533466204083,535.164131149611));
#59651=CARTESIAN_POINT('',(327.592975586641,289.12590330321,538.878400551891));
#59652=CARTESIAN_POINT('',(327.592975586641,289.12590330321,538.878400551891));
#59653=CARTESIAN_POINT('',(332.869141902417,283.941029104955,538.878400551891));
#59654=CARTESIAN_POINT('Origin',(327.610857186641,289.12590330321,537.030206650751));
#59655=CARTESIAN_POINT('',(269.329174195257,289.125903303206,538.878400551891));
#59656=CARTESIAN_POINT('',(269.329174195257,289.125903303206,538.878400551891));
#59657=CARTESIAN_POINT('',(327.592975586641,289.12590330321,538.878400551891));
#59658=CARTESIAN_POINT('Origin',(266.691091037369,286.533466204079,535.164131149611));
#59659=CARTESIAN_POINT('',(264.053007879482,283.941029104951,538.878400551891));
#59660=CARTESIAN_POINT('',(264.053007879482,283.941029104951,538.878400551891));
#59661=CARTESIAN_POINT('',(269.329174195257,289.125903303206,538.878400551891));
#59662=CARTESIAN_POINT('Origin',(263.733073385216,265.611994204078,535.345190946332));
#59663=CARTESIAN_POINT('',(264.053007879482,283.941029104951,538.878400551891));
#59664=CARTESIAN_POINT('Origin',(333.526892490952,247.282959303211,538.878400551891));
#59665=CARTESIAN_POINT('',(269.329174195263,205.440015303206,538.878400551892));
#59666=CARTESIAN_POINT('',(264.053007879487,210.624889501461,538.878400551892));
#59667=CARTESIAN_POINT('',(269.329174195263,205.440015303206,538.878400551892));
#59668=CARTESIAN_POINT('',(280.579474890949,288.053007303207,538.878400551891));
#59669=CARTESIAN_POINT('',(316.342674890949,288.053007303209,538.878400551891));
#59670=CARTESIAN_POINT('',(280.579474890949,288.053007303207,538.878400551891));
#59671=CARTESIAN_POINT('',(329.75387489095,274.64180730321,538.878400551891));
#59672=CARTESIAN_POINT('',(316.342674890949,288.053007303209,538.878400551891));
#59673=CARTESIAN_POINT('',(329.753874890953,219.92411130321,538.878400551892));
#59674=CARTESIAN_POINT('',(329.75387489095,274.64180730321,538.878400551891));
#59675=CARTESIAN_POINT('',(316.342674890955,206.512911303209,538.878400551892));
#59676=CARTESIAN_POINT('',(329.753874890953,219.92411130321,538.878400551891));
#59677=CARTESIAN_POINT('',(280.579474890954,206.512911303207,538.878400551892));
#59678=CARTESIAN_POINT('',(316.342674890955,206.512911303209,538.878400551892));
#59679=CARTESIAN_POINT('',(267.168274890954,219.924111303206,538.878400551892));
#59680=CARTESIAN_POINT('',(280.579474890954,206.512911303207,538.878400551892));
#59681=CARTESIAN_POINT('',(267.16827489095,274.641807303206,538.878400551891));
#59682=CARTESIAN_POINT('',(267.168274890954,219.924111303206,538.878400551892));
#59683=CARTESIAN_POINT('',(267.16827489095,274.641807303206,538.878400551891));
#59684=CARTESIAN_POINT('Origin',(442.189799370956,184.429135303217,445.000000551891));
#59685=CARTESIAN_POINT('',(375.115917770956,184.429135303212,377.944000551892));
#59686=CARTESIAN_POINT('Origin',(375.115917770956,184.429135303213,445.000000551892));
#59687=CARTESIAN_POINT('',(375.115917770956,184.429135303212,398.051859751892));
#59688=CARTESIAN_POINT('Origin',(375.115917770956,184.429135303213,445.000000551892));
#59689=CARTESIAN_POINT('Origin',(375.115917770956,183.937391303213,445.000000551892));
#59690=CARTESIAN_POINT('',(375.115917770956,183.445647303212,398.051859751892));
#59691=CARTESIAN_POINT('',(375.115917770956,183.937391303212,398.051859751892));
#59692=CARTESIAN_POINT('Origin',(375.115917770956,183.445647303212,445.000000551892));
#59693=CARTESIAN_POINT('Origin',(375.115917770956,174.415439303212,445.000000551892));
#59694=CARTESIAN_POINT('',(375.115917770957,174.504847303213,491.948141351892));
#59695=CARTESIAN_POINT('',(347.833950284685,174.504847303212,483.207619879123));
#59696=CARTESIAN_POINT('Origin',(375.115917770956,174.504847303213,445.000000551892));
#59697=CARTESIAN_POINT('',(347.533983587441,173.610767303209,483.627714704941));
#59698=CARTESIAN_POINT('',(347.80395361496,174.41543930321,483.249629361705));
#59699=CARTESIAN_POINT('Origin',(375.115917770956,173.610767303213,445.000000551892));
#59700=CARTESIAN_POINT('Origin',(375.115917770956,174.504847303213,445.000000551892));
#59701=CARTESIAN_POINT('Origin',(271.071258570951,247.282959303205,330.553791757734));
#59702=CARTESIAN_POINT('Origin',(313.603213770946,320.847861703208,383.487296551891));
#59703=CARTESIAN_POINT('',(303.589517770946,320.829980103207,393.500992551891));
#59704=CARTESIAN_POINT('Origin',(436.628621770955,192.583144903216,383.487296551891));
#59705=CARTESIAN_POINT('',(446.642317770956,173.610767303217,393.500992551891));
#59706=CARTESIAN_POINT('',(446.642317770956,173.610767303217,393.500992551891));
#59707=CARTESIAN_POINT('',(426.614925770956,173.610767303216,373.473600551892));
#59708=CARTESIAN_POINT('Origin',(446.642317770956,183.088015303217,393.483110951891));
#59709=CARTESIAN_POINT('',(446.642317770957,173.610767303218,496.499008551892));
#59710=CARTESIAN_POINT('',(446.642317770957,173.610767303218,496.499008551892));
#59711=CARTESIAN_POINT('',(446.642317770956,173.610767303217,393.500992551891));
#59712=CARTESIAN_POINT('Origin',(436.628621770955,192.583144903217,506.512704551891));
#59713=CARTESIAN_POINT('',(426.614925770957,173.610767303217,516.526400551892));
#59714=CARTESIAN_POINT('',(426.614925770957,173.610767303217,516.526400551892));
#59715=CARTESIAN_POINT('',(446.642317770957,173.610767303218,496.499008551892));
#59716=CARTESIAN_POINT('Origin',(426.632807370956,183.088015303217,516.526400551892));
#59717=CARTESIAN_POINT('',(323.616909770957,173.61076730321,516.526400551892));
#59718=CARTESIAN_POINT('',(323.616909770957,173.61076730321,516.526400551892));
#59719=CARTESIAN_POINT('',(426.614925770957,173.610767303217,516.526400551892));
#59720=CARTESIAN_POINT('Origin',(313.603213770955,192.583144903209,506.512704551892));
#59721=CARTESIAN_POINT('',(303.589517770957,173.610767303208,496.499008551892));
#59722=CARTESIAN_POINT('',(303.589517770957,173.610767303208,496.499008551892));
#59723=CARTESIAN_POINT('',(323.616909770957,173.61076730321,516.526400551892));
#59724=CARTESIAN_POINT('Origin',(303.589517770956,183.088015303207,393.483110951892));
#59725=CARTESIAN_POINT('',(303.589517770957,173.610767303208,496.499008551892));
#59726=CARTESIAN_POINT('Origin',(446.660199370957,173.610767303218,445.000000551892));
#59727=CARTESIAN_POINT('Origin',(327.610857186647,205.44001530321,537.030206650751));
#59728=CARTESIAN_POINT('',(269.329174195263,205.440015303206,538.878400551892));
#59729=CARTESIAN_POINT('Origin',(266.691091037374,208.032452402334,535.164131149612));
#59730=CARTESIAN_POINT('Origin',(317.611309698624,205.871791230878,335.477394119332));
#59731=CARTESIAN_POINT('Origin',(375.115917770952,313.069365703204,445.000000551892));
#59732=CARTESIAN_POINT('',(375.115917770947,312.962076103212,377.94400055189));
#59733=CARTESIAN_POINT('',(336.149100755717,312.962076103188,390.428081878454));
#59734=CARTESIAN_POINT('Origin',(375.115917770947,312.962076103213,445.00000055189));
#59735=CARTESIAN_POINT('Origin',(375.115917770947,312.962076103213,445.00000055189));
#59736=CARTESIAN_POINT('',(335.789140719017,314.034972103212,389.923968087461));
#59737=CARTESIAN_POINT('',(336.113104752046,313.069365703191,390.377670499354));
#59738=CARTESIAN_POINT('Origin',(375.115917770947,314.034972103213,445.00000055189));
#59739=CARTESIAN_POINT('Origin',(359.022477770951,247.282959303211,363.526482809593));
#59740=CARTESIAN_POINT('',(359.022477770953,217.089877703211,379.903853776783));
#59741=CARTESIAN_POINT('',(359.022477770953,217.089877703211,363.526482809593));
#59742=CARTESIAN_POINT('',(375.115917770953,221.736465111823,377.944000551891));
#59743=CARTESIAN_POINT('Ctrl Pts',(375.115917770953,221.736465111823,377.944000551891));
#59744=CARTESIAN_POINT('Ctrl Pts',(373.636790201116,220.804664034964,377.944000551891));
#59745=CARTESIAN_POINT('Ctrl Pts',(372.061821595824,219.993987408909,377.993721471897));
#59746=CARTESIAN_POINT('Ctrl Pts',(368.577472050991,218.571521074051,378.23758179025));
#59747=CARTESIAN_POINT('Ctrl Pts',(366.648020923175,218.002843790601,378.452212963473));
#59748=CARTESIAN_POINT('Ctrl Pts',(362.793307997576,217.262051385977,379.057096473175));
#59749=CARTESIAN_POINT('Ctrl Pts',(360.86809223922,217.089877703211,379.447570460802));
#59750=CARTESIAN_POINT('Ctrl Pts',(359.022477770953,217.089877703211,379.903853776783));
#59751=CARTESIAN_POINT('',(375.115917770927,272.829453494629,377.944000551891));
#59752=CARTESIAN_POINT('Ctrl Pts',(375.115917770905,272.829453494629,377.944000551891));
#59753=CARTESIAN_POINT('Ctrl Pts',(375.324314296131,272.698170628581,377.944000551891));
#59754=CARTESIAN_POINT('Ctrl Pts',(375.530826414793,272.564512070292,377.944972249753));
#59755=CARTESIAN_POINT('Ctrl Pts',(377.391519391247,271.327814419871,377.962161223403));
#59756=CARTESIAN_POINT('Ctrl Pts',(378.915731826797,270.075157816713,378.03807646561));
#59757=CARTESIAN_POINT('Ctrl Pts',(381.621934327401,267.395986355681,378.246486242121));
#59758=CARTESIAN_POINT('Ctrl Pts',(382.893971040304,265.877729518232,378.387027646642));
#59759=CARTESIAN_POINT('Ctrl Pts',(385.135941372981,262.570231420126,378.687215969435));
#59760=CARTESIAN_POINT('Ctrl Pts',(386.106062898885,260.781039831472,378.84600614933));
#59761=CARTESIAN_POINT('Ctrl Pts',(387.665333692241,257.045413463659,379.124007415217));
#59762=CARTESIAN_POINT('Ctrl Pts',(388.255709793393,255.095882880109,379.24279855252));
#59763=CARTESIAN_POINT('Ctrl Pts',(389.030925142045,251.170981356928,379.402467677427));
#59764=CARTESIAN_POINT('Ctrl Pts',(389.215559370951,249.195559926263,379.44309974998));
#59765=CARTESIAN_POINT('Ctrl Pts',(389.215559370951,245.370358680163,379.44309974998));
#59766=CARTESIAN_POINT('Ctrl Pts',(389.030925142045,243.394937249498,379.402467677427));
#59767=CARTESIAN_POINT('Ctrl Pts',(388.255709793394,239.470035726317,379.24279855252));
#59768=CARTESIAN_POINT('Ctrl Pts',(387.665333692242,237.520505142767,379.124007415217));
#59769=CARTESIAN_POINT('Ctrl Pts',(386.106062898887,233.784878774954,378.84600614933));
#59770=CARTESIAN_POINT('Ctrl Pts',(385.135941372983,231.9956871863,378.687215969435));
#59771=CARTESIAN_POINT('Ctrl Pts',(382.893971040307,228.688189088194,378.387027646642));
#59772=CARTESIAN_POINT('Ctrl Pts',(381.621934327403,227.169932250744,378.246486242122));
#59773=CARTESIAN_POINT('Ctrl Pts',(378.9157318268,224.490760789712,378.038076465611));
#59774=CARTESIAN_POINT('Ctrl Pts',(377.39151939125,223.238104186553,377.962161223404));
#59775=CARTESIAN_POINT('Ctrl Pts',(375.530826414811,222.001406536142,377.944972249754));
#59776=CARTESIAN_POINT('Ctrl Pts',(375.324314296163,221.867747977862,377.944000551891));
#59777=CARTESIAN_POINT('Ctrl Pts',(375.115917770953,221.736465111823,377.944000551891));
#59778=CARTESIAN_POINT('Ctrl Pts',(359.022477770953,217.089877703211,379.903853776783));
#59779=CARTESIAN_POINT('Ctrl Pts',(356.987690988922,217.089877703211,380.406905349138));
#59780=CARTESIAN_POINT('Ctrl Pts',(354.919861382001,217.298453320156,381.021595941104));
#59781=CARTESIAN_POINT('Ctrl Pts',(350.868410694004,218.138264239459,382.444622280587));
#59782=CARTESIAN_POINT('Ctrl Pts',(348.884628885239,218.768978182231,383.252808054169));
#59783=CARTESIAN_POINT('Ctrl Pts',(345.124132814251,220.400640082137,384.989258968462));
#59784=CARTESIAN_POINT('Ctrl Pts',(343.344590306969,221.402426333465,385.918364292264));
#59785=CARTESIAN_POINT('Ctrl Pts',(340.077241909773,223.688973202756,387.795558540336));
#59786=CARTESIAN_POINT('Ctrl Pts',(338.5892495324,224.973941335523,388.743070052525));
#59787=CARTESIAN_POINT('Ctrl Pts',(336.046567394082,227.614002320155,390.481116463648));
#59788=CARTESIAN_POINT('Ctrl Pts',(334.878783177339,229.05453689296,391.341550794677));
#59789=CARTESIAN_POINT('Ctrl Pts',(332.79430570224,232.207271532133,392.969842155029));
#59790=CARTESIAN_POINT('Ctrl Pts',(331.877170850109,233.919572526647,393.73693833283));
#59791=CARTESIAN_POINT('Ctrl Pts',(330.379937606024,237.533474697026,395.038184711296));
#59792=CARTESIAN_POINT('Ctrl Pts',(329.798561481046,239.439070802072,395.572021113079));
#59793=CARTESIAN_POINT('Ctrl Pts',(329.023070644187,243.333346648986,396.294380977303));
#59794=CARTESIAN_POINT('Ctrl Pts',(328.829396170951,245.322412916721,396.481292261452));
#59795=CARTESIAN_POINT('Ctrl Pts',(328.829396170951,247.282959303209,396.481292261452));
#59796=CARTESIAN_POINT('Ctrl Pts',(328.829396170951,249.243505689698,396.481292261452));
#59797=CARTESIAN_POINT('Ctrl Pts',(329.023070644186,251.232571957432,396.294380977303));
#59798=CARTESIAN_POINT('Ctrl Pts',(329.798561481045,255.126847804347,395.572021113079));
#59799=CARTESIAN_POINT('Ctrl Pts',(330.379937606023,257.032443909393,395.038184711295));
#59800=CARTESIAN_POINT('Ctrl Pts',(331.877170850107,260.646346079772,393.73693833283));
#59801=CARTESIAN_POINT('Ctrl Pts',(332.794305702238,262.358647074286,392.969842155029));
#59802=CARTESIAN_POINT('Ctrl Pts',(334.878783177337,265.511381713459,391.341550794677));
#59803=CARTESIAN_POINT('Ctrl Pts',(336.046567394079,266.951916286264,390.481116463648));
#59804=CARTESIAN_POINT('Ctrl Pts',(338.589249532397,269.591977270897,388.743070052524));
#59805=CARTESIAN_POINT('Ctrl Pts',(340.07724190977,270.876945403664,387.795558540335));
#59806=CARTESIAN_POINT('Ctrl Pts',(343.344590306966,273.163492272956,385.918364292264));
#59807=CARTESIAN_POINT('Ctrl Pts',(345.124132814247,274.165278524283,384.989258968461));
#59808=CARTESIAN_POINT('Ctrl Pts',(348.884628885235,275.79694042419,383.252808054168));
#59809=CARTESIAN_POINT('Ctrl Pts',(350.868410694,276.427654366962,382.444622280586));
#59810=CARTESIAN_POINT('Ctrl Pts',(354.919861381997,277.267465286266,381.021595941103));
#59811=CARTESIAN_POINT('Ctrl Pts',(356.987690988918,277.476040903211,380.406905349137));
#59812=CARTESIAN_POINT('Ctrl Pts',(360.868092239216,277.476040903211,379.447570460801));
#59813=CARTESIAN_POINT('Ctrl Pts',(362.793307997572,277.303867220446,379.057096473175));
#59814=CARTESIAN_POINT('Ctrl Pts',(366.648020923171,276.563074815822,378.452212963473));
#59815=CARTESIAN_POINT('Ctrl Pts',(368.577472050987,275.994397532373,378.23758179025));
#59816=CARTESIAN_POINT('Ctrl Pts',(372.061821595804,274.571931197522,377.993721471898));
#59817=CARTESIAN_POINT('Ctrl Pts',(373.636790201081,273.761254571476,377.944000551891));
#59818=CARTESIAN_POINT('Ctrl Pts',(375.115917770905,272.829453494629,377.944000551891));
#59819=CARTESIAN_POINT('Origin',(298.461074890952,247.282959303209,538.073728551892));
#59820=CARTESIAN_POINT('',(281.384594574745,271.198084181898,538.878400551893));
#59821=CARTESIAN_POINT('',(281.654564602264,270.819998838662,538.073728551893));
#59822=CARTESIAN_POINT('Origin',(298.461074890952,247.282959303208,538.878400551891));
#59823=CARTESIAN_POINT('Origin',(375.115917770951,248.695605703213,445.000000551891));
#59824=CARTESIAN_POINT('',(375.115917770951,248.695605703212,377.944000551891));
#59825=CARTESIAN_POINT('',(375.115917770951,248.695605703212,377.944000551891));
#59826=CARTESIAN_POINT('Origin',(400.433645843278,288.694127375543,334.86186607715));
#59827=CARTESIAN_POINT('Origin',(400.433645843284,205.871791230884,334.86186607715));
#59828=CARTESIAN_POINT('Origin',(375.115917770948,301.607260103212,445.000000551891));
#59829=CARTESIAN_POINT('',(375.115917770949,292.219420103213,491.948141351891));
#59830=CARTESIAN_POINT('Origin',(375.115917770948,292.219420103212,445.000000551891));
#59831=CARTESIAN_POINT('',(375.115917770947,310.995100103213,491.948141351891));
#59832=CARTESIAN_POINT('',(375.115917770948,301.607260103213,491.948141351891));
#59833=CARTESIAN_POINT('Origin',(375.115917770947,310.995100103212,445.000000551891));
#59834=CARTESIAN_POINT('Origin',(375.115917770946,320.025308103214,445.00000055189));
#59835=CARTESIAN_POINT('',(347.833950284676,319.93590010321,406.792381224659));
#59836=CARTESIAN_POINT('',(375.115917770947,319.935900103213,491.94814135189));
#59837=CARTESIAN_POINT('Origin',(375.115917770947,319.935900103212,445.00000055189));
#59838=CARTESIAN_POINT('Origin',(375.115917770947,319.935900103212,445.00000055189));
#59839=CARTESIAN_POINT('',(347.533983587431,320.829980103214,406.37228639884));
#59840=CARTESIAN_POINT('',(347.80395361495,320.025308103214,406.750371742075));
#59841=CARTESIAN_POINT('Origin',(375.115917770947,320.829980103212,445.00000055189));
#59842=CARTESIAN_POINT('Origin',(446.660199370947,320.829980103217,445.00000055189));
#59843=CARTESIAN_POINT('',(430.89144884552,320.829980103216,386.862702781548));
#59844=CARTESIAN_POINT('',(434.117682149752,320.829980103216,392.450702781548));
#59845=CARTESIAN_POINT('',(430.89144884552,320.829980103216,386.862702781548));
#59846=CARTESIAN_POINT('',(430.89144884552,320.829980103216,398.038702781548));
#59847=CARTESIAN_POINT('',(434.117682149752,320.829980103216,392.450702781548));
#59848=CARTESIAN_POINT('',(424.438982237057,320.829980103215,398.038702781548));
#59849=CARTESIAN_POINT('',(430.89144884552,320.829980103216,398.038702781548));
#59850=CARTESIAN_POINT('',(421.212748932825,320.829980103215,392.450702781548));
#59851=CARTESIAN_POINT('',(424.438982237057,320.829980103215,398.038702781548));
#59852=CARTESIAN_POINT('',(424.438982237057,320.829980103215,386.862702781548));
#59853=CARTESIAN_POINT('',(421.212748932825,320.829980103215,392.450702781548));
#59854=CARTESIAN_POINT('',(424.438982237057,320.829980103215,386.862702781548));
#59855=CARTESIAN_POINT('',(325.792853304836,320.82998010321,491.961298322233));
#59856=CARTESIAN_POINT('',(329.019086609068,320.82998010321,497.549298322233));
#59857=CARTESIAN_POINT('',(325.792853304836,320.829980103209,491.961298322233));
#59858=CARTESIAN_POINT('',(325.792853304836,320.82998010321,503.137298322233));
#59859=CARTESIAN_POINT('',(329.019086609068,320.82998010321,497.549298322233));
#59860=CARTESIAN_POINT('',(319.340386696373,320.829980103209,503.137298322233));
#59861=CARTESIAN_POINT('',(325.792853304836,320.82998010321,503.137298322233));
#59862=CARTESIAN_POINT('',(316.114153392142,320.829980103209,497.549298322233));
#59863=CARTESIAN_POINT('',(319.340386696373,320.829980103209,503.137298322233));
#59864=CARTESIAN_POINT('',(319.340386696373,320.829980103209,491.961298322233));
#59865=CARTESIAN_POINT('',(316.114153392142,320.829980103209,497.549298322233));
#59866=CARTESIAN_POINT('',(319.340386696373,320.829980103209,491.961298322233));
#59867=CARTESIAN_POINT('Origin',(442.162976970949,292.219420103217,445.000000551891));
#59868=CARTESIAN_POINT('',(375.115917770949,292.219420103213,512.029178151891));
#59869=CARTESIAN_POINT('Origin',(375.115917770948,292.219420103212,445.000000551891));
#59870=CARTESIAN_POINT('Origin',(375.115917770948,303.127196103212,445.000000551891));
#59871=CARTESIAN_POINT('',(375.115917770947,314.034972103213,512.029178151891));
#59872=CARTESIAN_POINT('Origin',(375.115917770947,314.034972103212,445.000000551891));
#59873=CARTESIAN_POINT('',(375.115917770948,303.127196103213,512.029178151891));
#59874=CARTESIAN_POINT('Origin',(442.80923616536,314.034972103217,445.00000055189));
#59875=CARTESIAN_POINT('Origin',(392.118190090946,325.425551303214,445.00000055189));
#59876=CARTESIAN_POINT('',(392.595628810946,325.425551303214,442.25249271189));
#59877=CARTESIAN_POINT('',(392.595628810946,327.022151685719,442.764007137444));
#59878=CARTESIAN_POINT('Origin',(392.595628810946,325.425551303214,445.00000055189));
#59879=CARTESIAN_POINT('Origin',(392.595628810946,325.425551303214,445.00000055189));
#59880=CARTESIAN_POINT('',(391.640751370946,325.425551303214,442.25249271189));
#59881=CARTESIAN_POINT('',(392.118190090946,325.425551303214,442.25249271189));
#59882=CARTESIAN_POINT('Origin',(391.640751370946,325.425551303214,445.00000055189));
#59883=CARTESIAN_POINT('Origin',(375.115917770946,331.254952903213,445.00000055189));
#59884=CARTESIAN_POINT('',(353.03991703791,331.147663303211,475.916811544351));
#59885=CARTESIAN_POINT('',(375.115917770946,331.147663303212,407.01054135189));
#59886=CARTESIAN_POINT('Origin',(375.115917770946,331.147663303213,445.00000055189));
#59887=CARTESIAN_POINT('Origin',(375.115917770946,331.147663303213,445.00000055189));
#59888=CARTESIAN_POINT('',(353.399877074602,332.220559303212,475.41269775337));
#59889=CARTESIAN_POINT('',(353.075913041579,331.254952903211,475.866400165253));
#59890=CARTESIAN_POINT('Origin',(375.115917770946,332.220559303213,445.00000055189));
#59891=CARTESIAN_POINT('Origin',(412.503821776533,332.220559303215,445.00000055189));
#59892=CARTESIAN_POINT('',(391.640751370946,332.220559303214,448.36174135189));
#59893=CARTESIAN_POINT('',(391.640751370946,332.220559303214,441.63825975189));
#59894=CARTESIAN_POINT('',(391.640751370946,332.220559303214,448.36174135189));
#59895=CARTESIAN_POINT('',(389.391142518186,332.220559303214,448.36174135189));
#59896=CARTESIAN_POINT('',(391.640751370946,332.220559303214,448.36174135189));
#59897=CARTESIAN_POINT('',(389.391142518186,332.220559303214,441.63825975189));
#59898=CARTESIAN_POINT('Origin',(375.115917770946,332.220559303213,445.00000055189));
#59899=CARTESIAN_POINT('',(391.640751370946,332.220559303214,441.63825975189));
#59900=CARTESIAN_POINT('Origin',(375.115917770946,330.289346503213,445.00000055189));
#59901=CARTESIAN_POINT('',(388.115106324191,330.074767303214,441.63825975189));
#59902=CARTESIAN_POINT('',(388.115106324191,330.074767303214,448.36174135189));
#59903=CARTESIAN_POINT('Origin',(375.115917770946,330.074767303213,445.00000055189));
#59904=CARTESIAN_POINT('Ctrl Pts',(388.115106324191,330.074767303214,441.63825975189));
#59905=CARTESIAN_POINT('Ctrl Pts',(388.541335653371,330.789504164161,441.63825975189));
#59906=CARTESIAN_POINT('Ctrl Pts',(388.966604868582,331.504817465291,441.63825975189));
#59907=CARTESIAN_POINT('Ctrl Pts',(389.391142518186,332.220559303214,441.63825975189));
#59908=CARTESIAN_POINT('Ctrl Pts',(389.391142518186,332.220559303214,448.36174135189));
#59909=CARTESIAN_POINT('Ctrl Pts',(388.966603199871,331.504814651955,448.36174135189));
#59910=CARTESIAN_POINT('Ctrl Pts',(388.54133083666,330.789496087098,448.36174135189));
#59911=CARTESIAN_POINT('Ctrl Pts',(388.115106324191,330.074767303214,448.36174135189));
#59912=CARTESIAN_POINT('Origin',(403.843567738701,147.345359303214,445.000000551892));
#59913=CARTESIAN_POINT('',(358.432425010641,147.345359303211,421.635243565227));
#59914=CARTESIAN_POINT('Origin',(375.115917770958,147.345359303212,445.000000551892));
#59915=CARTESIAN_POINT('Origin',(375.115917770951,247.282959303213,445.000000551891));
#59916=CARTESIAN_POINT('',(388.115106324202,164.491151303213,448.361741351892));
#59917=CARTESIAN_POINT('',(388.115106324191,330.074767303214,448.36174135189));
#59918=CARTESIAN_POINT('',(388.115106324202,164.491151303213,441.638259751892));
#59919=CARTESIAN_POINT('Origin',(375.115917770957,164.491151303213,445.000000551892));
#59920=CARTESIAN_POINT('',(388.115106324202,164.491151303213,441.638259751892));
#59921=CARTESIAN_POINT('',(370.923963348087,169.140367303212,457.755694275315));
#59922=CARTESIAN_POINT('Ctrl Pts',(370.923963348087,169.140367303212,457.755694275315));
#59923=CARTESIAN_POINT('Ctrl Pts',(370.923963348087,169.48641478499,457.755694275315));
#59924=CARTESIAN_POINT('Ctrl Pts',(370.856354814583,169.854836977962,457.734079023222));
#59925=CARTESIAN_POINT('Ctrl Pts',(370.586255285233,170.531462911025,457.640522237506));
#59926=CARTESIAN_POINT('Ctrl Pts',(370.384223692787,170.839753936057,457.567887535573));
#59927=CARTESIAN_POINT('Ctrl Pts',(369.927073334233,171.326528548091,457.386145959219));
#59928=CARTESIAN_POINT('Ctrl Pts',(369.641199463923,171.537822113727,457.264699280901));
#59929=CARTESIAN_POINT('Ctrl Pts',(369.02859564363,171.818522071294,456.972464156601));
#59930=CARTESIAN_POINT('Ctrl Pts',(368.702162046036,171.887875143212,456.801003724408));
#59931=CARTESIAN_POINT('Ctrl Pts',(368.102827095877,171.887875143212,456.454977529599));
#59932=CARTESIAN_POINT('Ctrl Pts',(367.791121207057,171.818522071294,456.258007957531));
#59933=CARTESIAN_POINT('Ctrl Pts',(367.231736255389,171.537822113727,455.873595048851));
#59934=CARTESIAN_POINT('Ctrl Pts',(366.983623411605,171.326528548091,455.686744354044));
#59935=CARTESIAN_POINT('Ctrl Pts',(366.597655410281,170.839753936057,455.381711318364));
#59936=CARTESIAN_POINT('Ctrl Pts',(366.433736116989,170.531462911025,455.243064177905));
#59937=CARTESIAN_POINT('Ctrl Pts',(366.217663799188,169.854836977962,455.055929516796));
#59938=CARTESIAN_POINT('Ctrl Pts',(366.165140175013,169.486414784989,455.008186435315));
#59939=CARTESIAN_POINT('Ctrl Pts',(366.165140175013,168.794319821435,455.008186435315));
#59940=CARTESIAN_POINT('Ctrl Pts',(366.217663799188,168.425897628462,455.055929516796));
#59941=CARTESIAN_POINT('Ctrl Pts',(366.433736116989,167.749271695399,455.243064177905));
#59942=CARTESIAN_POINT('Ctrl Pts',(366.597655410282,167.440980670367,455.381711318364));
#59943=CARTESIAN_POINT('Ctrl Pts',(366.983623411605,166.954206058333,455.686744354044));
#59944=CARTESIAN_POINT('Ctrl Pts',(367.231736255389,166.742912492697,455.873595048851));
#59945=CARTESIAN_POINT('Ctrl Pts',(367.791121207058,166.46221253513,456.258007957531));
#59946=CARTESIAN_POINT('Ctrl Pts',(368.102827095878,166.392859463212,456.454977529599));
#59947=CARTESIAN_POINT('Ctrl Pts',(368.702162046036,166.392859463212,456.801003724408));
#59948=CARTESIAN_POINT('Ctrl Pts',(369.02859564363,166.46221253513,456.972464156601));
#59949=CARTESIAN_POINT('Ctrl Pts',(369.641199463924,166.742912492697,457.264699280901));
#59950=CARTESIAN_POINT('Ctrl Pts',(369.927073334233,166.954206058333,457.386145959219));
#59951=CARTESIAN_POINT('Ctrl Pts',(370.384223692787,167.440980670368,457.567887535574));
#59952=CARTESIAN_POINT('Ctrl Pts',(370.586255285233,167.749271695399,457.640522237506));
#59953=CARTESIAN_POINT('Ctrl Pts',(370.856354814583,168.425897628462,457.734079023222));
#59954=CARTESIAN_POINT('Ctrl Pts',(370.923963348087,168.794319821435,457.755694275315));
#59955=CARTESIAN_POINT('Ctrl Pts',(370.923963348087,169.140367303212,457.755694275315));
#59956=CARTESIAN_POINT('',(366.165140175003,325.425551303212,434.991814668467));
#59957=CARTESIAN_POINT('Ctrl Pts',(366.165140175003,325.425551303212,434.991814668467));
#59958=CARTESIAN_POINT('Ctrl Pts',(366.165140175003,325.771598784989,434.991814668467));
#59959=CARTESIAN_POINT('Ctrl Pts',(366.217663799177,326.140020977962,434.944071586987));
#59960=CARTESIAN_POINT('Ctrl Pts',(366.433736116978,326.816646911025,434.756936925877));
#59961=CARTESIAN_POINT('Ctrl Pts',(366.597655410271,327.124937936057,434.618289785419));
#59962=CARTESIAN_POINT('Ctrl Pts',(366.983623411595,327.611712548091,434.313256749738));
#59963=CARTESIAN_POINT('Ctrl Pts',(367.231736255378,327.823006113727,434.126406054932));
#59964=CARTESIAN_POINT('Ctrl Pts',(367.791121207047,328.103706071295,433.741993146252));
#59965=CARTESIAN_POINT('Ctrl Pts',(368.102827095867,328.173059143212,433.545023574183));
#59966=CARTESIAN_POINT('Ctrl Pts',(368.702162046025,328.173059143212,433.198997379374));
#59967=CARTESIAN_POINT('Ctrl Pts',(369.028595643619,328.103706071295,433.027536947181));
#59968=CARTESIAN_POINT('Ctrl Pts',(369.641199463913,327.823006113727,432.735301822882));
#59969=CARTESIAN_POINT('Ctrl Pts',(369.927073334222,327.611712548091,432.613855144563));
#59970=CARTESIAN_POINT('Ctrl Pts',(370.384223692777,327.124937936057,432.432113568209));
#59971=CARTESIAN_POINT('Ctrl Pts',(370.586255285222,326.816646911026,432.359478866277));
#59972=CARTESIAN_POINT('Ctrl Pts',(370.856354814572,326.140020977963,432.265922080561));
#59973=CARTESIAN_POINT('Ctrl Pts',(370.923963348077,325.77159878499,432.244306828467));
#59974=CARTESIAN_POINT('Ctrl Pts',(370.923963348077,325.079503821435,432.244306828467));
#59975=CARTESIAN_POINT('Ctrl Pts',(370.856354814573,324.711081628462,432.265922080561));
#59976=CARTESIAN_POINT('Ctrl Pts',(370.586255285223,324.034455695399,432.359478866277));
#59977=CARTESIAN_POINT('Ctrl Pts',(370.384223692777,323.726164670368,432.432113568209));
#59978=CARTESIAN_POINT('Ctrl Pts',(369.927073334222,323.239390058333,432.613855144563));
#59979=CARTESIAN_POINT('Ctrl Pts',(369.641199463913,323.028096492698,432.735301822882));
#59980=CARTESIAN_POINT('Ctrl Pts',(369.028595643619,322.74739653513,433.027536947181));
#59981=CARTESIAN_POINT('Ctrl Pts',(368.702162046026,322.678043463212,433.198997379374));
#59982=CARTESIAN_POINT('Ctrl Pts',(368.102827095867,322.678043463212,433.545023574183));
#59983=CARTESIAN_POINT('Ctrl Pts',(367.791121207047,322.74739653513,433.741993146252));
#59984=CARTESIAN_POINT('Ctrl Pts',(367.231736255379,323.028096492697,434.126406054932));
#59985=CARTESIAN_POINT('Ctrl Pts',(366.983623411595,323.239390058333,434.313256749738));
#59986=CARTESIAN_POINT('Ctrl Pts',(366.597655410271,323.726164670367,434.618289785419));
#59987=CARTESIAN_POINT('Ctrl Pts',(366.433736116978,324.034455695399,434.756936925877));
#59988=CARTESIAN_POINT('Ctrl Pts',(366.217663799177,324.711081628462,434.944071586987));
#59989=CARTESIAN_POINT('Ctrl Pts',(366.165140175003,325.079503821435,434.991814668467));
#59990=CARTESIAN_POINT('Ctrl Pts',(366.165140175003,325.425551303212,434.991814668467));
#59991=CARTESIAN_POINT('Origin',(392.118190090957,169.140367303214,445.000000551892));
#59992=CARTESIAN_POINT('',(392.595628810957,169.140367303214,442.252492711892));
#59993=CARTESIAN_POINT('',(392.595628810957,170.736967685718,442.764007137445));
#59994=CARTESIAN_POINT('Origin',(392.595628810957,169.140367303214,445.000000551892));
#59995=CARTESIAN_POINT('Origin',(392.595628810957,169.140367303214,445.000000551892));
#59996=CARTESIAN_POINT('',(391.640751370957,169.140367303214,442.252492711892));
#59997=CARTESIAN_POINT('',(392.118190090957,169.140367303214,442.252492711892));
#59998=CARTESIAN_POINT('Origin',(391.640751370957,169.140367303214,445.000000551892));
#59999=CARTESIAN_POINT('Origin',(391.640751370957,162.327477703214,445.000000551892));
#60000=CARTESIAN_POINT('',(391.640751370946,332.220559303214,448.36174135189));
#60001=CARTESIAN_POINT('',(391.640751370946,332.220559303214,441.63825975189));
#60002=CARTESIAN_POINT('Origin',(356.121188170946,323.85907771718,412.100163808658));
#60003=CARTESIAN_POINT('',(357.282632160469,326.199847296226,411.429603808658));
#60004=CARTESIAN_POINT('',(357.28263216047,324.651255310195,411.429603808658));
#60005=CARTESIAN_POINT('',(357.282632160469,326.199847296226,411.429603808658));
#60006=CARTESIAN_POINT('',(356.121188170946,323.87695931718,412.100163808658));
#60007=CARTESIAN_POINT('',(357.28263216047,324.651255310195,411.429603808658));
#60008=CARTESIAN_POINT('',(354.959744181423,324.651255310195,412.770723808658));
#60009=CARTESIAN_POINT('',(356.121188170946,323.87695931718,412.100163808658));
#60010=CARTESIAN_POINT('',(354.959744181423,326.199847296226,412.770723808658));
#60011=CARTESIAN_POINT('',(354.959744181423,324.651255310195,412.770723808658));
#60012=CARTESIAN_POINT('',(356.121188170946,326.974143289242,412.100163808658));
#60013=CARTESIAN_POINT('',(354.959744181423,326.199847296226,412.770723808658));
#60014=CARTESIAN_POINT('',(356.121188170946,326.974143289242,412.100163808658));
#60015=CARTESIAN_POINT('Origin',(356.3929721424,326.416159246118,410.637994030892));
#60016=CARTESIAN_POINT('',(355.674148170946,326.974143289242,411.325867815642));
#60017=CARTESIAN_POINT('',(356.835592160469,326.199847296226,410.655307815642));
#60018=CARTESIAN_POINT('',(355.674148170946,326.974143289242,411.325867815642));
#60019=CARTESIAN_POINT('',(357.282632160469,326.199847296226,411.429603808658));
#60020=CARTESIAN_POINT('',(356.121188170946,326.974143289242,412.100163808658));
#60021=CARTESIAN_POINT('Origin',(355.231528152876,326.757831339351,411.308554030892));
#60022=CARTESIAN_POINT('',(354.512704181423,326.199847296226,411.996427815642));
#60023=CARTESIAN_POINT('',(354.512704181423,326.199847296226,411.996427815642));
#60024=CARTESIAN_POINT('',(354.959744181423,326.199847296226,412.770723808658));
#60025=CARTESIAN_POINT('Origin',(354.736224181423,324.633373710195,412.38357581215));
#60026=CARTESIAN_POINT('',(354.512704181423,324.651255310195,411.996427815642));
#60027=CARTESIAN_POINT('',(354.959744181423,324.651255310195,412.770723808658));
#60028=CARTESIAN_POINT('',(354.512704181423,326.199847296226,411.996427815642));
#60029=CARTESIAN_POINT('Origin',(355.231528152876,324.093271267072,411.308554030892));
#60030=CARTESIAN_POINT('',(355.674148170946,323.87695931718,411.325867815642));
#60031=CARTESIAN_POINT('',(355.674148170946,323.87695931718,411.325867815642));
#60032=CARTESIAN_POINT('',(356.121188170946,323.87695931718,412.100163808658));
#60033=CARTESIAN_POINT('Origin',(356.3929721424,324.434943360304,410.637994030892));
#60034=CARTESIAN_POINT('',(356.83559216047,324.651255310195,410.655307815642));
#60035=CARTESIAN_POINT('',(356.83559216047,324.651255310195,410.655307815642));
#60036=CARTESIAN_POINT('',(357.28263216047,324.651255310195,411.429603808658));
#60037=CARTESIAN_POINT('Origin',(357.05911216047,324.633373710195,411.04245581215));
#60038=CARTESIAN_POINT('',(356.835592160469,326.199847296226,410.655307815642));
#60039=CARTESIAN_POINT('Origin',(413.105376970946,323.859077717184,445.00000055189));
#60040=CARTESIAN_POINT('',(413.105376970946,326.19984729623,446.34112055189));
#60041=CARTESIAN_POINT('',(413.105376970946,324.651255310199,446.34112055189));
#60042=CARTESIAN_POINT('',(413.105376970946,326.19984729623,446.34112055189));
#60043=CARTESIAN_POINT('',(413.105376970946,323.876959317184,445.00000055189));
#60044=CARTESIAN_POINT('',(413.105376970946,324.651255310199,446.34112055189));
#60045=CARTESIAN_POINT('',(413.105376970946,324.651255310199,443.65888055189));
#60046=CARTESIAN_POINT('',(413.105376970946,323.876959317184,445.00000055189));
#60047=CARTESIAN_POINT('',(413.105376970946,326.19984729623,443.65888055189));
#60048=CARTESIAN_POINT('',(413.105376970946,324.651255310199,443.65888055189));
#60049=CARTESIAN_POINT('',(413.105376970946,326.974143289246,445.00000055189));
#60050=CARTESIAN_POINT('',(413.105376970946,326.19984729623,443.65888055189));
#60051=CARTESIAN_POINT('',(413.105376970946,326.974143289246,445.00000055189));
#60052=CARTESIAN_POINT('Origin',(414.017338570946,326.586995292738,445.67056055189));
#60053=CARTESIAN_POINT('',(413.999456970946,326.974143289246,445.00000055189));
#60054=CARTESIAN_POINT('',(413.999456970946,326.19984729623,446.34112055189));
#60055=CARTESIAN_POINT('',(413.999456970946,326.974143289246,445.00000055189));
#60056=CARTESIAN_POINT('',(413.105376970946,326.19984729623,446.34112055189));
#60057=CARTESIAN_POINT('',(413.105376970946,326.974143289246,445.00000055189));
#60058=CARTESIAN_POINT('Origin',(414.017338570946,326.586995292738,444.32944055189));
#60059=CARTESIAN_POINT('',(413.999456970946,326.19984729623,443.65888055189));
#60060=CARTESIAN_POINT('',(413.999456970946,326.19984729623,443.65888055189));
#60061=CARTESIAN_POINT('',(413.105376970946,326.19984729623,443.65888055189));
#60062=CARTESIAN_POINT('Origin',(414.017338570946,325.425551303215,443.65888055189));
#60063=CARTESIAN_POINT('',(413.999456970946,324.651255310199,443.65888055189));
#60064=CARTESIAN_POINT('',(413.105376970946,324.651255310199,443.65888055189));
#60065=CARTESIAN_POINT('',(413.999456970946,326.19984729623,443.65888055189));
#60066=CARTESIAN_POINT('Origin',(414.017338570946,324.264107313692,444.32944055189));
#60067=CARTESIAN_POINT('',(413.999456970946,323.876959317184,445.00000055189));
#60068=CARTESIAN_POINT('',(413.999456970946,323.876959317184,445.00000055189));
#60069=CARTESIAN_POINT('',(413.105376970946,323.876959317184,445.00000055189));
#60070=CARTESIAN_POINT('Origin',(414.017338570946,324.264107313692,445.67056055189));
#60071=CARTESIAN_POINT('',(413.999456970946,324.651255310199,446.34112055189));
#60072=CARTESIAN_POINT('',(413.999456970946,324.651255310199,446.34112055189));
#60073=CARTESIAN_POINT('',(413.105376970946,324.651255310199,446.34112055189));
#60074=CARTESIAN_POINT('Origin',(414.017338570946,325.425551303215,446.34112055189));
#60075=CARTESIAN_POINT('',(413.999456970946,326.19984729623,446.34112055189));
#60076=CARTESIAN_POINT('Origin',(355.674148170946,322.720959303211,411.325867815642));
#60077=CARTESIAN_POINT('',(357.567725598318,326.986821771622,410.232610378218));
#60078=CARTESIAN_POINT('Origin',(355.674148170946,325.425551303211,411.325867815642));
#60079=CARTESIAN_POINT('Origin',(355.973888490946,325.425551303211,411.845033278959));
#60080=CARTESIAN_POINT('',(358.370226366169,327.373892153973,410.538420363603));
#60081=CARTESIAN_POINT('',(353.103582997138,325.425551303211,413.579118330439));
#60082=CARTESIAN_POINT('Origin',(356.007192970946,325.425551303211,411.902718330439));
#60083=CARTESIAN_POINT('Origin',(356.007192970946,325.425551303211,411.902718330439));
#60084=CARTESIAN_POINT('',(358.289976289384,327.335185115738,410.507839365064));
#60085=CARTESIAN_POINT('Origin',(356.10125099401,325.425551303211,412.065631605245));
#60086=CARTESIAN_POINT('',(353.291699043265,325.425551303211,413.904944880051));
#60087=CARTESIAN_POINT('Ctrl Pts',(353.291699043265,325.425551303211,413.904944880051));
#60088=CARTESIAN_POINT('Ctrl Pts',(353.291699043265,325.004330608665,413.904944880051));
#60089=CARTESIAN_POINT('Ctrl Pts',(353.360762093389,324.555183834243,413.856113692485));
#60090=CARTESIAN_POINT('Ctrl Pts',(353.643146477605,323.729188378078,413.660750718005));
#60091=CARTESIAN_POINT('Ctrl Pts',(353.856660763807,323.352320991875,413.514577125536));
#60092=CARTESIAN_POINT('Ctrl Pts',(354.353438858032,322.757206995828,413.184794032729));
#60093=CARTESIAN_POINT('Ctrl Pts',(354.669916248831,322.499210926969,412.979213640235));
#60094=CARTESIAN_POINT('Ctrl Pts',(355.371290146867,322.156977028214,412.54203615688));
#60095=CARTESIAN_POINT('Ctrl Pts',(355.756401100623,322.072751303211,412.310773721906));
#60096=CARTESIAN_POINT('Ctrl Pts',(356.48597524127,322.072751303211,411.88955389541));
#60097=CARTESIAN_POINT('Ctrl Pts',(356.878809861776,322.156977028214,411.671669243669));
#60098=CARTESIAN_POINT('Ctrl Pts',(357.608103617342,322.499210926969,411.282850372095));
#60099=CARTESIAN_POINT('Ctrl Pts',(357.944380155161,322.757206995828,411.111563108187));
#60100=CARTESIAN_POINT('Ctrl Pts',(358.478369738383,323.352320991875,410.846232204948));
#60101=CARTESIAN_POINT('Ctrl Pts',(358.711716925925,323.729188378078,410.734410205261));
#60102=CARTESIAN_POINT('Ctrl Pts',(359.022098416891,324.555183834244,410.587539642138));
#60103=CARTESIAN_POINT('Ctrl Pts',(359.098918990882,325.004330608665,410.552144880051));
#60104=CARTESIAN_POINT('Ctrl Pts',(359.098918990882,325.846771997758,410.552144880051));
#60105=CARTESIAN_POINT('Ctrl Pts',(359.022098416891,326.295918772179,410.587539642138));
#60106=CARTESIAN_POINT('Ctrl Pts',(358.711716925925,327.121914228345,410.734410205261));
#60107=CARTESIAN_POINT('Ctrl Pts',(358.478369738383,327.498781614548,410.846232204948));
#60108=CARTESIAN_POINT('Ctrl Pts',(357.944380155161,328.093895610594,411.111563108187));
#60109=CARTESIAN_POINT('Ctrl Pts',(357.608103617341,328.351891679454,411.282850372095));
#60110=CARTESIAN_POINT('Ctrl Pts',(356.878809861776,328.694125578209,411.671669243669));
#60111=CARTESIAN_POINT('Ctrl Pts',(356.485975241269,328.778351303211,411.88955389541));
#60112=CARTESIAN_POINT('Ctrl Pts',(355.756401100623,328.778351303211,412.310773721906));
#60113=CARTESIAN_POINT('Ctrl Pts',(355.371290146867,328.694125578208,412.54203615688));
#60114=CARTESIAN_POINT('Ctrl Pts',(354.66991624883,328.351891679453,412.979213640235));
#60115=CARTESIAN_POINT('Ctrl Pts',(354.353438858032,328.093895610594,413.184794032729));
#60116=CARTESIAN_POINT('Ctrl Pts',(353.856660763806,327.498781614547,413.514577125536));
#60117=CARTESIAN_POINT('Ctrl Pts',(353.643146477605,327.121914228344,413.660750718005));
#60118=CARTESIAN_POINT('Ctrl Pts',(353.360762093389,326.295918772179,413.856113692485));
#60119=CARTESIAN_POINT('Ctrl Pts',(353.291699043265,325.846771997757,413.904944880051));
#60120=CARTESIAN_POINT('Ctrl Pts',(353.291699043265,325.425551303211,413.904944880051));
#60121=CARTESIAN_POINT('',(353.197641020201,325.425551303211,413.742031605245));
#60122=CARTESIAN_POINT('Origin',(367.928095722949,325.425551303212,432.550327568991));
#60123=CARTESIAN_POINT('',(365.545644264409,325.425551303212,433.918816276238));
#60124=CARTESIAN_POINT('',(365.988628751342,327.022151685719,433.663059063461));
#60125=CARTESIAN_POINT('Origin',(367.925055850946,325.425551303212,432.545062356238));
#60126=CARTESIAN_POINT('Origin',(367.925055850946,325.425551303212,432.545062356238));
#60127=CARTESIAN_POINT('',(366.061877143581,326.986821771622,433.690971921189));
#60128=CARTESIAN_POINT('',(365.99595359057,327.018618694307,433.665850349235));
#60129=CARTESIAN_POINT('Origin',(367.955454570946,325.425551303212,432.597714483763));
#60130=CARTESIAN_POINT('Origin',(367.955454570946,322.720959303212,432.597714483763));
#60131=CARTESIAN_POINT('Origin',(413.999456970946,322.720959303215,445.00000055189));
#60132=CARTESIAN_POINT('',(413.999456970946,326.986821771626,447.18651542674));
#60133=CARTESIAN_POINT('Origin',(413.999456970946,325.425551303215,445.00000055189));
#60134=CARTESIAN_POINT('Origin',(413.399976330946,325.425551303215,445.00000055189));
#60135=CARTESIAN_POINT('',(413.333367370946,327.373892153977,447.728596485562));
#60136=CARTESIAN_POINT('',(413.333367370946,325.425551303215,441.64720055189));
#60137=CARTESIAN_POINT('Origin',(413.333367370946,325.425551303215,445.00000055189));
#60138=CARTESIAN_POINT('Origin',(413.333367370946,325.425551303215,445.00000055189));
#60139=CARTESIAN_POINT('',(413.399976330946,327.335185115742,447.67438837968));
#60140=CARTESIAN_POINT('Origin',(413.105376970957,167.573893717184,445.000000551892));
#60141=CARTESIAN_POINT('',(413.105376970957,169.914663296231,446.341120551892));
#60142=CARTESIAN_POINT('',(413.105376970957,168.3660713102,446.341120551892));
#60143=CARTESIAN_POINT('',(413.105376970957,169.914663296231,446.341120551892));
#60144=CARTESIAN_POINT('',(413.105376970957,167.591775317184,445.000000551892));
#60145=CARTESIAN_POINT('',(413.105376970957,168.3660713102,446.341120551892));
#60146=CARTESIAN_POINT('',(413.105376970957,168.3660713102,443.658880551892));
#60147=CARTESIAN_POINT('',(413.105376970957,167.591775317184,445.000000551892));
#60148=CARTESIAN_POINT('',(413.105376970957,169.914663296231,443.658880551892));
#60149=CARTESIAN_POINT('',(413.105376970957,168.3660713102,443.658880551892));
#60150=CARTESIAN_POINT('',(413.105376970957,170.688959289246,445.000000551892));
#60151=CARTESIAN_POINT('',(413.105376970957,169.914663296231,443.658880551892));
#60152=CARTESIAN_POINT('',(413.105376970957,170.688959289246,445.000000551892));
#60153=CARTESIAN_POINT('Origin',(414.017338570957,170.301811292738,445.670560551892));
#60154=CARTESIAN_POINT('',(413.999456970957,170.688959289246,445.000000551892));
#60155=CARTESIAN_POINT('',(413.999456970957,169.914663296231,446.341120551892));
#60156=CARTESIAN_POINT('',(413.999456970957,170.688959289246,445.000000551892));
#60157=CARTESIAN_POINT('',(413.105376970957,169.914663296231,446.341120551892));
#60158=CARTESIAN_POINT('',(413.105376970957,170.688959289246,445.000000551892));
#60159=CARTESIAN_POINT('Origin',(414.017338570957,170.301811292738,444.329440551892));
#60160=CARTESIAN_POINT('',(413.999456970957,169.914663296231,443.658880551892));
#60161=CARTESIAN_POINT('',(413.999456970957,169.914663296231,443.658880551892));
#60162=CARTESIAN_POINT('',(413.105376970957,169.914663296231,443.658880551892));
#60163=CARTESIAN_POINT('Origin',(414.017338570957,169.140367303215,443.658880551892));
#60164=CARTESIAN_POINT('',(413.999456970957,168.3660713102,443.658880551892));
#60165=CARTESIAN_POINT('',(413.105376970957,168.3660713102,443.658880551892));
#60166=CARTESIAN_POINT('',(413.999456970957,169.914663296231,443.658880551892));
#60167=CARTESIAN_POINT('Origin',(414.017338570957,167.978923313692,444.329440551892));
#60168=CARTESIAN_POINT('',(413.999456970957,167.591775317184,445.000000551892));
#60169=CARTESIAN_POINT('',(413.999456970957,167.591775317184,445.000000551892));
#60170=CARTESIAN_POINT('',(413.105376970957,167.591775317184,445.000000551892));
#60171=CARTESIAN_POINT('Origin',(414.017338570957,167.978923313692,445.670560551892));
#60172=CARTESIAN_POINT('',(413.999456970957,168.3660713102,446.341120551892));
#60173=CARTESIAN_POINT('',(413.999456970957,168.3660713102,446.341120551892));
#60174=CARTESIAN_POINT('',(413.105376970957,168.3660713102,446.341120551892));
#60175=CARTESIAN_POINT('Origin',(414.017338570957,169.140367303215,446.341120551892));
#60176=CARTESIAN_POINT('',(413.999456970957,169.914663296231,446.341120551892));
#60177=CARTESIAN_POINT('Origin',(356.121188170957,167.57389371718,477.899837295124));
#60178=CARTESIAN_POINT('',(354.959744181434,169.914663296227,477.229277295124));
#60179=CARTESIAN_POINT('',(354.959744181434,168.366071310196,477.229277295124));
#60180=CARTESIAN_POINT('',(354.959744181434,169.914663296227,477.229277295124));
#60181=CARTESIAN_POINT('',(356.121188170957,167.59177531718,477.899837295124));
#60182=CARTESIAN_POINT('',(354.959744181434,168.366071310196,477.229277295124));
#60183=CARTESIAN_POINT('',(357.28263216048,168.366071310196,478.570397295124));
#60184=CARTESIAN_POINT('',(356.121188170957,167.59177531718,477.899837295124));
#60185=CARTESIAN_POINT('',(357.28263216048,169.914663296227,478.570397295124));
#60186=CARTESIAN_POINT('',(357.28263216048,168.366071310196,478.570397295124));
#60187=CARTESIAN_POINT('',(356.121188170957,170.688959289243,477.899837295124));
#60188=CARTESIAN_POINT('',(357.28263216048,169.914663296227,478.570397295124));
#60189=CARTESIAN_POINT('',(356.121188170957,170.688959289243,477.899837295124));
#60190=CARTESIAN_POINT('Origin',(355.402364199503,170.130975246119,477.211963510373));
#60191=CARTESIAN_POINT('',(355.674148170957,170.688959289243,478.67413328814));
#60192=CARTESIAN_POINT('',(354.512704181433,169.914663296227,478.00357328814));
#60193=CARTESIAN_POINT('',(355.674148170957,170.688959289243,478.67413328814));
#60194=CARTESIAN_POINT('',(354.959744181434,169.914663296227,477.229277295124));
#60195=CARTESIAN_POINT('',(356.121188170957,170.688959289243,477.899837295124));
#60196=CARTESIAN_POINT('Origin',(356.563808189027,170.472647339351,477.882523510373));
#60197=CARTESIAN_POINT('',(356.83559216048,169.914663296227,479.34469328814));
#60198=CARTESIAN_POINT('',(356.83559216048,169.914663296227,479.34469328814));
#60199=CARTESIAN_POINT('',(357.28263216048,169.914663296227,478.570397295124));
#60200=CARTESIAN_POINT('Origin',(357.05911216048,168.348189710196,478.957545291632));
#60201=CARTESIAN_POINT('',(356.83559216048,168.366071310196,479.34469328814));
#60202=CARTESIAN_POINT('',(357.28263216048,168.366071310196,478.570397295124));
#60203=CARTESIAN_POINT('',(356.83559216048,169.914663296227,479.34469328814));
#60204=CARTESIAN_POINT('Origin',(356.563808189027,167.808087267072,477.882523510373));
#60205=CARTESIAN_POINT('',(355.674148170957,167.59177531718,478.67413328814));
#60206=CARTESIAN_POINT('',(355.674148170957,167.59177531718,478.67413328814));
#60207=CARTESIAN_POINT('',(356.121188170957,167.59177531718,477.899837295124));
#60208=CARTESIAN_POINT('Origin',(355.402364199503,168.149759360304,477.211963510373));
#60209=CARTESIAN_POINT('',(354.512704181434,168.366071310196,478.00357328814));
#60210=CARTESIAN_POINT('',(354.512704181434,168.366071310196,478.00357328814));
#60211=CARTESIAN_POINT('',(354.959744181434,168.366071310196,477.229277295124));
#60212=CARTESIAN_POINT('Origin',(354.736224181434,168.348189710196,477.616425291632));
#60213=CARTESIAN_POINT('',(354.512704181433,169.914663296227,478.00357328814));
#60214=CARTESIAN_POINT('Origin',(355.674148170957,166.435775303211,478.67413328814));
#60215=CARTESIAN_POINT('',(353.780570743585,170.701637771622,477.580875850715));
#60216=CARTESIAN_POINT('Origin',(355.674148170957,169.140367303211,478.67413328814));
#60217=CARTESIAN_POINT('Origin',(355.973888490957,169.140367303211,478.154967824823));
#60218=CARTESIAN_POINT('',(353.644159575734,171.088708153973,476.732984806507));
#60219=CARTESIAN_POINT('',(358.910802944765,169.140367303212,479.773682773344));
#60220=CARTESIAN_POINT('Origin',(356.007192970957,169.140367303212,478.097282773343));
#60221=CARTESIAN_POINT('Origin',(356.007192970957,169.140367303212,478.097282773343));
#60222=CARTESIAN_POINT('',(353.657800692519,171.050001115738,476.817773910928));
#60223=CARTESIAN_POINT('Origin',(356.10125099402,169.140367303212,477.934369498538));
#60224=CARTESIAN_POINT('',(359.098918990893,169.140367303212,479.447856223731));
#60225=CARTESIAN_POINT('Ctrl Pts',(359.098918990893,169.140367303212,479.447856223731));
#60226=CARTESIAN_POINT('Ctrl Pts',(359.098918990893,168.719146608665,479.447856223731));
#60227=CARTESIAN_POINT('Ctrl Pts',(359.022098416902,168.269999834244,479.412461461645));
#60228=CARTESIAN_POINT('Ctrl Pts',(358.711716925936,167.444004378079,479.265590898522));
#60229=CARTESIAN_POINT('Ctrl Pts',(358.478369738394,167.067136991875,479.153768898834));
#60230=CARTESIAN_POINT('Ctrl Pts',(357.944380155172,166.472022995829,478.888437995595));
#60231=CARTESIAN_POINT('Ctrl Pts',(357.608103617353,166.214026926969,478.717150731687));
#60232=CARTESIAN_POINT('Ctrl Pts',(356.878809861787,165.871793028214,478.328331860114));
#60233=CARTESIAN_POINT('Ctrl Pts',(356.48597524128,165.787567303211,478.110447208372));
#60234=CARTESIAN_POINT('Ctrl Pts',(355.756401100634,165.787567303211,477.689227381876));
#60235=CARTESIAN_POINT('Ctrl Pts',(355.371290146878,165.871793028214,477.457964946902));
#60236=CARTESIAN_POINT('Ctrl Pts',(354.669916248842,166.214026926969,477.020787463548));
#60237=CARTESIAN_POINT('Ctrl Pts',(354.353438858043,166.472022995828,476.815207071053));
#60238=CARTESIAN_POINT('Ctrl Pts',(353.856660763817,167.067136991875,476.485423978246));
#60239=CARTESIAN_POINT('Ctrl Pts',(353.643146477615,167.444004378078,476.339250385777));
#60240=CARTESIAN_POINT('Ctrl Pts',(353.3607620934,168.269999834243,476.143887411298));
#60241=CARTESIAN_POINT('Ctrl Pts',(353.291699043276,168.719146608665,476.095056223732));
#60242=CARTESIAN_POINT('Ctrl Pts',(353.291699043276,169.561587997758,476.095056223732));
#60243=CARTESIAN_POINT('Ctrl Pts',(353.3607620934,170.010734772179,476.143887411298));
#60244=CARTESIAN_POINT('Ctrl Pts',(353.643146477615,170.836730228344,476.339250385777));
#60245=CARTESIAN_POINT('Ctrl Pts',(353.856660763817,171.213597614548,476.485423978246));
#60246=CARTESIAN_POINT('Ctrl Pts',(354.353438858043,171.808711610594,476.815207071053));
#60247=CARTESIAN_POINT('Ctrl Pts',(354.669916248841,172.066707679454,477.020787463548));
#60248=CARTESIAN_POINT('Ctrl Pts',(355.371290146877,172.408941578209,477.457964946902));
#60249=CARTESIAN_POINT('Ctrl Pts',(355.756401100633,172.493167303211,477.689227381876));
#60250=CARTESIAN_POINT('Ctrl Pts',(356.48597524128,172.493167303212,478.110447208372));
#60251=CARTESIAN_POINT('Ctrl Pts',(356.878809861787,172.408941578209,478.328331860114));
#60252=CARTESIAN_POINT('Ctrl Pts',(357.608103617352,172.066707679454,478.717150731687));
#60253=CARTESIAN_POINT('Ctrl Pts',(357.944380155172,171.808711610595,478.888437995595));
#60254=CARTESIAN_POINT('Ctrl Pts',(358.478369738394,171.213597614548,479.153768898834));
#60255=CARTESIAN_POINT('Ctrl Pts',(358.711716925935,170.836730228345,479.265590898522));
#60256=CARTESIAN_POINT('Ctrl Pts',(359.022098416902,170.010734772179,479.412461461645));
#60257=CARTESIAN_POINT('Ctrl Pts',(359.098918990893,169.561587997758,479.447856223732));
#60258=CARTESIAN_POINT('Ctrl Pts',(359.098918990893,169.140367303212,479.447856223732));
#60259=CARTESIAN_POINT('',(359.004860967829,169.140367303212,479.610769498538));
#60260=CARTESIAN_POINT('Origin',(367.928095722957,169.140367303212,457.449673534792));
#60261=CARTESIAN_POINT('',(370.304467437494,169.140367303212,458.828692667544));
#60262=CARTESIAN_POINT('',(369.861482950562,170.736967685717,458.572935454769));
#60263=CARTESIAN_POINT('Origin',(367.925055850957,169.140367303212,457.454938747544));
#60264=CARTESIAN_POINT('Origin',(367.925055850957,169.140367303212,457.454938747544));
#60265=CARTESIAN_POINT('',(369.849031998329,170.701637771622,458.495544057444));
#60266=CARTESIAN_POINT('',(369.860237855339,170.733434694307,458.565196315036));
#60267=CARTESIAN_POINT('Origin',(367.955454570957,169.140367303212,457.402286620019));
#60268=CARTESIAN_POINT('Origin',(367.955454570957,166.435775303212,457.402286620019));
#60269=CARTESIAN_POINT('Origin',(413.999456970957,166.435775303215,445.000000551892));
#60270=CARTESIAN_POINT('',(413.999456970957,170.701637771626,447.186515426741));
#60271=CARTESIAN_POINT('Origin',(413.999456970957,169.140367303215,445.000000551892));
#60272=CARTESIAN_POINT('Origin',(413.399976330957,169.140367303215,445.000000551892));
#60273=CARTESIAN_POINT('',(413.333367370957,171.088708153977,447.728596485564));
#60274=CARTESIAN_POINT('',(413.333367370957,169.140367303215,441.647200551892));
#60275=CARTESIAN_POINT('Origin',(413.333367370957,169.140367303215,445.000000551892));
#60276=CARTESIAN_POINT('Origin',(413.333367370957,169.140367303215,445.000000551892));
#60277=CARTESIAN_POINT('',(413.399976330957,171.050001115742,447.674388379681));
#60278=CARTESIAN_POINT('Origin',(413.145251324829,169.140367303215,445.000000551892));
#60279=CARTESIAN_POINT('',(412.957135278702,169.140367303215,441.647200551892));
#60280=CARTESIAN_POINT('Ctrl Pts',(412.957135278702,169.140367303215,441.647200551892));
#60281=CARTESIAN_POINT('Ctrl Pts',(412.957135278702,168.719146608669,441.647200551892));
#60282=CARTESIAN_POINT('Ctrl Pts',(412.964892802569,168.269999834247,441.731426501545));
#60283=CARTESIAN_POINT('Ctrl Pts',(412.99288990932,167.444004378082,442.073660039147));
#60284=CARTESIAN_POINT('Ctrl Pts',(413.012722810659,167.067136991879,442.331655631304));
#60285=CARTESIAN_POINT('Ctrl Pts',(413.049934299656,166.472022995832,442.92676962735));
#60286=CARTESIAN_POINT('Ctrl Pts',(413.069733446677,166.214026926973,443.303637283752));
#60287=CARTESIAN_POINT('Ctrl Pts',(413.097653304206,165.871793028218,444.12963363868));
#60288=CARTESIAN_POINT('Ctrl Pts',(413.105376970957,165.787567303215,444.578780725396));
#60289=CARTESIAN_POINT('Ctrl Pts',(413.105376970957,165.787567303215,445.421220378388));
#60290=CARTESIAN_POINT('Ctrl Pts',(413.097653304206,165.871793028218,445.870367465103));
#60291=CARTESIAN_POINT('Ctrl Pts',(413.069733446677,166.214026926973,446.696363820031));
#60292=CARTESIAN_POINT('Ctrl Pts',(413.049934299656,166.472022995832,447.073231476433));
#60293=CARTESIAN_POINT('Ctrl Pts',(413.012722810659,167.067136991879,447.66834547248));
#60294=CARTESIAN_POINT('Ctrl Pts',(412.99288990932,167.444004378082,447.926341064636));
#60295=CARTESIAN_POINT('Ctrl Pts',(412.964892802569,168.269999834247,448.268574602239));
#60296=CARTESIAN_POINT('Ctrl Pts',(412.957135278702,168.719146608669,448.352800551892));
#60297=CARTESIAN_POINT('Ctrl Pts',(412.957135278702,169.561587997761,448.352800551892));
#60298=CARTESIAN_POINT('Ctrl Pts',(412.964892802569,170.010734772183,448.268574602239));
#60299=CARTESIAN_POINT('Ctrl Pts',(412.992889909319,170.836730228348,447.926341064636));
#60300=CARTESIAN_POINT('Ctrl Pts',(413.012722810659,171.213597614551,447.66834547248));
#60301=CARTESIAN_POINT('Ctrl Pts',(413.049934299656,171.808711610598,447.073231476433));
#60302=CARTESIAN_POINT('Ctrl Pts',(413.069733446677,172.066707679457,446.696363820031));
#60303=CARTESIAN_POINT('Ctrl Pts',(413.097653304206,172.408941578212,445.870367465103));
#60304=CARTESIAN_POINT('Ctrl Pts',(413.105376970957,172.493167303215,445.421220378388));
#60305=CARTESIAN_POINT('Ctrl Pts',(413.105376970957,172.493167303215,444.578780725396));
#60306=CARTESIAN_POINT('Ctrl Pts',(413.097653304206,172.408941578212,444.12963363868));
#60307=CARTESIAN_POINT('Ctrl Pts',(413.069733446677,172.066707679457,443.303637283752));
#60308=CARTESIAN_POINT('Ctrl Pts',(413.049934299656,171.808711610598,442.92676962735));
#60309=CARTESIAN_POINT('Ctrl Pts',(413.012722810659,171.213597614551,442.331655631304));
#60310=CARTESIAN_POINT('Ctrl Pts',(412.992889909319,170.836730228348,442.073660039147));
#60311=CARTESIAN_POINT('Ctrl Pts',(412.964892802569,170.010734772183,441.731426501545));
#60312=CARTESIAN_POINT('Ctrl Pts',(412.957135278702,169.561587997761,441.647200551892));
#60313=CARTESIAN_POINT('Ctrl Pts',(412.957135278702,169.140367303215,441.647200551892));
#60314=CARTESIAN_POINT('',(413.145251324829,169.140367303215,441.647200551892));
#60315=CARTESIAN_POINT('Origin',(392.589549066957,169.140367303214,445.000000551892));
#60316=CARTESIAN_POINT('',(392.534831370957,170.701637771624,442.813485677043));
#60317=CARTESIAN_POINT('',(392.589549066957,170.733434694309,442.768954991405));
#60318=CARTESIAN_POINT('Origin',(392.534831370957,169.140367303214,445.000000551892));
#60319=CARTESIAN_POINT('Origin',(392.534831370957,166.435775303214,445.000000551892));
#60320=CARTESIAN_POINT('Origin',(368.234803806253,169.140367303212,456.91843955143));
#60321=CARTESIAN_POINT('',(370.61421539279,169.140367303212,458.29219347143));
#60322=CARTESIAN_POINT('Origin',(368.234803806243,325.425551303212,433.081561552353));
#60323=CARTESIAN_POINT('',(365.855392219706,325.425551303212,434.455315472353));
#60324=CARTESIAN_POINT('Origin',(392.534831370946,322.720959303214,445.00000055189));
#60325=CARTESIAN_POINT('',(392.534831370946,326.986821771625,442.813485677041));
#60326=CARTESIAN_POINT('Origin',(392.534831370946,325.425551303214,445.00000055189));
#60327=CARTESIAN_POINT('Origin',(392.589549066946,325.425551303214,445.00000055189));
#60328=CARTESIAN_POINT('',(392.589549066946,327.018618694309,442.768954991404));
#60329=CARTESIAN_POINT('Origin',(413.145251324819,325.425551303215,445.00000055189));
#60330=CARTESIAN_POINT('',(412.957135278691,325.425551303215,441.64720055189));
#60331=CARTESIAN_POINT('Ctrl Pts',(412.957135278691,325.425551303215,441.64720055189));
#60332=CARTESIAN_POINT('Ctrl Pts',(412.957135278691,325.004330608669,441.64720055189));
#60333=CARTESIAN_POINT('Ctrl Pts',(412.964892802559,324.555183834248,441.731426501543));
#60334=CARTESIAN_POINT('Ctrl Pts',(412.992889909309,323.729188378082,442.073660039146));
#60335=CARTESIAN_POINT('Ctrl Pts',(413.012722810649,323.352320991879,442.331655631302));
#60336=CARTESIAN_POINT('Ctrl Pts',(413.049934299646,322.757206995832,442.926769627349));
#60337=CARTESIAN_POINT('Ctrl Pts',(413.069733446666,322.499210926973,443.303637283751));
#60338=CARTESIAN_POINT('Ctrl Pts',(413.097653304196,322.156977028218,444.129633638679));
#60339=CARTESIAN_POINT('Ctrl Pts',(413.105376970947,322.072751303215,444.578780725394));
#60340=CARTESIAN_POINT('Ctrl Pts',(413.105376970947,322.072751303215,445.421220378386));
#60341=CARTESIAN_POINT('Ctrl Pts',(413.097653304196,322.156977028218,445.870367465102));
#60342=CARTESIAN_POINT('Ctrl Pts',(413.069733446666,322.499210926973,446.69636382003));
#60343=CARTESIAN_POINT('Ctrl Pts',(413.049934299646,322.757206995832,447.073231476432));
#60344=CARTESIAN_POINT('Ctrl Pts',(413.012722810649,323.352320991879,447.668345472478));
#60345=CARTESIAN_POINT('Ctrl Pts',(412.992889909309,323.729188378082,447.926341064635));
#60346=CARTESIAN_POINT('Ctrl Pts',(412.964892802559,324.555183834248,448.268574602237));
#60347=CARTESIAN_POINT('Ctrl Pts',(412.957135278691,325.004330608669,448.35280055189));
#60348=CARTESIAN_POINT('Ctrl Pts',(412.957135278691,325.846771997762,448.35280055189));
#60349=CARTESIAN_POINT('Ctrl Pts',(412.964892802559,326.295918772183,448.268574602237));
#60350=CARTESIAN_POINT('Ctrl Pts',(412.992889909309,327.121914228348,447.926341064635));
#60351=CARTESIAN_POINT('Ctrl Pts',(413.012722810649,327.498781614552,447.668345472478));
#60352=CARTESIAN_POINT('Ctrl Pts',(413.049934299645,328.093895610598,447.073231476432));
#60353=CARTESIAN_POINT('Ctrl Pts',(413.069733446666,328.351891679458,446.69636382003));
#60354=CARTESIAN_POINT('Ctrl Pts',(413.097653304195,328.694125578213,445.870367465102));
#60355=CARTESIAN_POINT('Ctrl Pts',(413.105376970946,328.778351303215,445.421220378386));
#60356=CARTESIAN_POINT('Ctrl Pts',(413.105376970946,328.778351303215,444.578780725394));
#60357=CARTESIAN_POINT('Ctrl Pts',(413.097653304195,328.694125578213,444.129633638679));
#60358=CARTESIAN_POINT('Ctrl Pts',(413.069733446666,328.351891679458,443.303637283751));
#60359=CARTESIAN_POINT('Ctrl Pts',(413.049934299645,328.093895610598,442.926769627349));
#60360=CARTESIAN_POINT('Ctrl Pts',(413.012722810649,327.498781614552,442.331655631302));
#60361=CARTESIAN_POINT('Ctrl Pts',(412.992889909309,327.121914228348,442.073660039146));
#60362=CARTESIAN_POINT('Ctrl Pts',(412.964892802559,326.295918772183,441.731426501543));
#60363=CARTESIAN_POINT('Ctrl Pts',(412.957135278691,325.846771997762,441.64720055189));
#60364=CARTESIAN_POINT('Ctrl Pts',(412.957135278691,325.425551303215,441.64720055189));
#60365=CARTESIAN_POINT('',(413.145251324819,325.425551303215,441.64720055189));
#60366=CARTESIAN_POINT('Origin',(375.115917770957,168.514511303212,445.000000551892));
#60367=CARTESIAN_POINT('',(375.115917770957,163.418255303212,407.010541351892));
#60368=CARTESIAN_POINT('',(353.039917037922,163.418255303211,414.083189559432));
#60369=CARTESIAN_POINT('Origin',(375.115917770957,163.418255303212,445.000000551892));
#60370=CARTESIAN_POINT('Origin',(375.115917770957,163.418255303212,445.000000551892));
#60371=CARTESIAN_POINT('',(375.115917770956,173.610767303212,407.010541351892));
#60372=CARTESIAN_POINT('',(375.115917770957,168.514511303212,407.010541351892));
#60373=CARTESIAN_POINT('Origin',(375.115917770956,173.610767303212,445.000000551892));
#60374=CARTESIAN_POINT('Origin',(375.115917770957,161.810965703212,445.000000551892));
#60375=CARTESIAN_POINT('',(353.579167835194,161.810965703211,414.838394960011));
#60376=CARTESIAN_POINT('Origin',(391.658632970951,247.282959303214,448.361741351891));
#60377=CARTESIAN_POINT('Ctrl Pts',(388.115106324202,164.491151303213,448.361741351892));
#60378=CARTESIAN_POINT('Ctrl Pts',(388.541335653383,163.776414442266,448.361741351892));
#60379=CARTESIAN_POINT('Ctrl Pts',(388.966604868594,163.061101141136,448.361741351892));
#60380=CARTESIAN_POINT('Ctrl Pts',(389.391142518198,162.345359303214,448.361741351892));
#60381=CARTESIAN_POINT('Origin',(375.115917770957,164.276572103213,445.000000551892));
#60382=CARTESIAN_POINT('Ctrl Pts',(389.391142518198,162.345359303214,441.638259751892));
#60383=CARTESIAN_POINT('Ctrl Pts',(388.966603199882,163.061103954472,441.638259751892));
#60384=CARTESIAN_POINT('Ctrl Pts',(388.541330836671,163.776422519329,441.638259751892));
#60385=CARTESIAN_POINT('Ctrl Pts',(388.115106324202,164.491151303213,441.638259751892));
#60386=CARTESIAN_POINT('Origin',(391.658632970951,247.282959303214,441.638259751891));
#60387=CARTESIAN_POINT('Origin',(375.115917770946,325.988821703213,445.00000055189));
#60388=CARTESIAN_POINT('',(375.115917770946,320.829980103212,407.01054135189));
#60389=CARTESIAN_POINT('Origin',(375.115917770947,320.829980103212,445.000000551891));
#60390=CARTESIAN_POINT('',(375.115917770946,325.988821703212,407.01054135189));
#60391=CARTESIAN_POINT('Origin',(422.081940170956,183.445647303215,445.000000551892));
#60392=CARTESIAN_POINT('',(375.115917770956,183.445647303212,407.010541351892));
#60393=CARTESIAN_POINT('Origin',(375.115917770956,183.445647303212,445.000000551892));
#60394=CARTESIAN_POINT('Origin',(422.081940170956,173.610767303215,445.000000551892));
#60395=CARTESIAN_POINT('',(375.115917770957,173.610767303213,491.948141351892));
#60396=CARTESIAN_POINT('Origin',(375.115917770956,173.610767303212,445.000000551892));
#60397=CARTESIAN_POINT('Origin',(375.115917770956,174.057807303212,445.000000551892));
#60398=CARTESIAN_POINT('',(375.115917770957,174.057807303213,491.948141351892));
#60399=CARTESIAN_POINT('Origin',(375.115917770951,247.220373703212,445.000000551891));
#60400=CARTESIAN_POINT('',(375.115917770947,310.995100103212,407.01054135189));
#60401=CARTESIAN_POINT('',(375.115917770951,247.220373703212,407.010541351891));
#60402=CARTESIAN_POINT('Origin',(375.115917770947,310.995100103212,445.000000551891));
#60403=CARTESIAN_POINT('Origin',(328.149895370947,310.995100103209,445.000000551891));
#60404=CARTESIAN_POINT('Origin',(328.149895370946,320.829980103209,445.000000551891));
#60405=CARTESIAN_POINT('',(375.115917770947,320.829980103213,491.94814135189));
#60406=CARTESIAN_POINT('Origin',(375.115917770947,320.829980103212,445.00000055189));
#60407=CARTESIAN_POINT('Origin',(375.115917770947,320.382940103212,445.00000055189));
#60408=CARTESIAN_POINT('',(375.115917770947,320.382940103213,491.94814135189));
#60409=CARTESIAN_POINT('Origin',(328.660166744143,326.48056570321,497.549298322233));
#60410=CARTESIAN_POINT('',(317.315530368861,326.480565703209,499.630144284955));
#60411=CARTESIAN_POINT('',(317.315530368861,326.480565703209,495.46845235951));
#60412=CARTESIAN_POINT('Origin',(322.566620000601,326.48056570321,497.549298322233));
#60413=CARTESIAN_POINT('',(318.139009719652,326.480565703209,501.05645235951));
#60414=CARTESIAN_POINT('',(318.139009719652,326.480565703209,501.05645235951));
#60415=CARTESIAN_POINT('',(321.743140649812,326.48056570321,503.137298322233));
#60416=CARTESIAN_POINT('Origin',(322.566620000605,326.48056570321,497.549298322231));
#60417=CARTESIAN_POINT('',(323.390099351396,326.48056570321,503.137298322233));
#60418=CARTESIAN_POINT('',(323.390099351396,326.48056570321,503.137298322233));
#60419=CARTESIAN_POINT('',(326.994230281556,326.48056570321,501.05645235951));
#60420=CARTESIAN_POINT('Origin',(322.566620000604,326.48056570321,497.549298322233));
#60421=CARTESIAN_POINT('',(327.817709632347,326.48056570321,499.630144284955));
#60422=CARTESIAN_POINT('',(327.817709632347,326.48056570321,499.630144284955));
#60423=CARTESIAN_POINT('',(327.817709632347,326.48056570321,495.46845235951));
#60424=CARTESIAN_POINT('Origin',(322.566620000604,326.48056570321,497.549298322233));
#60425=CARTESIAN_POINT('',(326.994230281556,326.48056570321,494.042144284955));
#60426=CARTESIAN_POINT('',(326.994230281556,326.48056570321,494.042144284955));
#60427=CARTESIAN_POINT('',(323.390099351396,326.48056570321,491.961298322233));
#60428=CARTESIAN_POINT('Origin',(322.566620000604,326.48056570321,497.549298322233));
#60429=CARTESIAN_POINT('',(321.743140649812,326.48056570321,491.961298322233));
#60430=CARTESIAN_POINT('',(321.743140649812,326.48056570321,491.961298322233));
#60431=CARTESIAN_POINT('',(318.139009719652,326.480565703209,494.042144284955));
#60432=CARTESIAN_POINT('Origin',(322.566620000605,326.48056570321,497.549298322235));
#60433=CARTESIAN_POINT('',(317.315530368861,326.480565703209,495.46845235951));
#60434=CARTESIAN_POINT('Origin',(322.566620000609,326.062734664725,497.549298322235));
#60435=CARTESIAN_POINT('',(319.340386696372,326.016308993793,491.961298322233));
#60436=CARTESIAN_POINT('Ctrl Pts',(319.340386696347,326.016308993785,491.961298322233));
#60437=CARTESIAN_POINT('Ctrl Pts',(320.621596852842,326.386162508159,491.961298322233));
#60438=CARTESIAN_POINT('Ctrl Pts',(321.743140649817,326.48056570321,491.961298322233));
#60439=CARTESIAN_POINT('Ctrl Pts',(318.13900971965,326.480565703209,494.042144284959));
#60440=CARTESIAN_POINT('Ctrl Pts',(318.699781618137,326.386162508158,493.070858865322));
#60441=CARTESIAN_POINT('Ctrl Pts',(319.340386696385,326.016308993785,491.961298322211));
#60442=CARTESIAN_POINT('Origin',(325.810734904862,323.65527290321,503.137298322233));
#60443=CARTESIAN_POINT('',(325.792853304836,326.016308993794,503.137298322233));
#60444=CARTESIAN_POINT('Ctrl Pts',(325.792853304861,326.016308993786,503.137298322233));
#60445=CARTESIAN_POINT('Ctrl Pts',(324.511643148366,326.386162508159,503.137298322233));
#60446=CARTESIAN_POINT('Ctrl Pts',(323.390099351391,326.48056570321,503.137298322233));
#60447=CARTESIAN_POINT('',(319.340386696372,326.016308993794,503.137298322233));
#60448=CARTESIAN_POINT('Ctrl Pts',(321.743140649817,326.48056570321,503.137298322233));
#60449=CARTESIAN_POINT('Ctrl Pts',(320.621596852842,326.386162508159,503.137298322233));
#60450=CARTESIAN_POINT('Ctrl Pts',(319.340386696347,326.016308993786,503.137298322233));
#60451=CARTESIAN_POINT('',(319.340386696372,326.016308993794,503.137298322233));
#60452=CARTESIAN_POINT('',(325.792853304836,326.016308993794,503.137298322233));
#60453=CARTESIAN_POINT('Origin',(327.405969956952,326.49844730321,500.343298322233));
#60454=CARTESIAN_POINT('',(329.019086609067,326.016308993794,497.549298322233));
#60455=CARTESIAN_POINT('Ctrl Pts',(329.01908660908,326.016308993786,497.549298322211));
#60456=CARTESIAN_POINT('Ctrl Pts',(328.378481530832,326.386162508159,498.658858865322));
#60457=CARTESIAN_POINT('Ctrl Pts',(327.817709632345,326.48056570321,499.630144284959));
#60458=CARTESIAN_POINT('Ctrl Pts',(326.994230281558,326.48056570321,501.056452359506));
#60459=CARTESIAN_POINT('Ctrl Pts',(326.433458383071,326.386162508159,502.027737779143));
#60460=CARTESIAN_POINT('Ctrl Pts',(325.792853304823,326.016308993786,503.137298322255));
#60461=CARTESIAN_POINT('',(329.019086609067,326.016308993794,497.549298322233));
#60462=CARTESIAN_POINT('Origin',(322.566620000604,326.062734664728,497.549298322233));
#60463=CARTESIAN_POINT('',(325.792853304836,326.016308993794,491.961298322233));
#60464=CARTESIAN_POINT('Ctrl Pts',(323.390099351391,326.48056570321,491.961298322233));
#60465=CARTESIAN_POINT('Ctrl Pts',(324.511643148366,326.386162508159,491.961298322233));
#60466=CARTESIAN_POINT('Ctrl Pts',(325.792853304861,326.016308993786,491.961298322233));
#60467=CARTESIAN_POINT('Ctrl Pts',(325.792853304823,326.016308993786,491.961298322211));
#60468=CARTESIAN_POINT('Ctrl Pts',(326.433458383071,326.386162508159,493.070858865322));
#60469=CARTESIAN_POINT('Ctrl Pts',(326.994230281558,326.48056570321,494.042144284959));
#60470=CARTESIAN_POINT('Origin',(322.566620000608,326.062734664731,497.549298322233));
#60471=CARTESIAN_POINT('Ctrl Pts',(327.817709632345,326.48056570321,495.468452359506));
#60472=CARTESIAN_POINT('Ctrl Pts',(328.378481530832,326.386162508159,496.439737779143));
#60473=CARTESIAN_POINT('Ctrl Pts',(329.01908660908,326.016308993786,497.549298322255));
#60474=CARTESIAN_POINT('Origin',(322.566620000601,326.062734664725,497.549298322228));
#60475=CARTESIAN_POINT('Origin',(322.5666200006,326.062734664732,497.549298322233));
#60476=CARTESIAN_POINT('',(316.114153392141,326.016308993793,497.549298322233));
#60477=CARTESIAN_POINT('Ctrl Pts',(317.315530368863,326.480565703209,499.630144284959));
#60478=CARTESIAN_POINT('Ctrl Pts',(316.754758470376,326.386162508158,498.658858865322));
#60479=CARTESIAN_POINT('Ctrl Pts',(316.114153392128,326.016308993785,497.549298322211));
#60480=CARTESIAN_POINT('Ctrl Pts',(316.114153392128,326.016308993785,497.549298322255));
#60481=CARTESIAN_POINT('Ctrl Pts',(316.754758470376,326.386162508158,496.439737779143));
#60482=CARTESIAN_POINT('Ctrl Pts',(317.315530368863,326.480565703209,495.468452359506));
#60483=CARTESIAN_POINT('Origin',(322.566620000606,326.06273466473,497.549298322236));
#60484=CARTESIAN_POINT('Ctrl Pts',(319.340386696385,326.016308993786,503.137298322255));
#60485=CARTESIAN_POINT('Ctrl Pts',(318.699781618137,326.386162508159,502.027737779143));
#60486=CARTESIAN_POINT('Ctrl Pts',(318.13900971965,326.480565703209,501.056452359506));
#60487=CARTESIAN_POINT('Origin',(317.727270044256,326.498447303209,500.343298322233));
#60488=CARTESIAN_POINT('',(316.114153392141,326.016308993793,497.549298322233));
#60489=CARTESIAN_POINT('Origin',(317.727270044256,326.498447303209,494.755298322233));
#60490=CARTESIAN_POINT('',(319.340386696372,326.016308993793,491.961298322233));
#60491=CARTESIAN_POINT('Origin',(325.810734904862,323.65527290321,491.961298322233));
#60492=CARTESIAN_POINT('',(325.792853304836,326.016308993794,491.961298322233));
#60493=CARTESIAN_POINT('Origin',(327.405969956952,326.49844730321,494.755298322233));
#60494=CARTESIAN_POINT('Origin',(433.758762284827,326.480565703216,392.450702781548));
#60495=CARTESIAN_POINT('',(422.414125909545,326.480565703216,394.531548744271));
#60496=CARTESIAN_POINT('',(422.414125909545,326.480565703216,390.369856818826));
#60497=CARTESIAN_POINT('Origin',(427.665215541288,326.480565703216,392.450702781548));
#60498=CARTESIAN_POINT('',(423.237605260337,326.480565703216,395.957856818826));
#60499=CARTESIAN_POINT('',(423.237605260337,326.480565703216,395.957856818826));
#60500=CARTESIAN_POINT('',(426.841736190497,326.480565703216,398.038702781548));
#60501=CARTESIAN_POINT('Origin',(427.665215541288,326.480565703216,392.450702781548));
#60502=CARTESIAN_POINT('',(428.48869489208,326.480565703216,398.038702781548));
#60503=CARTESIAN_POINT('',(428.48869489208,326.480565703216,398.038702781548));
#60504=CARTESIAN_POINT('',(432.09282582224,326.480565703216,395.957856818826));
#60505=CARTESIAN_POINT('Origin',(427.665215541288,326.480565703216,392.450702781548));
#60506=CARTESIAN_POINT('',(432.916305173032,326.480565703216,394.531548744271));
#60507=CARTESIAN_POINT('',(432.916305173032,326.480565703216,394.531548744271));
#60508=CARTESIAN_POINT('',(432.916305173032,326.480565703216,390.369856818826));
#60509=CARTESIAN_POINT('Origin',(427.665215541289,326.480565703216,392.450702781548));
#60510=CARTESIAN_POINT('',(432.09282582224,326.480565703216,388.943548744271));
#60511=CARTESIAN_POINT('',(432.09282582224,326.480565703216,388.943548744271));
#60512=CARTESIAN_POINT('',(428.48869489208,326.480565703216,386.862702781548));
#60513=CARTESIAN_POINT('Origin',(427.665215541288,326.480565703216,392.450702781548));
#60514=CARTESIAN_POINT('',(426.841736190497,326.480565703216,386.862702781548));
#60515=CARTESIAN_POINT('',(426.841736190497,326.480565703216,386.862702781548));
#60516=CARTESIAN_POINT('',(423.237605260337,326.480565703216,388.943548744271));
#60517=CARTESIAN_POINT('Origin',(427.665215541288,326.480565703216,392.450702781548));
#60518=CARTESIAN_POINT('',(422.414125909545,326.480565703216,390.369856818826));
#60519=CARTESIAN_POINT('Origin',(427.665215541288,326.062734664734,392.450702781548));
#60520=CARTESIAN_POINT('',(424.438982237057,326.016308993799,386.862702781548));
#60521=CARTESIAN_POINT('Ctrl Pts',(424.438982237031,326.016308993792,386.862702781548));
#60522=CARTESIAN_POINT('Ctrl Pts',(425.720192393527,326.386162508165,386.862702781548));
#60523=CARTESIAN_POINT('Ctrl Pts',(426.841736190502,326.480565703216,386.862702781548));
#60524=CARTESIAN_POINT('Ctrl Pts',(423.237605260334,326.480565703216,388.943548744275));
#60525=CARTESIAN_POINT('Ctrl Pts',(423.798377158822,326.386162508165,387.972263324638));
#60526=CARTESIAN_POINT('Ctrl Pts',(424.438982237069,326.016308993792,386.862702781526));
#60527=CARTESIAN_POINT('Origin',(430.909330445546,323.655272903216,398.038702781548));
#60528=CARTESIAN_POINT('',(430.89144884552,326.0163089938,398.038702781548));
#60529=CARTESIAN_POINT('Ctrl Pts',(430.891448845546,326.016308993792,398.038702781548));
#60530=CARTESIAN_POINT('Ctrl Pts',(429.61023868905,326.386162508165,398.038702781548));
#60531=CARTESIAN_POINT('Ctrl Pts',(428.488694892075,326.480565703216,398.038702781548));
#60532=CARTESIAN_POINT('',(424.438982237057,326.016308993799,398.038702781548));
#60533=CARTESIAN_POINT('Ctrl Pts',(426.841736190502,326.480565703216,398.038702781548));
#60534=CARTESIAN_POINT('Ctrl Pts',(425.720192393527,326.386162508165,398.038702781548));
#60535=CARTESIAN_POINT('Ctrl Pts',(424.438982237031,326.016308993792,398.038702781548));
#60536=CARTESIAN_POINT('',(424.438982237057,326.016308993799,398.038702781548));
#60537=CARTESIAN_POINT('',(430.89144884552,326.016308993799,398.038702781548));
#60538=CARTESIAN_POINT('Origin',(432.504565497636,326.498447303216,395.244702781548));
#60539=CARTESIAN_POINT('',(434.117682149752,326.0163089938,392.450702781548));
#60540=CARTESIAN_POINT('Ctrl Pts',(434.117682149764,326.016308993792,392.450702781526));
#60541=CARTESIAN_POINT('Ctrl Pts',(433.477077071517,326.386162508165,393.560263324638));
#60542=CARTESIAN_POINT('Ctrl Pts',(432.916305173029,326.480565703216,394.531548744275));
#60543=CARTESIAN_POINT('Ctrl Pts',(432.092825822242,326.480565703216,395.957856818821));
#60544=CARTESIAN_POINT('Ctrl Pts',(431.532053923755,326.386162508165,396.929142238459));
#60545=CARTESIAN_POINT('Ctrl Pts',(430.891448845507,326.016308993792,398.03870278157));
#60546=CARTESIAN_POINT('',(434.117682149752,326.016308993799,392.450702781548));
#60547=CARTESIAN_POINT('Origin',(427.665215541288,326.062734664734,392.450702781549));
#60548=CARTESIAN_POINT('',(430.89144884552,326.0163089938,386.862702781548));
#60549=CARTESIAN_POINT('Ctrl Pts',(428.488694892075,326.480565703216,386.862702781548));
#60550=CARTESIAN_POINT('Ctrl Pts',(429.61023868905,326.386162508165,386.862702781548));
#60551=CARTESIAN_POINT('Ctrl Pts',(430.891448845545,326.016308993792,386.862702781548));
#60552=CARTESIAN_POINT('Ctrl Pts',(430.891448845507,326.016308993792,386.862702781526));
#60553=CARTESIAN_POINT('Ctrl Pts',(431.532053923755,326.386162508165,387.972263324638));
#60554=CARTESIAN_POINT('Ctrl Pts',(432.092825822242,326.480565703216,388.943548744275));
#60555=CARTESIAN_POINT('Origin',(427.665215541293,326.062734664737,392.450702781548));
#60556=CARTESIAN_POINT('Ctrl Pts',(432.916305173029,326.480565703216,390.369856818821));
#60557=CARTESIAN_POINT('Ctrl Pts',(433.477077071517,326.386162508165,391.341142238458));
#60558=CARTESIAN_POINT('Ctrl Pts',(434.117682149764,326.016308993792,392.45070278157));
#60559=CARTESIAN_POINT('Origin',(427.665215541288,326.062734664734,392.450702781548));
#60560=CARTESIAN_POINT('Origin',(427.665215541289,326.062734664734,392.450702781548));
#60561=CARTESIAN_POINT('',(421.212748932825,326.016308993799,392.450702781548));
#60562=CARTESIAN_POINT('Ctrl Pts',(422.414125909548,326.480565703216,394.531548744275));
#60563=CARTESIAN_POINT('Ctrl Pts',(421.85335401106,326.386162508165,393.560263324638));
#60564=CARTESIAN_POINT('Ctrl Pts',(421.212748932812,326.016308993791,392.450702781526));
#60565=CARTESIAN_POINT('Ctrl Pts',(421.212748932812,326.016308993791,392.45070278157));
#60566=CARTESIAN_POINT('Ctrl Pts',(421.85335401106,326.386162508165,391.341142238459));
#60567=CARTESIAN_POINT('Ctrl Pts',(422.414125909547,326.480565703216,390.369856818821));
#60568=CARTESIAN_POINT('Origin',(427.665215541289,326.062734664734,392.450702781548));
#60569=CARTESIAN_POINT('Ctrl Pts',(424.438982237069,326.016308993792,398.03870278157));
#60570=CARTESIAN_POINT('Ctrl Pts',(423.798377158822,326.386162508165,396.929142238459));
#60571=CARTESIAN_POINT('Ctrl Pts',(423.237605260334,326.480565703216,395.957856818821));
#60572=CARTESIAN_POINT('Origin',(422.825865584941,326.498447303216,395.244702781548));
#60573=CARTESIAN_POINT('',(421.212748932825,326.016308993798,392.450702781548));
#60574=CARTESIAN_POINT('Origin',(422.825865584941,326.498447303216,389.656702781548));
#60575=CARTESIAN_POINT('',(424.438982237057,326.016308993799,386.862702781548));
#60576=CARTESIAN_POINT('Origin',(430.909330445546,323.655272903216,386.862702781548));
#60577=CARTESIAN_POINT('',(430.89144884552,326.016308993799,386.862702781548));
#60578=CARTESIAN_POINT('Origin',(432.504565497636,326.498447303216,389.656702781548));
#60579=CARTESIAN_POINT('Origin',(280.876756490954,220.460559303207,538.878400551892));
#60580=CARTESIAN_POINT('',(277.226674890954,216.828359303207,538.878400551892));
#60581=CARTESIAN_POINT('Origin',(277.226674890954,220.460559303207,538.878400551892));
#60582=CARTESIAN_POINT('Origin',(323.345556490953,220.46055930321,538.878400551891));
#60583=CARTESIAN_POINT('',(319.695474890954,216.82835930321,538.878400551891));
#60584=CARTESIAN_POINT('Origin',(319.695474890954,220.46055930321,538.878400551891));
#60585=CARTESIAN_POINT('Origin',(280.87675649095,274.105359303207,538.878400551891));
#60586=CARTESIAN_POINT('',(277.22667489095,270.473159303207,538.878400551891));
#60587=CARTESIAN_POINT('Origin',(277.22667489095,274.105359303207,538.878400551891));
#60588=CARTESIAN_POINT('Origin',(298.461074890955,194.755759303208,556.760000551892));
#60589=CARTESIAN_POINT('',(298.461074890955,197.503267143208,560.336320551892));
#60590=CARTESIAN_POINT('Origin',(298.461074890955,194.755759303208,560.336320551892));
#60591=CARTESIAN_POINT('',(298.461074890955,197.503267143208,553.183680551892));
#60592=CARTESIAN_POINT('',(298.461074890955,197.503267143208,556.760000551892));
#60593=CARTESIAN_POINT('Origin',(298.461074890955,194.755759303208,553.183680551892));
#60594=CARTESIAN_POINT('Origin',(298.461074890948,299.810159303208,556.760000551891));
#60595=CARTESIAN_POINT('',(298.461074890948,302.557667143208,560.336320551891));
#60596=CARTESIAN_POINT('Origin',(298.461074890948,299.810159303208,560.336320551891));
#60597=CARTESIAN_POINT('',(298.461074890948,302.557667143208,553.183680551891));
#60598=CARTESIAN_POINT('',(298.461074890948,302.557667143208,556.760000551891));
#60599=CARTESIAN_POINT('Origin',(298.461074890948,299.810159303208,553.183680551891));
#60600=CARTESIAN_POINT('Origin',(298.461074890952,247.282959303208,538.699584551891));
#60601=CARTESIAN_POINT('',(298.46107489095,269.108793223208,543.348800551891));
#60602=CARTESIAN_POINT('Origin',(298.461074890952,247.282959303208,543.348800551891));
#60603=CARTESIAN_POINT('',(298.46107489095,269.108793223208,538.699584551891));
#60604=CARTESIAN_POINT('Origin',(335.603414207691,284.425298619953,556.760000551891));
#60605=CARTESIAN_POINT('',(335.603414207691,288.057498619953,560.336320551891));
#60606=CARTESIAN_POINT('Origin',(335.603414207691,284.425298619953,560.336320551891));
#60607=CARTESIAN_POINT('',(335.603414207691,288.057498619953,553.183680551891));
#60608=CARTESIAN_POINT('',(335.603414207691,288.057498619953,556.760000551891));
#60609=CARTESIAN_POINT('Origin',(335.603414207691,284.425298619953,553.183680551891));
#60610=CARTESIAN_POINT('Origin',(335.603414207696,210.140619986469,556.760000551891));
#60611=CARTESIAN_POINT('',(335.603414207696,213.772819986469,560.336320551891));
#60612=CARTESIAN_POINT('Origin',(335.603414207696,210.140619986469,560.336320551892));
#60613=CARTESIAN_POINT('',(335.603414207696,213.772819986469,553.183680551891));
#60614=CARTESIAN_POINT('',(335.603414207696,213.772819986469,556.760000551891));
#60615=CARTESIAN_POINT('Origin',(335.603414207696,210.140619986469,553.183680551891));
#60616=CARTESIAN_POINT('Origin',(261.318735574212,210.140619986464,556.760000551892));
#60617=CARTESIAN_POINT('',(261.318735574212,213.772819986464,560.336320551892));
#60618=CARTESIAN_POINT('Origin',(261.318735574212,210.140619986464,560.336320551892));
#60619=CARTESIAN_POINT('',(261.318735574212,213.772819986464,553.183680551891));
#60620=CARTESIAN_POINT('',(261.318735574212,213.772819986464,556.760000551892));
#60621=CARTESIAN_POINT('Origin',(261.318735574212,210.140619986464,553.183680551892));
#60622=CARTESIAN_POINT('Origin',(261.318735574207,284.425298619948,556.760000551891));
#60623=CARTESIAN_POINT('',(261.318735574207,288.057498619948,560.336320551891));
#60624=CARTESIAN_POINT('Origin',(261.318735574207,284.425298619948,560.336320551891));
#60625=CARTESIAN_POINT('',(261.318735574207,288.057498619948,553.183680551891));
#60626=CARTESIAN_POINT('',(261.318735574207,288.057498619948,556.760000551891));
#60627=CARTESIAN_POINT('Origin',(261.318735574207,284.425298619948,553.183680551891));
#60628=CARTESIAN_POINT('Origin',(331.524498889391,292.950375595403,555.865920551891));
#60629=CARTESIAN_POINT('',(323.713038793177,284.604387432155,555.865920551891));
#60630=CARTESIAN_POINT('',(305.715314890949,291.756846928711,555.865920551891));
#60631=CARTESIAN_POINT('Origin',(298.461074890952,247.282959303207,555.865920551892));
#60632=CARTESIAN_POINT('',(326.432817338928,284.864294221222,555.865920551891));
#60633=CARTESIAN_POINT('Origin',(324.915513264712,286.381598295438,555.865920551891));
#60634=CARTESIAN_POINT('',(330.801832688819,289.233309571114,555.865920551891));
#60635=CARTESIAN_POINT('',(326.432817338928,284.864294221222,555.865920551891));
#60636=CARTESIAN_POINT('',(330.525741198797,292.500989213059,555.865920551891));
#60637=CARTESIAN_POINT('Origin',(329.284528614603,290.75061364533,555.865920551891));
#60638=CARTESIAN_POINT('',(306.366782273498,302.149277250954,555.865920551891));
#60639=CARTESIAN_POINT('Origin',(298.461074890953,247.282959303211,555.865920551892));
#60640=CARTESIAN_POINT('',(303.914962890948,300.025419782009,555.865920551891));
#60641=CARTESIAN_POINT('Origin',(306.060754890948,300.025419782009,555.865920551891));
#60642=CARTESIAN_POINT('',(303.914962890949,293.874651101354,555.865920551891));
#60643=CARTESIAN_POINT('',(303.914962890948,300.025419782009,555.865920551891));
#60644=CARTESIAN_POINT('Origin',(306.060754890949,293.874651101354,555.865920551891));
#60645=CARTESIAN_POINT('Origin',(351.010702786122,254.077967303212,558.101120551891));
#60646=CARTESIAN_POINT('',(344.814100392115,254.077967303212,560.336320551891));
#60647=CARTESIAN_POINT('',(350.992821186122,254.077967303212,560.336320551891));
#60648=CARTESIAN_POINT('',(344.814100392115,254.077967303212,560.336320551891));
#60649=CARTESIAN_POINT('',(350.992821186122,254.077967303212,555.865920551891));
#60650=CARTESIAN_POINT('',(350.992821186122,254.077967303212,555.865920551891));
#60651=CARTESIAN_POINT('',(344.814100392115,254.077967303212,555.865920551891));
#60652=CARTESIAN_POINT('',(344.814100392115,254.077967303212,555.865920551891));
#60653=CARTESIAN_POINT('',(344.814100392115,254.077967303212,555.865920551891));
#60654=CARTESIAN_POINT('Origin',(350.992821186122,256.223759303212,558.101120551891));
#60655=CARTESIAN_POINT('',(353.108193550251,256.583791341156,560.336320551891));
#60656=CARTESIAN_POINT('Origin',(350.992821186122,256.223759303212,560.336320551891));
#60657=CARTESIAN_POINT('',(353.108193550251,256.583791341156,555.865920551891));
#60658=CARTESIAN_POINT('',(353.108193550251,256.583791341156,555.865920551891));
#60659=CARTESIAN_POINT('Origin',(350.992821186122,256.223759303212,555.865920551891));
#60660=CARTESIAN_POINT('Origin',(298.461074890952,247.282959303209,558.101120551891));
#60661=CARTESIAN_POINT('',(343.679104575705,279.347625928489,560.336320551891));
#60662=CARTESIAN_POINT('Origin',(298.461074890952,247.282959303209,560.336320551891));
#60663=CARTESIAN_POINT('',(343.679104575705,279.347625928489,555.865920551891));
#60664=CARTESIAN_POINT('',(343.679104575705,279.347625928489,555.865920551891));
#60665=CARTESIAN_POINT('Origin',(298.461074890952,247.282959303209,555.865920551891));
#60666=CARTESIAN_POINT('Origin',(341.928729233069,278.106413026865,558.101120551891));
#60667=CARTESIAN_POINT('',(340.411425158853,279.623717101081,560.336320551891));
#60668=CARTESIAN_POINT('Origin',(341.928729233069,278.106413026865,560.336320551891));
#60669=CARTESIAN_POINT('',(340.411425158853,279.623717101081,555.865920551891));
#60670=CARTESIAN_POINT('',(340.411425158853,279.623717101081,555.865920551891));
#60671=CARTESIAN_POINT('Origin',(341.928729233069,278.106413026866,555.865920551891));
#60672=CARTESIAN_POINT('Origin',(338.226917483907,277.439209426135,555.848038951891));
#60673=CARTESIAN_POINT('',(336.042409808962,275.254701751189,560.336320551891));
#60674=CARTESIAN_POINT('',(340.411425158853,279.623717101081,560.336320551891));
#60675=CARTESIAN_POINT('',(336.042409808962,275.254701751189,555.865920551891));
#60676=CARTESIAN_POINT('',(336.042409808962,275.254701751189,555.865920551891));
#60677=CARTESIAN_POINT('',(340.411425158853,279.623717101081,555.865920551891));
#60678=CARTESIAN_POINT('Origin',(337.559713883178,273.737397676974,558.101120551891));
#60679=CARTESIAN_POINT('',(335.782502581966,272.53492385268,560.336320551891));
#60680=CARTESIAN_POINT('Origin',(337.559713883178,273.737397676974,560.336320551891));
#60681=CARTESIAN_POINT('',(335.782502581966,272.53492385268,555.865920551891));
#60682=CARTESIAN_POINT('',(335.782502581966,272.53492385268,555.865920551891));
#60683=CARTESIAN_POINT('Origin',(337.559713883178,273.737397676974,555.865920551891));
#60684=CARTESIAN_POINT('Origin',(298.461074890951,247.282959303208,558.101120551891));
#60685=CARTESIAN_POINT('',(342.707144718038,255.817359303211,560.336320551891));
#60686=CARTESIAN_POINT('Origin',(298.461074890951,247.282959303208,560.336320551891));
#60687=CARTESIAN_POINT('',(342.707144718038,255.817359303211,555.865920551891));
#60688=CARTESIAN_POINT('',(342.707144718038,255.817359303211,555.865920551891));
#60689=CARTESIAN_POINT('Origin',(298.461074890951,247.282959303208,555.865920551891));
#60690=CARTESIAN_POINT('Origin',(344.814100424089,256.223759303212,558.101120551891));
#60691=CARTESIAN_POINT('Origin',(344.814100424089,256.223759303212,560.336320551891));
#60692=CARTESIAN_POINT('Origin',(344.814100424089,256.223759303212,555.865920551891));
#60693=CARTESIAN_POINT('Origin',(353.29330925736,267.203234460617,555.865920551891));
#60694=CARTESIAN_POINT('Origin',(338.226917483912,217.126709180287,555.848038951891));
#60695=CARTESIAN_POINT('',(336.042409808966,219.311216855232,560.336320551891));
#60696=CARTESIAN_POINT('',(340.411425158857,214.942201505341,560.336320551891));
#60697=CARTESIAN_POINT('',(336.042409808966,219.311216855232,560.336320551891));
#60698=CARTESIAN_POINT('',(340.411425158857,214.942201505341,555.865920551891));
#60699=CARTESIAN_POINT('',(340.411425158857,214.942201505341,555.865920551891));
#60700=CARTESIAN_POINT('',(336.042409808966,219.311216855232,555.865920551891));
#60701=CARTESIAN_POINT('',(336.042409808966,219.311216855232,555.865920551891));
#60702=CARTESIAN_POINT('',(336.042409808966,219.311216855232,555.865920551891));
#60703=CARTESIAN_POINT('Origin',(341.928729233073,216.459505579557,558.101120551891));
#60704=CARTESIAN_POINT('',(343.679104471958,215.218292531622,560.336320551891));
#60705=CARTESIAN_POINT('Origin',(341.928729233073,216.459505579557,560.336320551891));
#60706=CARTESIAN_POINT('',(343.679104471958,215.218292531622,555.865920551891));
#60707=CARTESIAN_POINT('',(343.679104471958,215.218292531622,555.865920551891));
#60708=CARTESIAN_POINT('Origin',(341.928729233073,216.459505579557,555.865920551891));
#60709=CARTESIAN_POINT('Origin',(298.461074890951,247.282959303208,558.101120551891));
#60710=CARTESIAN_POINT('',(353.108193520157,237.982127088447,560.336320551891));
#60711=CARTESIAN_POINT('Origin',(298.461074890952,247.282959303209,560.336320551891));
#60712=CARTESIAN_POINT('',(353.108193520157,237.982127088447,555.865920551891));
#60713=CARTESIAN_POINT('',(353.108193520157,237.982127088447,555.865920551891));
#60714=CARTESIAN_POINT('Origin',(298.461074890952,247.282959303208,555.865920551892));
#60715=CARTESIAN_POINT('Origin',(350.992821186124,238.342159303212,558.101120551891));
#60716=CARTESIAN_POINT('',(350.992821154148,240.487951303212,560.336320551891));
#60717=CARTESIAN_POINT('Origin',(350.992821186123,238.342159303212,560.336320551891));
#60718=CARTESIAN_POINT('',(350.992821154148,240.487951303212,555.865920551891));
#60719=CARTESIAN_POINT('',(350.992821154148,240.487951303212,555.865920551891));
#60720=CARTESIAN_POINT('Origin',(350.992821186123,238.342159303212,555.865920551891));
#60721=CARTESIAN_POINT('Origin',(351.010702754149,240.487951303212,558.101120551891));
#60722=CARTESIAN_POINT('',(344.81410042409,240.487951303211,560.336320551891));
#60723=CARTESIAN_POINT('',(350.992821154148,240.487951303212,560.336320551891));
#60724=CARTESIAN_POINT('',(344.81410042409,240.487951303211,555.865920551891));
#60725=CARTESIAN_POINT('',(344.81410042409,240.487951303211,555.865920551891));
#60726=CARTESIAN_POINT('',(350.992821154148,240.487951303212,555.865920551891));
#60727=CARTESIAN_POINT('Origin',(344.81410042409,238.342159303212,558.101120551891));
#60728=CARTESIAN_POINT('',(342.707144808688,238.748559773175,560.336320551891));
#60729=CARTESIAN_POINT('Origin',(344.81410042409,238.342159303211,560.336320551891));
#60730=CARTESIAN_POINT('',(342.707144808688,238.748559773175,555.865920551891));
#60731=CARTESIAN_POINT('',(342.707144808688,238.748559773175,555.865920551891));
#60732=CARTESIAN_POINT('Origin',(344.81410042409,238.342159303211,555.865920551891));
#60733=CARTESIAN_POINT('Origin',(298.461074890952,247.282959303208,558.101120551891));
#60734=CARTESIAN_POINT('',(335.782502502643,222.030994636499,560.336320551891));
#60735=CARTESIAN_POINT('Origin',(298.461074890951,247.282959303209,560.33632055189));
#60736=CARTESIAN_POINT('',(335.782502502643,222.030994636499,555.865920551891));
#60737=CARTESIAN_POINT('',(335.782502502643,222.030994636499,555.865920551891));
#60738=CARTESIAN_POINT('Origin',(298.461074890951,247.282959303209,555.865920551889));
#60739=CARTESIAN_POINT('Origin',(337.559713883181,220.828520929449,558.101120551891));
#60740=CARTESIAN_POINT('Origin',(337.559713883181,220.828520929448,560.336320551891));
#60741=CARTESIAN_POINT('Origin',(337.559713883181,220.828520929448,555.865920551891));
#60742=CARTESIAN_POINT('Origin',(353.293309320179,227.362684172507,555.865920551891));
#60743=CARTESIAN_POINT('Origin',(303.914962890955,197.615883164736,555.848038951892));
#60744=CARTESIAN_POINT('',(303.914962890955,200.691267505063,560.336320551892));
#60745=CARTESIAN_POINT('',(303.914962890955,194.540498824408,560.336320551892));
#60746=CARTESIAN_POINT('',(303.914962890955,200.691267505063,560.336320551892));
#60747=CARTESIAN_POINT('',(303.914962890955,194.540498824408,555.865920551892));
#60748=CARTESIAN_POINT('',(303.914962890955,194.540498824408,555.865920551892));
#60749=CARTESIAN_POINT('',(303.914962890955,200.691267505063,555.865920551892));
#60750=CARTESIAN_POINT('',(303.914962890955,200.691267505063,555.865920551892));
#60751=CARTESIAN_POINT('',(303.914962890955,200.691267505063,555.865920551892));
#60752=CARTESIAN_POINT('Origin',(306.060754890955,194.540498824408,558.101120551892));
#60753=CARTESIAN_POINT('',(306.366782273506,192.416641355463,560.336320551892));
#60754=CARTESIAN_POINT('Origin',(306.060754890955,194.540498824409,560.336320551892));
#60755=CARTESIAN_POINT('',(306.366782273505,192.416641355463,555.865920551892));
#60756=CARTESIAN_POINT('',(306.366782273505,192.416641355463,555.865920551892));
#60757=CARTESIAN_POINT('Origin',(306.060754890955,194.540498824409,555.865920551892));
#60758=CARTESIAN_POINT('Origin',(298.461074890951,247.282959303211,558.101120551891));
#60759=CARTESIAN_POINT('',(330.525741516232,202.064929618455,560.336320551892));
#60760=CARTESIAN_POINT('Origin',(298.461074890951,247.282959303209,560.336320551892));
#60761=CARTESIAN_POINT('',(330.525741516232,202.064929618455,555.865920551891));
#60762=CARTESIAN_POINT('',(330.525741516232,202.064929618455,555.865920551891));
#60763=CARTESIAN_POINT('Origin',(298.461074890951,247.282959303209,555.86592055189));
#60764=CARTESIAN_POINT('Origin',(329.284528614608,203.815304961091,558.101120551892));
#60765=CARTESIAN_POINT('',(330.801832688824,205.332609035307,560.336320551892));
#60766=CARTESIAN_POINT('Origin',(329.284528614609,203.815304961091,560.336320551892));
#60767=CARTESIAN_POINT('',(330.801832688824,205.332609035307,555.865920551891));
#60768=CARTESIAN_POINT('',(330.801832688824,205.332609035307,555.865920551891));
#60769=CARTESIAN_POINT('Origin',(329.284528614609,203.815304961091,555.865920551891));
#60770=CARTESIAN_POINT('Origin',(328.617325013878,207.517116710252,555.848038951891));
#60771=CARTESIAN_POINT('',(326.432817338932,209.701624385198,560.336320551892));
#60772=CARTESIAN_POINT('',(330.801832688824,205.332609035307,560.336320551892));
#60773=CARTESIAN_POINT('',(326.432817338932,209.701624385198,555.865920551891));
#60774=CARTESIAN_POINT('',(326.432817338932,209.701624385198,555.865920551891));
#60775=CARTESIAN_POINT('',(330.801832688824,205.332609035307,555.865920551891));
#60776=CARTESIAN_POINT('Origin',(324.915513264717,208.184320310982,558.101120551891));
#60777=CARTESIAN_POINT('',(323.713039257659,209.961531488534,560.336320551892));
#60778=CARTESIAN_POINT('Origin',(324.915513264717,208.184320310982,560.336320551892));
#60779=CARTESIAN_POINT('',(323.713039257659,209.961531488534,555.865920551891));
#60780=CARTESIAN_POINT('',(323.713039257659,209.961531488534,555.865920551891));
#60781=CARTESIAN_POINT('Origin',(324.915513264717,208.184320310982,555.865920551891));
#60782=CARTESIAN_POINT('Origin',(298.461074890953,247.282959303205,558.101120551891));
#60783=CARTESIAN_POINT('',(305.715314890955,202.809071677706,560.336320551892));
#60784=CARTESIAN_POINT('Origin',(298.461074890953,247.282959303206,560.336320551891));
#60785=CARTESIAN_POINT('',(305.715314890955,202.809071677706,555.865920551892));
#60786=CARTESIAN_POINT('',(305.715314890955,202.809071677706,555.865920551892));
#60787=CARTESIAN_POINT('Origin',(298.461074890953,247.282959303206,555.865920551891));
#60788=CARTESIAN_POINT('Origin',(306.060754890955,200.691267505063,558.101120551892));
#60789=CARTESIAN_POINT('Origin',(306.060754890955,200.691267505063,560.336320551892));
#60790=CARTESIAN_POINT('Origin',(306.060754890955,200.691267505063,555.865920551892));
#60791=CARTESIAN_POINT('Origin',(331.524498805765,201.615542844315,555.865920551891));
#60792=CARTESIAN_POINT('Origin',(277.22667489095,274.105359303207,543.795840551891));
#60793=CARTESIAN_POINT('',(277.22667489095,270.473159303207,548.713280551891));
#60794=CARTESIAN_POINT('',(277.22667489095,270.473159303207,543.795840551891));
#60795=CARTESIAN_POINT('Origin',(277.22667489095,274.105359303207,548.713280551891));
#60796=CARTESIAN_POINT('Origin',(319.695474890954,220.46055930321,543.795840551891));
#60797=CARTESIAN_POINT('',(319.695474890954,216.82835930321,548.713280551891));
#60798=CARTESIAN_POINT('',(319.695474890954,216.82835930321,543.795840551891));
#60799=CARTESIAN_POINT('Origin',(319.695474890954,220.46055930321,548.713280551891));
#60800=CARTESIAN_POINT('Origin',(277.226674890954,220.460559303207,543.795840551892));
#60801=CARTESIAN_POINT('',(277.226674890954,216.828359303207,548.713280551892));
#60802=CARTESIAN_POINT('',(277.226674890954,216.828359303207,543.795840551892));
#60803=CARTESIAN_POINT('Origin',(277.226674890954,220.460559303207,548.713280551892));
#60804=CARTESIAN_POINT('Origin',(298.461074890952,247.282959303208,558.655450151891));
#60805=CARTESIAN_POINT('',(327.384562890954,219.289859923024,560.336320551891));
#60806=CARTESIAN_POINT('',(327.38456289095,275.276058683397,560.336320551891));
#60807=CARTESIAN_POINT('Origin',(298.461074890952,247.282959303208,560.336320551891));
#60808=CARTESIAN_POINT('',(327.267168315382,275.396848266106,556.974579751891));
#60809=CARTESIAN_POINT('Origin',(308.672610372403,257.207479808827,24.496731278983));
#60810=CARTESIAN_POINT('',(327.267168315386,219.169070340315,556.974579751891));
#60811=CARTESIAN_POINT('Origin',(298.461074890952,247.282959303208,556.974579751891));
#60812=CARTESIAN_POINT('Origin',(308.657304290093,237.373317660302,24.0584227317262));
#60813=CARTESIAN_POINT('Origin',(354.723367946653,247.282959303212,556.974579751891));
#60814=CARTESIAN_POINT('',(327.267168315382,275.396848266106,556.974579751891));
#60815=CARTESIAN_POINT('Origin',(298.461074890952,247.282959303209,558.655450151891));
#60816=CARTESIAN_POINT('',(311.739002757719,285.281359303209,560.336320551891));
#60817=CARTESIAN_POINT('',(285.183147024179,285.281359303207,560.336320551891));
#60818=CARTESIAN_POINT('Origin',(298.461074890952,247.282959303206,560.336320551891));
#60819=CARTESIAN_POINT('',(284.851842766054,285.16396472764,556.974579751891));
#60820=CARTESIAN_POINT('Origin',(1528.18940949044,280.947624093096,436.288406677437));
#60821=CARTESIAN_POINT('',(312.070307015844,285.163964727641,556.974579751891));
#60822=CARTESIAN_POINT('Origin',(298.461074890952,247.282959303209,556.974579751891));
#60823=CARTESIAN_POINT('Origin',(-931.267259897731,280.947624001165,436.288406661732));
#60824=CARTESIAN_POINT('Origin',(312.088188615844,287.608609437492,556.974579751891));
#60825=CARTESIAN_POINT('',(284.851842766054,285.16396472764,556.974579751891));
#60826=CARTESIAN_POINT('Origin',(298.461074890952,247.282959303209,558.655450151891));
#60827=CARTESIAN_POINT('',(269.53758689095,275.276058683393,560.336320551891));
#60828=CARTESIAN_POINT('',(269.654981466518,275.396848266102,556.974579751891));
#60829=CARTESIAN_POINT('Origin',(288.253780195306,257.203359931411,24.3752918824331));
#60830=CARTESIAN_POINT('',(269.537586890954,219.28985992302,560.336320551892));
#60831=CARTESIAN_POINT('Origin',(298.461074890952,247.282959303208,560.336320551891));
#60832=CARTESIAN_POINT('',(269.654981466522,219.169070340311,556.974579751891));
#60833=CARTESIAN_POINT('Origin',(288.259429378608,237.368050819944,24.2135203256732));
#60834=CARTESIAN_POINT('Origin',(298.461074890951,247.282959303208,556.974579751891));
#60835=CARTESIAN_POINT('Origin',(269.67286306652,247.282959303206,556.974579751891));
#60836=CARTESIAN_POINT('',(269.654981466522,219.169070340311,556.974579751891));
#60837=CARTESIAN_POINT('Origin',(288.644076490954,218.651822053524,548.713280551891));
#60838=CARTESIAN_POINT('',(288.626194890954,209.690444803841,548.713280551892));
#60839=CARTESIAN_POINT('',(278.478386890954,209.69044480384,548.713280551892));
#60840=CARTESIAN_POINT('',(288.626194890954,209.690444803841,548.713280551892));
#60841=CARTESIAN_POINT('',(288.626194890954,218.672399303208,548.713280551891));
#60842=CARTESIAN_POINT('',(288.626194890954,218.672399303208,548.713280551891));
#60843=CARTESIAN_POINT('',(279.685394890953,227.613199303207,548.713280551891));
#60844=CARTESIAN_POINT('Origin',(279.685394890954,218.672399303207,548.713280551892));
#60845=CARTESIAN_POINT('',(269.943472391586,227.613199303206,548.713280551891));
#60846=CARTESIAN_POINT('',(269.943472391586,227.613199303206,548.713280551891));
#60847=CARTESIAN_POINT('',(269.943472391587,218.225359303206,548.713280551892));
#60848=CARTESIAN_POINT('',(269.943472391587,218.225359303206,548.713280551892));
#60849=CARTESIAN_POINT('Origin',(278.478386890954,218.225359303207,548.713280551892));
#60850=CARTESIAN_POINT('Origin',(288.64407649095,275.914096552891,548.713280551891));
#60851=CARTESIAN_POINT('',(278.478386890949,284.875473802573,548.713280551891));
#60852=CARTESIAN_POINT('',(288.626194890949,284.875473802574,548.713280551891));
#60853=CARTESIAN_POINT('',(278.478386890949,284.875473802574,548.713280551891));
#60854=CARTESIAN_POINT('',(269.943472391583,276.340559303206,548.713280551891));
#60855=CARTESIAN_POINT('Origin',(278.47838689095,276.340559303207,548.713280551891));
#60856=CARTESIAN_POINT('',(269.943472391583,266.952719303206,548.713280551891));
#60857=CARTESIAN_POINT('',(269.943472391583,266.952719303206,548.713280551891));
#60858=CARTESIAN_POINT('',(279.68539489095,266.952719303207,548.713280551891));
#60859=CARTESIAN_POINT('',(279.68539489095,266.952719303207,548.713280551891));
#60860=CARTESIAN_POINT('',(288.62619489095,275.893519303208,548.713280551891));
#60861=CARTESIAN_POINT('Origin',(279.68539489095,275.893519303207,548.713280551891));
#60862=CARTESIAN_POINT('',(288.626194890949,284.875473802574,548.713280551891));
#60863=CARTESIAN_POINT('Origin',(326.996558990316,275.914096552894,548.713280551891));
#60864=CARTESIAN_POINT('',(326.978677390316,276.34055930321,548.713280551891));
#60865=CARTESIAN_POINT('',(326.978677390317,266.95271930321,548.713280551891));
#60866=CARTESIAN_POINT('',(326.978677390316,276.34055930321,548.713280551891));
#60867=CARTESIAN_POINT('',(318.443762890949,284.875473802576,548.713280551891));
#60868=CARTESIAN_POINT('Origin',(318.44376289095,276.34055930321,548.713280551891));
#60869=CARTESIAN_POINT('',(308.295954890949,284.875473802576,548.713280551891));
#60870=CARTESIAN_POINT('',(308.295954890949,284.875473802576,548.713280551891));
#60871=CARTESIAN_POINT('',(308.29595489095,275.893519303209,548.713280551891));
#60872=CARTESIAN_POINT('',(308.29595489095,275.893519303209,548.713280551891));
#60873=CARTESIAN_POINT('',(317.23675489095,266.95271930321,548.713280551891));
#60874=CARTESIAN_POINT('Origin',(317.23675489095,275.89351930321,548.713280551891));
#60875=CARTESIAN_POINT('',(326.978677390317,266.95271930321,548.713280551891));
#60876=CARTESIAN_POINT('',(322.550443684267,270.107056728403,548.713280551891));
#60877=CARTESIAN_POINT('Origin',(319.69547489095,274.10535930321,548.713280551891));
#60878=CARTESIAN_POINT('Origin',(298.461074890956,247.282959303207,559.796751782383));
#60879=CARTESIAN_POINT('',(264.689833477746,294.578622153519,560.336320551894));
#60880=CARTESIAN_POINT('Origin',(298.461074890952,247.282959303208,560.336320551891));
#60881=CARTESIAN_POINT('',(264.74456349207,294.501974325459,554.940632856795));
#60882=CARTESIAN_POINT('',(264.695306479179,294.570957370713,559.796751782384));
#60883=CARTESIAN_POINT('',(298.461074890956,189.261941382259,554.940632856797));
#60884=CARTESIAN_POINT('Origin',(298.461074890952,247.282959303208,554.940632856796));
#60885=CARTESIAN_POINT('Origin',(298.461074890952,247.282959303208,554.940632856796));
#60886=CARTESIAN_POINT('Origin',(280.594960810809,284.397922553604,536.282915140689));
#60887=CARTESIAN_POINT('',(276.061696911308,288.167387864213,542.153831267514));
#60888=CARTESIAN_POINT('',(276.061696911308,288.167387864213,542.153831267514));
#60889=CARTESIAN_POINT('',(267.053894329943,279.159585282847,542.153831267514));
#60890=CARTESIAN_POINT('',(267.16827489095,274.641807303206,538.878400551891));
#60891=CARTESIAN_POINT('',(267.053894329943,279.159585282847,542.153831267514));
#60892=CARTESIAN_POINT('Origin',(329.883741371816,279.879071753365,542.673535228732));
#60893=CARTESIAN_POINT('',(320.860452870589,288.167387864216,542.153831267514));
#60894=CARTESIAN_POINT('',(316.342674890949,288.053007303209,538.878400551891));
#60895=CARTESIAN_POINT('',(329.868255451956,279.159585282851,542.153831267514));
#60896=CARTESIAN_POINT('',(320.860452870589,288.167387864216,542.153831267514));
#60897=CARTESIAN_POINT('',(329.868255451956,279.159585282851,542.153831267514));
#60898=CARTESIAN_POINT('Origin',(280.594960810814,210.16799605281,536.28291514069));
#60899=CARTESIAN_POINT('',(267.053894329947,215.406333323565,542.153831267515));
#60900=CARTESIAN_POINT('',(267.053894329947,215.406333323565,542.153831267515));
#60901=CARTESIAN_POINT('',(276.061696911314,206.3985307422,542.153831267515));
#60902=CARTESIAN_POINT('',(280.579474890954,206.512911303207,538.878400551892));
#60903=CARTESIAN_POINT('',(276.061696911314,206.3985307422,542.153831267515));
#60904=CARTESIAN_POINT('Origin',(329.883741371821,214.686846853056,542.673535228733));
#60905=CARTESIAN_POINT('',(320.860452870594,206.398530742203,542.153831267515));
#60906=CARTESIAN_POINT('',(320.860452870594,206.398530742203,542.153831267515));
#60907=CARTESIAN_POINT('',(329.86825545196,215.40633332357,542.153831267514));
#60908=CARTESIAN_POINT('',(329.753874890953,219.92411130321,538.878400551891));
#60909=CARTESIAN_POINT('',(329.86825545196,215.40633332357,542.153831267514));
#60910=CARTESIAN_POINT('Origin',(269.834195526028,276.358440903206,551.842560551891));
#60911=CARTESIAN_POINT('',(269.53758689095,276.340559303206,560.336320551891));
#60912=CARTESIAN_POINT('',(269.53758689095,276.340559303206,560.336320551891));
#60913=CARTESIAN_POINT('',(269.537586890954,218.225359303206,560.336320551892));
#60914=CARTESIAN_POINT('',(269.537586890954,219.28985992302,560.336320551892));
#60915=CARTESIAN_POINT('',(269.943472391587,218.225359303206,548.713280551892));
#60916=CARTESIAN_POINT('',(270.130804161109,227.613199303206,543.348800551891));
#60917=CARTESIAN_POINT('',(269.943472391586,227.613199303206,548.713280551891));
#60918=CARTESIAN_POINT('',(270.130804161106,266.952719303206,543.348800551891));
#60919=CARTESIAN_POINT('',(270.130804161106,266.952719303206,543.348800551891));
#60920=CARTESIAN_POINT('',(270.130804161106,266.952719303206,543.348800551891));
#60921=CARTESIAN_POINT('',(269.943472391583,276.340559303206,548.713280551891));
#60922=CARTESIAN_POINT('Origin',(278.47838689095,276.340559303206,549.875584551891));
#60923=CARTESIAN_POINT('',(278.478386890949,285.281359303207,560.336320551891));
#60924=CARTESIAN_POINT('',(278.478386890949,284.875473802574,548.713280551891));
#60925=CARTESIAN_POINT('Origin',(278.47838689095,276.340559303207,560.336320551891));
#60926=CARTESIAN_POINT('Origin',(318.461644490949,284.984750668131,551.842560551891));
#60927=CARTESIAN_POINT('',(318.443762890949,285.28135930321,560.336320551891));
#60928=CARTESIAN_POINT('',(318.443762890949,285.28135930321,560.336320551891));
#60929=CARTESIAN_POINT('',(285.183147024179,285.281359303208,560.336320551891));
#60930=CARTESIAN_POINT('',(288.626194890949,284.688142033051,543.348800551891));
#60931=CARTESIAN_POINT('',(288.626194890949,284.875473802574,548.713280551891));
#60932=CARTESIAN_POINT('',(308.295954890949,284.688142033052,543.348800551891));
#60933=CARTESIAN_POINT('',(308.295954890949,284.688142033052,543.348800551891));
#60934=CARTESIAN_POINT('',(308.295954890949,284.688142033052,543.348800551891));
#60935=CARTESIAN_POINT('',(318.443762890949,284.875473802576,548.713280551891));
#60936=CARTESIAN_POINT('Origin',(318.44376289095,276.34055930321,549.875584551891));
#60937=CARTESIAN_POINT('',(327.38456289095,276.34055930321,560.336320551891));
#60938=CARTESIAN_POINT('',(326.978677390316,276.34055930321,548.713280551891));
#60939=CARTESIAN_POINT('Origin',(318.44376289095,276.34055930321,560.336320551891));
#60940=CARTESIAN_POINT('Origin',(327.087954255871,276.35844090321,551.842560551891));
#60941=CARTESIAN_POINT('',(327.384562890954,218.22535930321,560.336320551891));
#60942=CARTESIAN_POINT('',(327.384562890954,218.22535930321,560.336320551891));
#60943=CARTESIAN_POINT('',(327.38456289095,275.276058683397,560.336320551891));
#60944=CARTESIAN_POINT('',(326.791345620794,266.95271930321,543.348800551891));
#60945=CARTESIAN_POINT('',(326.978677390317,266.95271930321,548.713280551891));
#60946=CARTESIAN_POINT('',(326.791345620796,227.61319930321,543.348800551891));
#60947=CARTESIAN_POINT('',(326.791345620796,227.61319930321,543.348800551891));
#60948=CARTESIAN_POINT('',(326.978677390319,227.61319930321,548.713280551891));
#60949=CARTESIAN_POINT('',(326.791345620796,227.61319930321,543.348800551891));
#60950=CARTESIAN_POINT('',(326.97867739032,218.22535930321,548.713280551891));
#60951=CARTESIAN_POINT('',(326.978677390319,227.61319930321,548.713280551891));
#60952=CARTESIAN_POINT('',(326.97867739032,218.22535930321,548.713280551891));
#60953=CARTESIAN_POINT('Origin',(318.443762890954,218.225359303209,549.875584551891));
#60954=CARTESIAN_POINT('',(318.443762890954,209.690444803843,548.713280551891));
#60955=CARTESIAN_POINT('Origin',(318.443762890954,218.22535930321,548.713280551891));
#60956=CARTESIAN_POINT('',(318.443762890954,209.28455930321,560.336320551892));
#60957=CARTESIAN_POINT('',(318.443762890954,209.690444803843,548.713280551891));
#60958=CARTESIAN_POINT('Origin',(318.443762890954,218.22535930321,560.336320551891));
#60959=CARTESIAN_POINT('Origin',(318.461644490954,209.581167938288,551.842560551891));
#60960=CARTESIAN_POINT('',(278.478386890954,209.284559303207,560.336320551892));
#60961=CARTESIAN_POINT('',(285.183147024184,209.284559303207,560.336320551892));
#60962=CARTESIAN_POINT('',(278.478386890954,209.284559303207,560.336320551892));
#60963=CARTESIAN_POINT('',(284.851842766059,209.401953878775,556.974579751891));
#60964=CARTESIAN_POINT('Origin',(1528.1900678514,213.616412470822,436.288276072105));
#60965=CARTESIAN_POINT('',(312.070307015849,209.401953878777,556.974579751891));
#60966=CARTESIAN_POINT('',(312.070307015849,209.401953878777,556.974579751891));
#60967=CARTESIAN_POINT('',(311.739002757724,209.284559303209,560.336320551892));
#60968=CARTESIAN_POINT('Origin',(-931.267917787646,213.616412469681,436.288276099316));
#60969=CARTESIAN_POINT('',(311.739002757723,209.284559303209,560.336320551892));
#60970=CARTESIAN_POINT('',(308.295954890954,209.690444803842,548.713280551892));
#60971=CARTESIAN_POINT('',(318.443762890954,209.690444803843,548.713280551891));
#60972=CARTESIAN_POINT('',(308.295954890954,209.877776573365,543.348800551892));
#60973=CARTESIAN_POINT('',(308.295954890954,209.690444803842,548.713280551892));
#60974=CARTESIAN_POINT('',(288.626194890954,209.877776573364,543.348800551892));
#60975=CARTESIAN_POINT('',(288.626194890954,209.877776573364,543.348800551892));
#60976=CARTESIAN_POINT('',(288.626194890954,209.877776573364,543.348800551892));
#60977=CARTESIAN_POINT('',(278.478386890954,209.69044480384,548.713280551892));
#60978=CARTESIAN_POINT('Origin',(278.478386890954,218.225359303207,549.875584551892));
#60979=CARTESIAN_POINT('Origin',(278.478386890954,218.225359303207,560.336320551892));
#60980=CARTESIAN_POINT('Origin',(326.809227220795,247.28295930321,543.348800551891));
#60981=CARTESIAN_POINT('',(288.626194890954,218.672399303207,543.348800551892));
#60982=CARTESIAN_POINT('',(288.626194890954,218.672399303207,543.348800551892));
#60983=CARTESIAN_POINT('',(308.295954890954,218.672399303209,543.348800551892));
#60984=CARTESIAN_POINT('',(308.295954890954,218.672399303209,543.348800551891));
#60985=CARTESIAN_POINT('',(317.236754890953,227.613199303209,543.348800551891));
#60986=CARTESIAN_POINT('Origin',(317.236754890954,218.672399303209,543.348800551892));
#60987=CARTESIAN_POINT('',(317.236754890953,227.613199303209,543.348800551891));
#60988=CARTESIAN_POINT('',(317.23675489095,266.95271930321,543.348800551891));
#60989=CARTESIAN_POINT('',(317.23675489095,266.95271930321,543.348800551891));
#60990=CARTESIAN_POINT('',(308.29595489095,275.893519303209,543.348800551891));
#60991=CARTESIAN_POINT('Origin',(317.23675489095,275.893519303209,543.348800551891));
#60992=CARTESIAN_POINT('',(308.29595489095,275.893519303209,543.348800551891));
#60993=CARTESIAN_POINT('',(288.62619489095,275.893519303207,543.348800551891));
#60994=CARTESIAN_POINT('',(288.62619489095,275.893519303208,543.348800551891));
#60995=CARTESIAN_POINT('',(279.68539489095,266.952719303207,543.348800551891));
#60996=CARTESIAN_POINT('Origin',(279.68539489095,275.893519303207,543.348800551891));
#60997=CARTESIAN_POINT('',(279.68539489095,266.952719303207,543.348800551891));
#60998=CARTESIAN_POINT('',(279.685394890953,227.613199303207,543.348800551891));
#60999=CARTESIAN_POINT('',(279.685394890953,227.613199303207,543.348800551891));
#61000=CARTESIAN_POINT('Origin',(279.685394890954,218.672399303207,543.348800551892));
#61001=CARTESIAN_POINT('Origin',(308.295954890954,214.181422053526,543.330918951892));
#61002=CARTESIAN_POINT('',(308.295954890954,218.672399303209,548.713280551891));
#61003=CARTESIAN_POINT('',(308.295954890954,209.690444803842,548.713280551892));
#61004=CARTESIAN_POINT('',(308.295954890954,218.672399303209,548.713280551891));
#61005=CARTESIAN_POINT('Origin',(317.236754890954,218.67239930321,546.031040551891));
#61006=CARTESIAN_POINT('',(317.236754890953,227.61319930321,548.713280551891));
#61007=CARTESIAN_POINT('Origin',(317.236754890954,218.67239930321,548.713280551891));
#61008=CARTESIAN_POINT('',(317.236754890953,227.61319930321,548.713280551891));
#61009=CARTESIAN_POINT('Origin',(326.99655899032,227.61319930321,546.031040551891));
#61010=CARTESIAN_POINT('',(317.236754890953,227.61319930321,548.713280551891));
#61011=CARTESIAN_POINT('Origin',(322.107716140633,266.95271930321,543.330918951891));
#61012=CARTESIAN_POINT('',(317.23675489095,266.95271930321,548.713280551891));
#61013=CARTESIAN_POINT('Origin',(317.23675489095,275.89351930321,546.031040551891));
#61014=CARTESIAN_POINT('',(308.29595489095,275.893519303209,548.713280551891));
#61015=CARTESIAN_POINT('Origin',(308.295954890949,280.384496552892,543.330918951891));
#61016=CARTESIAN_POINT('Origin',(288.626194890949,280.384496552891,543.330918951891));
#61017=CARTESIAN_POINT('',(288.62619489095,275.893519303208,548.713280551891));
#61018=CARTESIAN_POINT('Origin',(279.68539489095,275.893519303207,546.031040551891));
#61019=CARTESIAN_POINT('',(279.68539489095,266.952719303207,548.713280551891));
#61020=CARTESIAN_POINT('Origin',(279.70327649095,266.952719303207,546.031040551891));
#61021=CARTESIAN_POINT('Origin',(274.814433641269,227.613199303207,543.330918951892));
#61022=CARTESIAN_POINT('',(279.685394890953,227.613199303207,548.713280551891));
#61023=CARTESIAN_POINT('Origin',(279.685394890954,218.672399303207,546.031040551891));
#61024=CARTESIAN_POINT('',(288.626194890954,218.672399303208,548.713280551891));
#61025=CARTESIAN_POINT('Origin',(288.626194890954,214.181422053524,543.330918951892));
#61026=CARTESIAN_POINT('Origin',(326.99655899032,218.651822053527,548.713280551891));
#61027=CARTESIAN_POINT('Origin',(298.461074890952,247.282959303208,558.655450151891));
#61028=CARTESIAN_POINT('Origin',(298.461074890952,247.28295930321,560.336320551891));
#61029=CARTESIAN_POINT('Origin',(298.461074890952,247.282959303208,556.974579751891));
#61030=CARTESIAN_POINT('Origin',(312.08818861585,206.957309168927,556.974579751891));
#61031=CARTESIAN_POINT('Origin',(245.92932859578,256.223759303205,558.101120551891));
#61032=CARTESIAN_POINT('',(243.813956261746,256.58379151797,560.336320551891));
#61033=CARTESIAN_POINT('',(245.92932859578,254.077967303205,560.336320551891));
#61034=CARTESIAN_POINT('Origin',(245.92932859578,256.223759303205,560.336320551891));
#61035=CARTESIAN_POINT('',(245.92932859578,254.077967303205,555.865920551891));
#61036=CARTESIAN_POINT('',(245.92932859578,254.077967303205,555.865920551891));
#61037=CARTESIAN_POINT('',(243.813956261746,256.58379151797,555.865920551891));
#61038=CARTESIAN_POINT('Origin',(245.92932859578,256.223759303205,555.865920551891));
#61039=CARTESIAN_POINT('',(243.813956261746,256.58379151797,555.865920551891));
#61040=CARTESIAN_POINT('Origin',(252.125930957813,254.077967303205,558.101120551891));
#61041=CARTESIAN_POINT('',(252.108049357812,254.077967303205,560.336320551891));
#61042=CARTESIAN_POINT('',(245.92932859578,254.077967303205,560.336320551891));
#61043=CARTESIAN_POINT('',(252.108049357812,254.077967303205,555.865920551891));
#61044=CARTESIAN_POINT('',(252.108049357812,254.077967303205,555.865920551891));
#61045=CARTESIAN_POINT('',(245.92932859578,254.077967303205,555.865920551891));
#61046=CARTESIAN_POINT('Origin',(252.108049357814,256.223759303204,558.101120551891));
#61047=CARTESIAN_POINT('',(254.215005063864,255.817359303205,560.336320551891));
#61048=CARTESIAN_POINT('Origin',(252.108049357813,256.223759303205,560.336320551891));
#61049=CARTESIAN_POINT('',(254.215005063864,255.817359303205,555.865920551891));
#61050=CARTESIAN_POINT('',(254.215005063864,255.817359303205,555.865920551891));
#61051=CARTESIAN_POINT('Origin',(252.108049357813,256.223759303205,555.865920551891));
#61052=CARTESIAN_POINT('Origin',(298.461074890954,247.282959303206,558.101120551891));
#61053=CARTESIAN_POINT('',(261.139646762005,272.534923205434,560.336320551891));
#61054=CARTESIAN_POINT('Origin',(298.461074890955,247.282959303206,560.336320551891));
#61055=CARTESIAN_POINT('',(261.139646762005,272.534923205434,555.865920551891));
#61056=CARTESIAN_POINT('',(261.139646762005,272.534923205434,555.865920551891));
#61057=CARTESIAN_POINT('Origin',(298.461074890955,247.282959303206,555.865920551892));
#61058=CARTESIAN_POINT('Origin',(259.362435898722,273.737397676969,558.101120551891));
#61059=CARTESIAN_POINT('',(260.879739972938,275.254701751184,560.336320551891));
#61060=CARTESIAN_POINT('Origin',(259.362435898722,273.737397676968,560.336320551891));
#61061=CARTESIAN_POINT('',(260.879739972938,275.254701751184,555.865920551891));
#61062=CARTESIAN_POINT('',(260.879739972938,275.254701751184,555.865920551891));
#61063=CARTESIAN_POINT('Origin',(259.362435898722,273.737397676968,555.865920551891));
#61064=CARTESIAN_POINT('Origin',(258.695232297992,277.43920942613,555.848038951891));
#61065=CARTESIAN_POINT('',(256.510724623046,279.623717101076,560.336320551891));
#61066=CARTESIAN_POINT('',(260.879739972938,275.254701751184,560.336320551891));
#61067=CARTESIAN_POINT('',(256.510724623046,279.623717101076,555.865920551891));
#61068=CARTESIAN_POINT('',(256.510724623046,279.623717101076,555.865920551891));
#61069=CARTESIAN_POINT('',(260.879739972938,275.254701751184,555.865920551891));
#61070=CARTESIAN_POINT('Origin',(254.993420548831,278.106413026859,558.101120551891));
#61071=CARTESIAN_POINT('',(253.243045309946,279.347626074795,560.336320551891));
#61072=CARTESIAN_POINT('Origin',(254.99342054883,278.106413026859,560.336320551891));
#61073=CARTESIAN_POINT('',(253.243045309946,279.347626074795,555.865920551891));
#61074=CARTESIAN_POINT('',(253.243045309946,279.347626074795,555.865920551891));
#61075=CARTESIAN_POINT('Origin',(254.99342054883,278.106413026859,555.865920551891));
#61076=CARTESIAN_POINT('Origin',(298.461074890961,247.282959303205,558.101120551891));
#61077=CARTESIAN_POINT('Origin',(298.46107489096,247.282959303205,560.33632055189));
#61078=CARTESIAN_POINT('Origin',(298.46107489096,247.282959303205,555.865920551891));
#61079=CARTESIAN_POINT('Origin',(262.15022814681,267.203234441337,555.865920551891));
#61080=CARTESIAN_POINT('Origin',(268.304824768025,287.048801896164,555.848038951891));
#61081=CARTESIAN_POINT('',(266.120317093079,289.23330957111,560.336320551891));
#61082=CARTESIAN_POINT('',(270.48933244297,284.864294221219,560.336320551891));
#61083=CARTESIAN_POINT('',(266.120317093079,289.23330957111,560.336320551891));
#61084=CARTESIAN_POINT('',(270.48933244297,284.864294221219,555.865920551891));
#61085=CARTESIAN_POINT('',(270.48933244297,284.864294221219,555.865920551891));
#61086=CARTESIAN_POINT('',(266.120317093079,289.23330957111,555.865920551891));
#61087=CARTESIAN_POINT('',(266.120317093079,289.23330957111,555.865920551891));
#61088=CARTESIAN_POINT('',(266.120317093079,289.23330957111,555.865920551891));
#61089=CARTESIAN_POINT('Origin',(272.006636517186,286.381598295435,558.101120551891));
#61090=CARTESIAN_POINT('',(273.209110988721,284.604387432152,560.336320551891));
#61091=CARTESIAN_POINT('Origin',(272.006636517186,286.381598295436,560.336320551891));
#61092=CARTESIAN_POINT('',(273.209110988721,284.604387432152,555.865920551891));
#61093=CARTESIAN_POINT('',(273.209110988721,284.604387432152,555.865920551891));
#61094=CARTESIAN_POINT('Origin',(272.006636517186,286.381598295436,555.865920551891));
#61095=CARTESIAN_POINT('Origin',(298.461074890949,247.282959303215,558.101120551891));
#61096=CARTESIAN_POINT('',(291.206834890949,291.75684692871,560.336320551891));
#61097=CARTESIAN_POINT('Origin',(298.461074890951,247.282959303211,560.336320551892));
#61098=CARTESIAN_POINT('',(291.206834890949,291.75684692871,555.865920551891));
#61099=CARTESIAN_POINT('',(291.206834890949,291.75684692871,555.865920551891));
#61100=CARTESIAN_POINT('Origin',(298.461074890951,247.282959303211,555.865920551891));
#61101=CARTESIAN_POINT('Origin',(290.861394890949,293.874651101353,558.101120551891));
#61102=CARTESIAN_POINT('',(293.007186890949,293.874651101353,560.336320551891));
#61103=CARTESIAN_POINT('Origin',(290.861394890949,293.874651101353,560.336320551891));
#61104=CARTESIAN_POINT('',(293.007186890949,293.874651101353,555.865920551891));
#61105=CARTESIAN_POINT('',(293.007186890949,293.874651101353,555.865920551891));
#61106=CARTESIAN_POINT('Origin',(290.861394890949,293.874651101353,555.865920551891));
#61107=CARTESIAN_POINT('Origin',(293.007186890948,296.950035441681,555.848038951891));
#61108=CARTESIAN_POINT('',(293.007186890948,300.025419782008,560.336320551891));
#61109=CARTESIAN_POINT('',(293.007186890949,293.874651101353,560.336320551891));
#61110=CARTESIAN_POINT('',(293.007186890948,300.025419782008,555.865920551891));
#61111=CARTESIAN_POINT('',(293.007186890948,300.025419782008,555.865920551891));
#61112=CARTESIAN_POINT('',(293.007186890949,293.874651101353,555.865920551891));
#61113=CARTESIAN_POINT('Origin',(290.861394890948,300.025419782008,558.101120551891));
#61114=CARTESIAN_POINT('',(290.555367685928,302.149277276534,560.336320551891));
#61115=CARTESIAN_POINT('Origin',(290.861394890948,300.025419782008,560.336320551891));
#61116=CARTESIAN_POINT('',(290.555367685928,302.149277276534,555.865920551891));
#61117=CARTESIAN_POINT('',(290.555367685928,302.149277276534,555.865920551891));
#61118=CARTESIAN_POINT('Origin',(290.861394890948,300.025419782008,555.865920551891));
#61119=CARTESIAN_POINT('Origin',(298.461074890954,247.282959303205,558.101120551891));
#61120=CARTESIAN_POINT('',(266.396408265671,292.500988987961,560.336320551891));
#61121=CARTESIAN_POINT('Origin',(298.461074890952,247.282959303207,560.336320551891));
#61122=CARTESIAN_POINT('',(266.396408265671,292.500988987961,555.865920551891));
#61123=CARTESIAN_POINT('',(266.396408265671,292.500988987961,555.865920551891));
#61124=CARTESIAN_POINT('Origin',(298.461074890952,247.282959303207,555.865920551891));
#61125=CARTESIAN_POINT('Origin',(267.637621167297,290.750613645327,558.101120551891));
#61126=CARTESIAN_POINT('Origin',(267.637621167294,290.750613645326,560.336320551891));
#61127=CARTESIAN_POINT('Origin',(267.637621167294,290.750613645326,555.865920551891));
#61128=CARTESIAN_POINT('Origin',(293.025068490949,292.95037556378,555.865920551891));
#61129=CARTESIAN_POINT('Origin',(298.461074890946,247.282959303207,558.101120551891));
#61130=CARTESIAN_POINT('',(243.813956261747,237.98212708844,560.336320551892));
#61131=CARTESIAN_POINT('',(253.243045206199,215.218292677928,560.336320551892));
#61132=CARTESIAN_POINT('Origin',(298.461074890947,247.282959303207,560.336320551892));
#61133=CARTESIAN_POINT('',(253.243045206199,215.218292677928,555.865920551892));
#61134=CARTESIAN_POINT('',(253.243045206199,215.218292677928,555.865920551892));
#61135=CARTESIAN_POINT('',(243.813956261747,237.982127088439,555.865920551891));
#61136=CARTESIAN_POINT('Origin',(298.461074890947,247.282959303207,555.865920551892));
#61137=CARTESIAN_POINT('',(243.813956261747,237.982127088439,555.865920551891));
#61138=CARTESIAN_POINT('Origin',(254.993420548834,216.459505579551,558.101120551892));
#61139=CARTESIAN_POINT('',(256.51072462305,214.942201505336,560.336320551892));
#61140=CARTESIAN_POINT('Origin',(254.993420548834,216.459505579551,560.336320551892));
#61141=CARTESIAN_POINT('',(256.51072462305,214.942201505335,555.865920551892));
#61142=CARTESIAN_POINT('',(256.51072462305,214.942201505335,555.865920551892));
#61143=CARTESIAN_POINT('Origin',(254.993420548834,216.459505579551,555.865920551892));
#61144=CARTESIAN_POINT('Origin',(258.695232297996,217.126709180281,555.848038951892));
#61145=CARTESIAN_POINT('',(260.879739972942,219.311216855227,560.336320551892));
#61146=CARTESIAN_POINT('',(256.51072462305,214.942201505336,560.336320551892));
#61147=CARTESIAN_POINT('',(260.879739972942,219.311216855227,555.865920551891));
#61148=CARTESIAN_POINT('',(260.879739972942,219.311216855227,555.865920551891));
#61149=CARTESIAN_POINT('',(256.51072462305,214.942201505335,555.865920551892));
#61150=CARTESIAN_POINT('Origin',(259.362435898725,220.828520929443,558.101120551892));
#61151=CARTESIAN_POINT('',(261.139646762008,222.030995400978,560.336320551892));
#61152=CARTESIAN_POINT('Origin',(259.362435898726,220.828520929443,560.336320551892));
#61153=CARTESIAN_POINT('',(261.139646762008,222.030995400978,555.865920551891));
#61154=CARTESIAN_POINT('',(261.139646762008,222.030995400978,555.865920551891));
#61155=CARTESIAN_POINT('Origin',(259.362435898726,220.828520929443,555.865920551891));
#61156=CARTESIAN_POINT('Origin',(298.461074890954,247.28295930321,558.101120551891));
#61157=CARTESIAN_POINT('',(254.215005063865,238.748559303205,560.336320551891));
#61158=CARTESIAN_POINT('Origin',(298.461074890955,247.282959303211,560.336320551891));
#61159=CARTESIAN_POINT('',(254.215005063865,238.748559303205,555.865920551891));
#61160=CARTESIAN_POINT('',(254.215005063865,238.748559303205,555.865920551891));
#61161=CARTESIAN_POINT('Origin',(298.461074890955,247.282959303211,555.86592055189));
#61162=CARTESIAN_POINT('Origin',(252.108049357813,238.342159303204,558.101120551891));
#61163=CARTESIAN_POINT('',(252.108049357813,240.487951303205,560.336320551891));
#61164=CARTESIAN_POINT('Origin',(252.108049357814,238.342159303206,560.336320551891));
#61165=CARTESIAN_POINT('',(252.108049357813,240.487951303205,555.865920551891));
#61166=CARTESIAN_POINT('',(252.108049357813,240.487951303205,555.865920551891));
#61167=CARTESIAN_POINT('Origin',(252.108049357814,238.342159303206,555.865920551891));
#61168=CARTESIAN_POINT('Origin',(252.125930957813,240.487951303205,558.101120551891));
#61169=CARTESIAN_POINT('',(245.929328595781,240.487951303205,560.336320551891));
#61170=CARTESIAN_POINT('',(252.108049357813,240.487951303205,560.336320551891));
#61171=CARTESIAN_POINT('',(245.929328595781,240.487951303205,555.865920551891));
#61172=CARTESIAN_POINT('',(245.929328595781,240.487951303205,555.865920551891));
#61173=CARTESIAN_POINT('',(252.108049357813,240.487951303205,555.865920551891));
#61174=CARTESIAN_POINT('Origin',(245.929328595778,238.342159303205,558.101120551891));
#61175=CARTESIAN_POINT('Origin',(245.929328595781,238.342159303205,560.336320551892));
#61176=CARTESIAN_POINT('Origin',(245.929328595781,238.342159303205,555.865920551891));
#61177=CARTESIAN_POINT('Origin',(262.150228146813,227.362684145801,555.865920551891));
#61178=CARTESIAN_POINT('Origin',(298.461074890952,247.282959303211,558.101120551891));
#61179=CARTESIAN_POINT('',(266.396408265677,202.064929618451,560.336320551892));
#61180=CARTESIAN_POINT('',(290.555367508405,192.416641355462,560.336320551892));
#61181=CARTESIAN_POINT('Origin',(298.461074890951,247.282959303207,560.33632055189));
#61182=CARTESIAN_POINT('',(290.555367508405,192.416641355462,555.865920551892));
#61183=CARTESIAN_POINT('',(290.555367508405,192.416641355462,555.865920551892));
#61184=CARTESIAN_POINT('',(266.396408265677,202.064929618451,555.865920551892));
#61185=CARTESIAN_POINT('Origin',(298.461074890951,247.282959303206,555.86592055189));
#61186=CARTESIAN_POINT('',(266.396408265677,202.064929618451,555.865920551892));
#61187=CARTESIAN_POINT('Origin',(290.861394890955,194.540498824408,558.101120551892));
#61188=CARTESIAN_POINT('',(293.007186890955,194.540498824408,560.336320551892));
#61189=CARTESIAN_POINT('Origin',(290.861394890955,194.540498824408,560.336320551892));
#61190=CARTESIAN_POINT('',(293.007186890955,194.540498824408,555.865920551892));
#61191=CARTESIAN_POINT('',(293.007186890955,194.540498824408,555.865920551892));
#61192=CARTESIAN_POINT('Origin',(290.861394890955,194.540498824408,555.865920551892));
#61193=CARTESIAN_POINT('Origin',(293.007186890955,197.615883164735,555.848038951892));
#61194=CARTESIAN_POINT('',(293.007186890955,200.691267505062,560.336320551892));
#61195=CARTESIAN_POINT('',(293.007186890955,194.540498824408,560.336320551892));
#61196=CARTESIAN_POINT('',(293.007186890955,200.691267505062,555.865920551892));
#61197=CARTESIAN_POINT('',(293.007186890955,200.691267505062,555.865920551892));
#61198=CARTESIAN_POINT('',(293.007186890955,194.540498824408,555.865920551892));
#61199=CARTESIAN_POINT('Origin',(290.861394890955,200.691267505062,558.101120551892));
#61200=CARTESIAN_POINT('',(291.206834656197,202.809071715997,560.336320551892));
#61201=CARTESIAN_POINT('Origin',(290.861394890955,200.691267505062,560.336320551892));
#61202=CARTESIAN_POINT('',(291.206834656197,202.809071715997,555.865920551892));
#61203=CARTESIAN_POINT('',(291.206834656197,202.809071715997,555.865920551892));
#61204=CARTESIAN_POINT('Origin',(290.861394890955,200.691267505062,555.865920551892));
#61205=CARTESIAN_POINT('Origin',(298.461074890951,247.282959303207,558.101120551891));
#61206=CARTESIAN_POINT('',(273.209110224242,209.961531691517,560.336320551892));
#61207=CARTESIAN_POINT('Origin',(298.461074890951,247.282959303207,560.336320551891));
#61208=CARTESIAN_POINT('',(273.209110224242,209.961531691517,555.865920551892));
#61209=CARTESIAN_POINT('',(273.209110224242,209.961531691517,555.865920551892));
#61210=CARTESIAN_POINT('Origin',(298.46107489095,247.282959303205,555.865920551891));
#61211=CARTESIAN_POINT('Origin',(272.006636517191,208.184320310979,558.101120551892));
#61212=CARTESIAN_POINT('',(270.489332442976,209.701624385194,560.336320551892));
#61213=CARTESIAN_POINT('Origin',(272.006636517192,208.184320310979,560.336320551892));
#61214=CARTESIAN_POINT('',(270.489332442976,209.701624385194,555.865920551892));
#61215=CARTESIAN_POINT('',(270.489332442976,209.701624385194,555.865920551892));
#61216=CARTESIAN_POINT('Origin',(272.006636517192,208.184320310979,555.865920551892));
#61217=CARTESIAN_POINT('Origin',(268.30482476803,207.517116710248,555.848038951892));
#61218=CARTESIAN_POINT('',(266.120317093085,205.332609035303,560.336320551892));
#61219=CARTESIAN_POINT('',(270.489332442976,209.701624385194,560.336320551892));
#61220=CARTESIAN_POINT('',(266.120317093085,205.332609035303,555.865920551892));
#61221=CARTESIAN_POINT('',(266.120317093085,205.332609035303,555.865920551892));
#61222=CARTESIAN_POINT('',(270.489332442976,209.701624385194,555.865920551892));
#61223=CARTESIAN_POINT('Origin',(267.637621167301,203.815304961088,558.101120551892));
#61224=CARTESIAN_POINT('Origin',(267.6376211673,203.815304961087,560.336320551892));
#61225=CARTESIAN_POINT('Origin',(267.6376211673,203.815304961087,555.865920551892));
#61226=CARTESIAN_POINT('Origin',(293.025068490955,201.615542736639,555.865920551892));
#61227=CARTESIAN_POINT('Origin',(298.461074890952,247.28295930321,558.101120551891));
#61228=CARTESIAN_POINT('',(323.713038793177,284.604387432155,560.336320551891));
#61229=CARTESIAN_POINT('',(305.715314890949,291.756846928711,560.336320551891));
#61230=CARTESIAN_POINT('Origin',(298.461074890952,247.282959303207,560.336320551891));
#61231=CARTESIAN_POINT('',(323.713038793177,284.604387432155,555.865920551891));
#61232=CARTESIAN_POINT('',(305.715314890949,291.756846928711,555.865920551891));
#61233=CARTESIAN_POINT('Origin',(306.060754890949,293.874651101355,558.101120551891));
#61234=CARTESIAN_POINT('',(303.914962890949,293.874651101354,560.336320551891));
#61235=CARTESIAN_POINT('Origin',(306.060754890949,293.874651101354,560.336320551891));
#61236=CARTESIAN_POINT('',(303.914962890949,293.874651101354,555.865920551891));
#61237=CARTESIAN_POINT('Origin',(303.914962890948,296.950035441682,555.848038951891));
#61238=CARTESIAN_POINT('',(303.914962890948,300.025419782009,560.336320551891));
#61239=CARTESIAN_POINT('',(303.914962890948,300.025419782009,560.336320551891));
#61240=CARTESIAN_POINT('',(303.914962890948,300.025419782009,555.865920551891));
#61241=CARTESIAN_POINT('Origin',(306.060754890948,300.025419782009,558.101120551891));
#61242=CARTESIAN_POINT('',(306.366782273498,302.149277250954,560.336320551891));
#61243=CARTESIAN_POINT('Origin',(306.060754890948,300.025419782009,560.336320551891));
#61244=CARTESIAN_POINT('',(306.366782273498,302.149277250954,555.865920551891));
#61245=CARTESIAN_POINT('Origin',(298.461074890952,247.282959303207,558.101120551891));
#61246=CARTESIAN_POINT('',(330.525741198797,292.500989213059,560.336320551891));
#61247=CARTESIAN_POINT('Origin',(298.461074890953,247.282959303211,560.336320551892));
#61248=CARTESIAN_POINT('',(330.525741198797,292.500989213059,555.865920551891));
#61249=CARTESIAN_POINT('Origin',(329.284528614603,290.75061364533,558.101120551891));
#61250=CARTESIAN_POINT('',(330.801832688819,289.233309571114,560.336320551891));
#61251=CARTESIAN_POINT('Origin',(329.284528614603,290.75061364533,560.336320551891));
#61252=CARTESIAN_POINT('',(330.801832688819,289.233309571114,555.865920551891));
#61253=CARTESIAN_POINT('Origin',(324.915513264711,286.381598295438,558.101120551891));
#61254=CARTESIAN_POINT('',(326.432817338928,284.864294221223,560.336320551891));
#61255=CARTESIAN_POINT('Origin',(324.915513264712,286.381598295438,560.336320551891));
#61256=CARTESIAN_POINT('',(326.432817338928,284.864294221222,555.865920551891));
#61257=CARTESIAN_POINT('Origin',(328.617325013873,287.048801896168,555.848038951891));
#61258=CARTESIAN_POINT('',(326.432817338928,284.864294221223,560.336320551891));
#61259=CARTESIAN_POINT('Origin',(298.461074890952,247.282959303208,554.971840551891));
#61260=CARTESIAN_POINT('',(298.461074890956,191.04982903683,553.183680551892));
#61261=CARTESIAN_POINT('Origin',(298.461074890956,191.049829036829,554.971840551892));
#61262=CARTESIAN_POINT('Origin',(298.461074890952,247.282959303208,553.183680551891));
#61263=CARTESIAN_POINT('Origin',(354.71208675733,247.282959303212,553.183680551891));
#61264=CARTESIAN_POINT('',(266.668723505555,279.319128262139,553.183680551891));
#61265=CARTESIAN_POINT('',(266.668723505559,215.246790344273,553.183680551891));
#61266=CARTESIAN_POINT('',(266.668723505555,279.319128262139,553.183680551891));
#61267=CARTESIAN_POINT('',(275.902153932022,206.013359917812,553.183680551892));
#61268=CARTESIAN_POINT('',(266.668723505559,215.246790344273,553.183680551891));
#61269=CARTESIAN_POINT('',(321.019995849888,206.013359917815,553.183680551891));
#61270=CARTESIAN_POINT('',(275.902153932022,206.013359917812,553.183680551892));
#61271=CARTESIAN_POINT('',(330.253426276349,215.246790344278,553.183680551891));
#61272=CARTESIAN_POINT('',(321.019995849888,206.013359917815,553.183680551891));
#61273=CARTESIAN_POINT('',(330.253426276344,279.319128262143,553.183680551891));
#61274=CARTESIAN_POINT('',(330.253426276349,215.246790344278,553.183680551891));
#61275=CARTESIAN_POINT('',(321.019995849882,288.552558688605,553.183680551891));
#61276=CARTESIAN_POINT('',(330.253426276344,279.319128262143,553.183680551891));
#61277=CARTESIAN_POINT('',(275.902153932016,288.552558688602,553.183680551891));
#61278=CARTESIAN_POINT('',(321.019995849882,288.552558688605,553.183680551891));
#61279=CARTESIAN_POINT('',(275.902153932016,288.552558688602,553.183680551891));
#61280=CARTESIAN_POINT('Origin',(271.558236896863,283.663045297292,542.135960560502));
#61281=CARTESIAN_POINT('',(266.668723505555,279.319128262139,553.183680551891));
#61282=CARTESIAN_POINT('',(275.902153932016,288.552558688602,553.183680551891));
#61283=CARTESIAN_POINT('Origin',(325.363912885035,283.663045297296,542.135960560501));
#61284=CARTESIAN_POINT('',(321.019995849882,288.552558688605,553.183680551891));
#61285=CARTESIAN_POINT('',(330.253426276344,279.319128262143,553.183680551891));
#61286=CARTESIAN_POINT('Origin',(321.037877449882,288.302782995907,546.031040551891));
#61287=CARTESIAN_POINT('Origin',(321.037877449888,206.263135610512,546.031040551891));
#61288=CARTESIAN_POINT('',(321.019995849888,206.013359917815,553.183680551891));
#61289=CARTESIAN_POINT('',(275.902153932022,206.013359917812,553.183680551892));
#61290=CARTESIAN_POINT('Origin',(271.558236896869,210.902873309121,542.135960560502));
#61291=CARTESIAN_POINT('',(266.668723505559,215.246790344273,553.183680551891));
#61292=CARTESIAN_POINT('Origin',(356.594156490952,247.282959303212,560.336320551891));
#61293=CARTESIAN_POINT('Origin',(330.003650583647,279.337009862143,546.031040551891));
#61294=CARTESIAN_POINT('',(330.253426276349,215.246790344278,553.183680551891));
#61295=CARTESIAN_POINT('Origin',(266.918499198253,279.337009862139,546.031040551891));
#61296=CARTESIAN_POINT('Origin',(325.36391288504,210.902873309124,542.135960560502));
#61297=CARTESIAN_POINT('Origin',(327.864997019629,247.28295930321,538.878400551891));
#61298=CARTESIAN_POINT('Origin',(319.69547489095,274.10535930321,552.727699751891));
#61299=CARTESIAN_POINT('',(319.69547489095,279.13008890321,552.682995751891));
#61300=CARTESIAN_POINT('',(322.615388379292,278.194615075807,552.682995751891));
#61301=CARTESIAN_POINT('Origin',(319.69547489095,274.10535930321,552.682995751891));
#61302=CARTESIAN_POINT('Origin',(319.69547489095,274.10535930321,552.682995751891));
#61303=CARTESIAN_POINT('',(322.35560959919,277.830802284651,553.130035751891));
#61304=CARTESIAN_POINT('',(322.589410501282,278.158233796692,552.727699751891));
#61305=CARTESIAN_POINT('Origin',(319.69547489095,274.10535930321,553.130035751891));
#61306=CARTESIAN_POINT('Origin',(319.69547489095,274.10535930321,550.754018151891));
#61307=CARTESIAN_POINT('',(319.69547489095,279.13008890321,548.825040551891));
#61308=CARTESIAN_POINT('',(319.69547489095,279.13008890321,550.754018151891));
#61309=CARTESIAN_POINT('',(322.615388379293,270.016103530613,548.825040551891));
#61310=CARTESIAN_POINT('Origin',(319.69547489095,274.10535930321,548.825040551891));
#61311=CARTESIAN_POINT('Origin',(319.69547489095,274.10535930321,548.825040551891));
#61312=CARTESIAN_POINT('Origin',(319.69547489095,274.10535930321,548.813864551891));
#61313=CARTESIAN_POINT('',(322.60889390979,270.025198850392,548.813864551891));
#61314=CARTESIAN_POINT('Origin',(316.89700449095,274.10535930321,553.147917351891));
#61315=CARTESIAN_POINT('',(316.89700449095,275.721056941969,553.130035751891));
#61316=CARTESIAN_POINT('',(316.89700449095,272.489661664451,553.130035751891));
#61317=CARTESIAN_POINT('',(316.89700449095,275.721056941969,553.130035751891));
#61318=CARTESIAN_POINT('',(316.89700449095,272.48966166445,550.984243751891));
#61319=CARTESIAN_POINT('',(316.89700449095,272.48966166445,550.984243751891));
#61320=CARTESIAN_POINT('',(316.89700449095,275.721056941969,550.984243751891));
#61321=CARTESIAN_POINT('',(316.89700449095,275.721056941969,550.984243751891));
#61322=CARTESIAN_POINT('',(316.89700449095,275.721056941969,550.984243751891));
#61323=CARTESIAN_POINT('Origin',(318.29623969095,271.681812845071,553.147917351891));
#61324=CARTESIAN_POINT('',(319.69547489095,270.873964025691,553.130035751891));
#61325=CARTESIAN_POINT('',(316.89700449095,272.489661664451,553.130035751891));
#61326=CARTESIAN_POINT('',(319.69547489095,270.873964025691,550.984243751891));
#61327=CARTESIAN_POINT('',(319.69547489095,270.873964025691,550.984243751891));
#61328=CARTESIAN_POINT('',(316.89700449095,272.48966166445,550.984243751891));
#61329=CARTESIAN_POINT('Origin',(321.09471009095,271.681812845071,553.147917351891));
#61330=CARTESIAN_POINT('',(322.49394529095,272.489661664451,553.130035751891));
#61331=CARTESIAN_POINT('',(319.69547489095,270.873964025691,553.130035751891));
#61332=CARTESIAN_POINT('',(322.49394529095,272.489661664451,550.984243751891));
#61333=CARTESIAN_POINT('',(322.49394529095,272.489661664451,550.984243751891));
#61334=CARTESIAN_POINT('',(319.69547489095,270.873964025691,550.984243751891));
#61335=CARTESIAN_POINT('Origin',(322.49394529095,274.10535930321,553.147917351891));
#61336=CARTESIAN_POINT('',(322.49394529095,275.721056941969,553.130035751891));
#61337=CARTESIAN_POINT('',(322.49394529095,275.721056941969,553.130035751891));
#61338=CARTESIAN_POINT('',(322.49394529095,275.721056941969,550.984243751891));
#61339=CARTESIAN_POINT('',(322.49394529095,275.721056941969,550.984243751891));
#61340=CARTESIAN_POINT('',(322.49394529095,272.489661664451,550.984243751891));
#61341=CARTESIAN_POINT('Origin',(321.09471009095,276.528905761349,553.147917351891));
#61342=CARTESIAN_POINT('',(319.69547489095,277.336754580728,553.130035751891));
#61343=CARTESIAN_POINT('',(322.49394529095,275.721056941969,553.130035751891));
#61344=CARTESIAN_POINT('',(319.69547489095,277.336754580728,550.984243751891));
#61345=CARTESIAN_POINT('',(319.69547489095,277.336754580728,550.984243751891));
#61346=CARTESIAN_POINT('',(322.49394529095,275.721056941969,550.984243751891));
#61347=CARTESIAN_POINT('Origin',(316.87912289095,274.10535930321,550.984243751891));
#61348=CARTESIAN_POINT('',(319.69547489095,277.336754580728,550.984243751891));
#61349=CARTESIAN_POINT('Origin',(318.29623969095,276.528905761349,553.147917351891));
#61350=CARTESIAN_POINT('',(319.69547489095,277.336754580728,553.130035751891));
#61351=CARTESIAN_POINT('Origin',(315.09990369095,274.10535930321,553.130035751891));
#61778=UNCERTAINTY_MEASURE_WITH_UNIT(LENGTH_MEASURE(0.01),#61812,
'DISTANCE_ACCURACY_VALUE',
'Maximum model space distance between geometric entities at asserted c
onnectivities');
#61780=UNCERTAINTY_MEASURE_WITH_UNIT(LENGTH_MEASURE(0.01),#61812,
'DISTANCE_ACCURACY_VALUE',
'Maximum model space distance between geometric entities at asserted c
onnectivities');
#61809=(
GEOMETRIC_REPRESENTATION_CONTEXT(3)
GLOBAL_UNCERTAINTY_ASSIGNED_CONTEXT((#61778))
GLOBAL_UNIT_ASSIGNED_CONTEXT((#61812,#61814,#61815))
REPRESENTATION_CONTEXT('','3D')
);
#61811=(
GEOMETRIC_REPRESENTATION_CONTEXT(3)
GLOBAL_UNCERTAINTY_ASSIGNED_CONTEXT((#61780))
GLOBAL_UNIT_ASSIGNED_CONTEXT((#61812,#61814,#61815))
REPRESENTATION_CONTEXT('','3D')
);
#61812=(
LENGTH_UNIT()
NAMED_UNIT(*)
SI_UNIT(.MILLI.,.METRE.)
);
#61814=(
NAMED_UNIT(*)
PLANE_ANGLE_UNIT()
SI_UNIT($,.RADIAN.)
);
#61815=(
NAMED_UNIT(*)
SI_UNIT($,.STERADIAN.)
SOLID_ANGLE_UNIT()
);
#61844=SHAPE_DEFINITION_REPRESENTATION(#61908,#61996);
#61908=PRODUCT_DEFINITION_SHAPE('',$,#62027);
#61996=SHAPE_REPRESENTATION('',(#37247),#61809);
#61998=PRODUCT_DEFINITION_CONTEXT('part definition',#62090,'design');
#62027=PRODUCT_DEFINITION('Gearbox Reducer','Gearbox Reducer',#62057,#61998);
#62057=PRODUCT_DEFINITION_FORMATION('',$,#62120);
#62090=APPLICATION_CONTEXT('Managed model based 3d engineering');
#62091=PRODUCT_CONTEXT('part definition',#62090,'mechanical');
#62120=PRODUCT('Gearbox Reducer','Gearbox Reducer',$,(#62091));
#62164=COLOUR_RGB('Off White',0.89,0.88,0.83);
#62165=FILL_AREA_STYLE_COLOUR('',#62164);
#62166=FILL_AREA_STYLE('',(#62165));
#62167=SURFACE_STYLE_FILL_AREA(#62166);
#62168=SURFACE_SIDE_STYLE('',(#62167));
#62169=SURFACE_STYLE_USAGE(.BOTH.,#62168);
#62170=PRESENTATION_STYLE_ASSIGNMENT((#62169));
ENDSEC;
END-ISO-10303-21;
